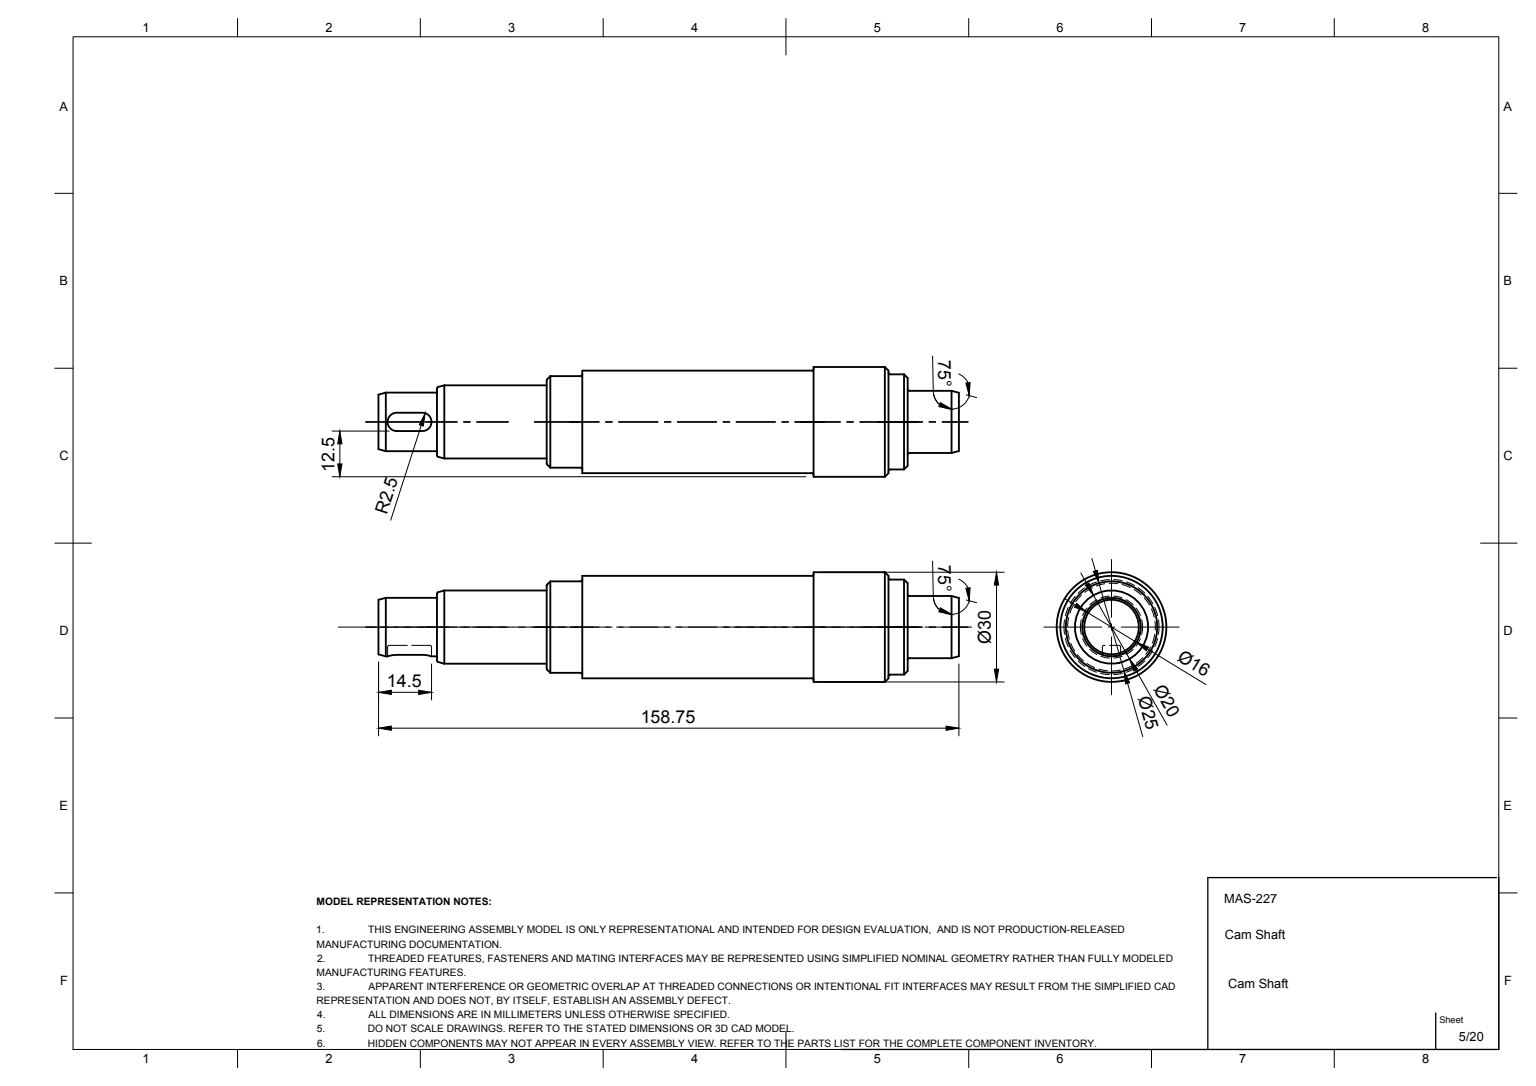
ISO-10303-21;
HEADER;
FILE_DESCRIPTION (('STEP AP214'),
    '1' );
FILE_NAME ( 'Cam Shaft.step', '2026-10-06T08:24:41', ( '' ), ( '' ), 'STEP AP214', 'Unspecified', '' );
FILE_SCHEMA (( 'AUTOMOTIVE_DESIGN' ));
ENDSEC;
DATA;
#1=ORIENTED_EDGE ( 'NONE', *, *, #7056, .T. ) ;
#8=CARTESIAN_POINT ( 'NONE',  ( 0.4441657790107835790, 0.2564944395515610931, 1.766732283464566899 ) ) ;
#9=CARTESIAN_POINT ( 'NONE',  ( -0.4441657790107816917, 0.2564944395515652564, 1.747047244094488194 ) ) ;
#12=ORIENTED_EDGE ( 'NONE', *, *, #1724, .F. ) ;
#14=CARTESIAN_POINT ( 'NONE',  ( 0.3392387706403788838, 0.1151913129404419922, -3.115157480314960647 ) ) ;
#21=CARTESIAN_POINT ( 'NONE',  ( 0.3324885138898234782, -0.04380447413659139394, 1.973425196850393970 ) ) ;
#25=VERTEX_POINT ( 'NONE', #21962 ) ;
#35=LINE ( 'NONE', #6897, #10289 ) ;
#46=CARTESIAN_POINT ( 'NONE',  ( -0.08600259748440698682, 0.2165354330708661457, -3.223068998490977499 ) ) ;
#47=ORIENTED_EDGE ( 'NONE', *, *, #24932, .T. ) ;
#49=DIRECTION ( 'NONE',  ( 0.000000000000000000, 0.000000000000000000, 1.000000000000000000 ) ) ;
#56=CARTESIAN_POINT ( 'NONE',  ( -0.5476281405333500718, 0.07214854559197644845, 0.9399606299212598381 ) ) ;
#59=ORIENTED_EDGE ( 'NONE', *, *, #13176, .F. ) ;
#74=CARTESIAN_POINT ( 'NONE',  ( 0.1480156394741928561, -0.5526079293736928522, 0.9399606299212598381 ) ) ;
#77=CARTESIAN_POINT ( 'NONE',  ( 0.04673558830902516809, 0.3552036222399216903, -3.115157480314960647 ) ) ;
#82=CARTESIAN_POINT ( 'NONE',  ( 0.4856708409191422549, -0.1649135259639211148, -1.550196850393700920 ) ) ;
#84=CARTESIAN_POINT ( 'NONE',  ( 0.5144793533649091311, -0.1379038425970198489, 1.747047244094488416 ) ) ;
#88=VERTEX_POINT ( 'NONE', #13082 ) ;
#90=CIRCLE ( 'NONE', #23529, 0.3937007874015748254 ) ;
#99=CARTESIAN_POINT ( 'NONE',  ( -0.3001918266901933974, 0.3912931228432126596, -1.550196850393700920 ) ) ;
#101=CARTESIAN_POINT ( 'NONE',  ( 0.1458850421962362143, -0.4296318976989931815, -1.934055118110236338 ) ) ;
#106=DIRECTION ( 'NONE',  ( -1.000000000000000000, 0.000000000000000000, -0.000000000000000000 ) ) ;
#113=CARTESIAN_POINT ( 'NONE',  ( -0.3350125228558759050, 0.2937477835494528011, -1.934055118110236560 ) ) ;
#118=CARTESIAN_POINT ( 'NONE',  ( -0.1839420097223181394, -0.5417097841048805762, 0.9399606299212598381 ) ) ;
#123=CARTESIAN_POINT ( 'NONE',  ( 0.3858827008519146728, -0.2227458012931471110, -1.934055118110236338 ) ) ;
#124=CARTESIAN_POINT ( 'NONE',  ( 0.3233561589689052385, -0.1867299569291582528, -3.115157480314960647 ) ) ;
#138=CARTESIAN_POINT ( 'NONE',  ( -0.4069448477556107946, -0.3121994997598286914, 1.766732283464566899 ) ) ;
#144=CARTESIAN_POINT ( 'NONE',  ( 0.3460635936745020680, -0.09269288654273737105, -3.115157480314960647 ) ) ;
#157=ORIENTED_EDGE ( 'NONE', *, *, #9364, .T. ) ;
#162=CARTESIAN_POINT ( 'NONE',  ( 0.09842519685039370636, 0.2165354330708661457, -3.456364829396325167 ) ) ;
#174=CARTESIAN_POINT ( 'NONE',  ( -0.07870736599817811097, 0.1968503937007873850, -3.212150913008701814 ) ) ;
#175=EDGE_LOOP ( 'NONE', ( #22367, #5338, #24383, #19393 ) ) ;
#188=CARTESIAN_POINT ( 'NONE',  ( -0.4382482975805212511, 0.3362148458989001609, 0.9399606299212598381 ) ) ;
#205=CARTESIAN_POINT ( 'NONE',  ( 0.07472527936312040042, -0.5671862884095228985, 0.9399606299212598381 ) ) ;
#215=CARTESIAN_POINT ( 'NONE',  ( 0.4954757973265890847, -0.2860025288253325582, 0.9399606299212601712 ) ) ;
#255=CARTESIAN_POINT ( 'NONE',  ( -0.03736310157557653361, -0.5708661417322835607, 0.9399606299212598381 ) ) ;
#258=CARTESIAN_POINT ( 'NONE',  ( 0.4303681241740789920, -0.1153557615287144622, -1.934055118110236338 ) ) ;
#259=CARTESIAN_POINT ( 'NONE',  ( -0.3233561589689049609, -0.1867299569291588357, -3.115157480314960647 ) ) ;
#271=CARTESIAN_POINT ( 'NONE',  ( 0.5118110236220472231, 0.03349795313260757468, 1.766732283464566899 ) ) ;
#277=CARTESIAN_POINT ( 'NONE',  ( 0.2362439534887500470, 0.2693339498142248156, -3.115157480314960647 ) ) ;
#283=CARTESIAN_POINT ( 'NONE',  ( 0.2521176338356670432, 0.2211428102655656758, 1.953740157480315043 ) ) ;
#285=VERTEX_POINT ( 'NONE', #25460 ) ;
#301=ORIENTED_EDGE ( 'NONE', *, *, #18506, .T. ) ;
#306=CARTESIAN_POINT ( 'NONE',  ( 0.07870736599818350943, 0.1968503937007873850, -3.212150913008773312 ) ) ;
#310=CARTESIAN_POINT ( 'NONE',  ( 0.3362554559023149814, -0.1141145734059788724, 1.953740157480315043 ) ) ;
#314=PLANE ( 'NONE',  #8850 ) ;
#317=CARTESIAN_POINT ( 'NONE',  ( 0.4783323773986625782, 0.2762247810518427271, 0.9399606299212598381 ) ) ;
#319=DIRECTION ( 'NONE',  ( 1.000000000000000000, 0.000000000000000000, 0.000000000000000000 ) ) ;
#324=AXIS2_PLACEMENT_3D ( 'NONE', #9492, #22508, #24756 ) ;
#330=ORIENTED_EDGE ( 'NONE', *, *, #18348, .T. ) ;
#332=CARTESIAN_POINT ( 'NONE',  ( -0.2529800193559212929, 0.5131133041954029084, 0.9399606299212598381 ) ) ;
#334=CARTESIAN_POINT ( 'NONE',  ( -0.5118110236220472231, 0.000000000000000000, 1.953740157480315043 ) ) ;
#349=LINE ( 'NONE', #4682, #16207 ) ;
#360=CARTESIAN_POINT ( 'NONE',  ( 0.4423390553432928751, 0.2180862235769577551, -1.550196850393700920 ) ) ;
#361=CARTESIAN_POINT ( 'NONE',  ( -0.4438564651657384008, -0.1188866373884874261, -1.928289503579162067 ) ) ;
#362=CARTESIAN_POINT ( 'NONE',  ( 0.09842519685039358146, 0.2991866959364303802, -3.548228346456693050 ) ) ;
#364=LINE ( 'NONE', #17572, #14246 ) ;
#381=CARTESIAN_POINT ( 'NONE',  ( 0.05811992390581651596, -0.4417530401346463909, -1.934055118110236560 ) ) ;
#382=CARTESIAN_POINT ( 'NONE',  ( -0.3349073414798507953, 0.1651192144506273274, -3.115157480314960647 ) ) ;
#396=CARTESIAN_POINT ( 'NONE',  ( -0.1649135259617042215, 0.4856708409200647392, 1.766732283464566899 ) ) ;
#399=ORIENTED_EDGE ( 'NONE', *, *, #24266, .F. ) ;
#400=CARTESIAN_POINT ( 'NONE',  ( 0.3349073414798194315, 0.1651192144506304638, -3.115157480314960647 ) ) ;
#405=CARTESIAN_POINT ( 'NONE',  ( -0.02190250779245987017, -0.3346456692913385988, 1.953740157480315043 ) ) ;
#408=ADVANCED_FACE ( 'NONE', ( #17123 ), #19236, .F. ) ;
#412=ORIENTED_EDGE ( 'NONE', *, *, #25098, .T. ) ;
#431=CARTESIAN_POINT ( 'NONE',  ( 0.2161875334157469797, -0.2816963220976381743, 1.953740157480315043 ) ) ;
#438=CARTESIAN_POINT ( 'NONE',  ( -0.1775991818008579581, 0.5230301363771275858, 0.9399606299212598381 ) ) ;
#453=CARTESIAN_POINT ( 'NONE',  ( -0.2860899518037610667, -0.4954156765914530247, 0.9399606299212598381 ) ) ;
#477=CARTESIAN_POINT ( 'NONE',  ( -0.03220957031754079214, -0.4921259842519685179, -1.550196850393700920 ) ) ;
#481=CARTESIAN_POINT ( 'NONE',  ( 0.1648264847746512829, -0.4857053587577857545, -1.550196850393700920 ) ) ;
#502=CARTESIAN_POINT ( 'NONE',  ( 0.2712680014829234043, -0.3534612032201311371, -1.934055118110236338 ) ) ;
#517=CARTESIAN_POINT ( 'NONE',  ( -0.4600326175560697783, 0.2268096725222554233, 1.747047244094488194 ) ) ;
#518=ADVANCED_FACE ( 'NONE', ( #21226 ), #21837, .T. ) ;
#521=CARTESIAN_POINT ( 'NONE',  ( 0.1867299569291587802, -0.3233561589689049609, -3.115157480314960647 ) ) ;
#522=EDGE_CURVE ( 'NONE', #3990, #21275, #23634, .T. ) ;
#526=CARTESIAN_POINT ( 'NONE',  ( -0.3175540113612211890, 0.1078280746903930443, 1.953740157480315043 ) ) ;
#535=CARTESIAN_POINT ( 'NONE',  ( -0.04840761057735708250, 0.1968503937007874127, -3.611172162805734942 ) ) ;
#538=CARTESIAN_POINT ( 'NONE',  ( -0.07874015748031502893, 0.1968503937007874127, -3.272637795275590733 ) ) ;
#542=CARTESIAN_POINT ( 'NONE',  ( -0.3074993854542729665, -0.1775730735577446262, 1.953740157480315043 ) ) ;
#549=ADVANCED_FACE ( 'NONE', ( #4668 ), #4259, .T. ) ;
#556=EDGE_CURVE ( 'NONE', #4928, #5829, #1626, .T. ) ;
#561=CARTESIAN_POINT ( 'NONE',  ( 0.4152525734085952824, 0.3642352168757231889, 0.9399606299212598381 ) ) ;
#574=CARTESIAN_POINT ( 'NONE',  ( -0.2904160862623708650, 0.1677079028045392328, 1.953740157480315043 ) ) ;
#579=CARTESIAN_POINT ( 'NONE',  ( -0.5131133041954075713, -0.2529800193559338384, 0.9399606299212598381 ) ) ;
#581=CARTESIAN_POINT ( 'NONE',  ( -0.2577577458591217563, -0.4472135058506044314, 1.766732283464566899 ) ) ;
#601=CARTESIAN_POINT ( 'NONE',  ( -0.06048688188729484105, 0.2165354330708661734, -3.626935712834467029 ) ) ;
#605=CARTESIAN_POINT ( 'NONE',  ( 0.1275996891957845991, -0.4763861460130774939, -1.550196850393700920 ) ) ;
#606=CARTESIAN_POINT ( 'NONE',  ( 0.03001016326913514068, -0.4585215200179055817, -1.928289503579156516 ) ) ;
#636=CARTESIAN_POINT ( 'NONE',  ( -0.2227458012934312725, -0.3858827008515844370, -1.934055118110236560 ) ) ;
#637=CARTESIAN_POINT ( 'NONE',  ( -0.3384212623783161011, 0.1668516812751324463, -3.100567304031758287 ) ) ;
#641=CARTESIAN_POINT ( 'NONE',  ( -0.2478439864030018425, -0.4300129863948121134, -1.569881889763780070 ) ) ;
#649=CARTESIAN_POINT ( 'NONE',  ( -0.1327036767659477978, -0.4954415918530775120, 1.747047244094488194 ) ) ;
#651=CARTESIAN_POINT ( 'NONE',  ( 0.2962590301041581609, -0.2272836761397895311, -3.115157480314960647 ) ) ;
#654=VECTOR ( 'NONE', #25570, 39.37007874015748143 ) ;
#656=CARTESIAN_POINT ( 'NONE',  ( 0.1677079028045289355, -0.2904160862623609840, 1.953740157480315043 ) ) ;
#663=ADVANCED_FACE ( 'NONE', ( #5225 ), #20348, .T. ) ;
#668=FACE_OUTER_BOUND ( 'NONE', #21089, .T. ) ;
#674=CARTESIAN_POINT ( 'NONE',  ( 0.04956879728060029772, 0.2165354330708661457, -3.186635197996628310 ) ) ;
#683=CARTESIAN_POINT ( 'NONE',  ( 0.1649135259617122706, 0.4856708409200614640, 1.766732283464566899 ) ) ;
#691=CARTESIAN_POINT ( 'NONE',  ( -0.3667122560601319692, 0.09855118063547732565, -3.100567304031763616 ) ) ;
#696=CARTESIAN_POINT ( 'NONE',  ( 0.5131133041954023533, 0.2529800193559384458, 0.9399606299212598381 ) ) ;
#704=CARTESIAN_POINT ( 'NONE',  ( 0.09842519685039355370, 0.2165354330708661457, -3.548228346456693050 ) ) ;
#711=CARTESIAN_POINT ( 'NONE',  ( 0.2521176338356516666, -0.2211428102655709216, 1.953740157480315043 ) ) ;
#713=SHAPE_REPRESENTATION ( 'Cam Shaft', ( #11588 ), #2999 ) ;
#718=CARTESIAN_POINT ( 'NONE',  ( 0.4984899526255158753, -0.1339654526248288402, 1.766732283464567788 ) ) ;
#724=VERTEX_POINT ( 'NONE', #23035 ) ;
#738=CARTESIAN_POINT ( 'NONE',  ( 0.3765118517642104257, -2.263258471485603576E-17, -3.100567304031763172 ) ) ;
#741=CARTESIAN_POINT ( 'NONE',  ( 0.3007905576423847704, 0.1482986320106501610, 1.973425196850393970 ) ) ;
#742=CARTESIAN_POINT ( 'NONE',  ( -0.5118110236220182463, 0.03349795313034509281, -1.550196850393700920 ) ) ;
#743=CARTESIAN_POINT ( 'NONE',  ( -0.2297883689023225706, -0.3979194638820617858, -1.928289503579150077 ) ) ;
#750=CARTESIAN_POINT ( 'NONE',  ( 0.1188866373884869265, 0.4438564651657460614, -1.928289503579154740 ) ) ;
#752=CARTESIAN_POINT ( 'NONE',  ( -0.03220957031754000111, 0.4921259842519685179, -1.569881889763779625 ) ) ;
#756=CARTESIAN_POINT ( 'NONE',  ( 0.4724409448465559103, 5.785732908924860203E-17, 1.953740157480315043 ) ) ;
#757=DIRECTION ( 'NONE',  ( 0.000000000000000000, 0.000000000000000000, 1.000000000000000000 ) ) ;
#763=CARTESIAN_POINT ( 'NONE',  ( -0.1775236553381950300, 0.3075341118176279642, 1.953740157480315487 ) ) ;
#766=CARTESIAN_POINT ( 'NONE',  ( 0.4498374011142918794, -0.05926487674658236643, -1.934055118110236338 ) ) ;
#770=FACE_OUTER_BOUND ( 'NONE', #2926, .T. ) ;
#775=EDGE_CURVE ( 'NONE', #24094, #88, #25559, .T. ) ;
#778=CARTESIAN_POINT ( 'NONE',  ( -0.4446020952038909901, -0.02920026389085020324, -1.934055118110237448 ) ) ;
#779=CARTESIAN_POINT ( 'NONE',  ( -0.1668516812751421607, 0.3384212623783116602, -3.100567304031759175 ) ) ;
#784=CARTESIAN_POINT ( 'NONE',  ( -0.3858397471888794783, 0.2228126397720086582, -1.934055118110236338 ) ) ;
#792=CARTESIAN_POINT ( 'NONE',  ( 0.2564944395515950104, 0.4441657790108120563, 1.747047244094488194 ) ) ;
#794=CARTESIAN_POINT ( 'NONE',  ( 0.3702005978258383068, -0.04877294052296102245, -3.115157480314960647 ) ) ;
#800=ORIENTED_EDGE ( 'NONE', *, *, #13640, .T. ) ;
#802=CARTESIAN_POINT ( 'NONE',  ( 0.1152775731717068236, 0.4303822302054135518, -1.934055118110236338 ) ) ;
#804=VERTEX_POINT ( 'NONE', #4097 ) ;
#816=CARTESIAN_POINT ( 'NONE',  ( -0.04380501567505455662, -0.3346456692913385433, 1.973425196850393970 ) ) ;
#817=CARTESIAN_POINT ( 'NONE',  ( 0.3184841198566381593, 0.1570220809524529026, 1.953740157480315043 ) ) ;
#822=CARTESIAN_POINT ( 'NONE',  ( -0.5280699926563170443, -0.06957181182498474448, 1.747047244094488194 ) ) ;
#823=CARTESIAN_POINT ( 'NONE',  ( 0.5118110236220472231, 0.000000000000000000, 1.766732283464566899 ) ) ;
#836=CARTESIAN_POINT ( 'NONE',  ( -0.4921259842519685179, -0.03220957031763953954, -1.569881889763779625 ) ) ;
#840=CARTESIAN_POINT ( 'NONE',  ( -0.4382482975804890546, -0.3362148458988509225, 0.9399606299212598381 ) ) ;
#856=CARTESIAN_POINT ( 'NONE',  ( -0.04380447413658625222, -0.3324885138898230341, 1.953740157480315043 ) ) ;
#871=EDGE_CURVE ( 'NONE', #12664, #8508, #14728, .T. ) ;
#878=CARTESIAN_POINT ( 'NONE',  ( 0.09842519685039355370, 0.2165354330708661457, -3.548228346456692162 ) ) ;
#885=CARTESIAN_POINT ( 'NONE',  ( -2.685748425196850164E-17, 0.000000000000000000, -3.115157480314960647 ) ) ;
#886=CARTESIAN_POINT ( 'NONE',  ( -0.3239425792934405024, 0.08676778863011171128, 1.973425196850393970 ) ) ;
#888=CARTESIAN_POINT ( 'NONE',  ( 0.03220957031753916844, -0.4921259842519685179, -1.550196850393700920 ) ) ;
#891=CARTESIAN_POINT ( 'NONE',  ( 0.5230301363771324707, 0.1775991818008611500, 0.9202755905511811330 ) ) ;
#896=CARTESIAN_POINT ( 'NONE',  ( 0.2031943647053748025, 0.4121342552748526455, -1.928289503579147190 ) ) ;
#914=CARTESIAN_POINT ( 'NONE',  ( 0.08582765042225336261, 0.3030860912054640921, -3.222734230592224858 ) ) ;
#920=CARTESIAN_POINT ( 'NONE',  ( 0.3572819248074489140, -0.1213180142433802344, -3.100567304031756066 ) ) ;
#925=CARTESIAN_POINT ( 'NONE',  ( -0.2228126397719833174, 0.3858397471888795893, -1.934055118110236338 ) ) ;
#931=FACE_OUTER_BOUND ( 'NONE', #26813, .T. ) ;
#933=CARTESIAN_POINT ( 'NONE',  ( 0.06699507805369034341, 0.5085118447801111330, 1.747047244094488194 ) ) ;
#937=CARTESIAN_POINT ( 'NONE',  ( -0.02464264302293797324, 0.3765118517642104257, -3.100567304031763172 ) ) ;
#948=CARTESIAN_POINT ( 'NONE',  ( 0.07667729696052867638, 0.1968503937007874405, -3.568863587253130021 ) ) ;
#950=B_SPLINE_CURVE_WITH_KNOTS ( 'NONE', 2,
 ( #2095, #10422, #14562 ),
 .UNSPECIFIED., .F., .F.,
 ( 3, 3 ),
 ( 0.000000000000000000, 1.000000000000000000 ),
 .UNSPECIFIED. ) ;
#952=CARTESIAN_POINT ( 'NONE',  ( -0.3392387706403475200, 0.1151913129404399938, -3.115157480314960647 ) ) ;
#961=CARTESIAN_POINT ( 'NONE',  ( -0.3543307086614173596, -0.02319089060378156514, 1.953740157480315043 ) ) ;
#964=FACE_OUTER_BOUND ( 'NONE', #13122, .T. ) ;
#966=CARTESIAN_POINT ( 'NONE',  ( -0.4004221243553304777, 0.3512268162760389667, 1.747047244094488194 ) ) ;
#974=CARTESIAN_POINT ( 'NONE',  ( -0.04632170870458265227, -0.3520570504767543962, 1.953740157480315043 ) ) ;
#975=DIRECTION ( 'NONE',  ( 1.000000000000000000, 0.000000000000000000, 0.000000000000000000 ) ) ;
#977=ORIENTED_EDGE ( 'NONE', *, *, #2179, .T. ) ;
#979=CARTESIAN_POINT ( 'NONE',  ( 0.1585706980422492418, -0.4669911931914798586, -1.569881889763779625 ) ) ;
#981=CARTESIAN_POINT ( 'NONE',  ( -0.5671862884095143498, 0.07472527936311554320, 0.9399606299212598381 ) ) ;
#990=DIRECTION ( 'NONE',  ( 0.000000000000000000, 0.000000000000000000, -1.000000000000000000 ) ) ;
#995=CARTESIAN_POINT ( 'NONE',  ( 0.3346456692913385988, 0.000000000000000000, 1.953740157480315043 ) ) ;
#1002=CARTESIAN_POINT ( 'NONE',  ( 0.000000000000000000, 0.000000000000000000, 2.504921259842519898 ) ) ;
#1007=ORIENTED_EDGE ( 'NONE', *, *, #24560, .F. ) ;
#1010=CARTESIAN_POINT ( 'NONE',  ( 0.02061007003135870153, 0.1968503937007873850, -3.624919108234744058 ) ) ;
#1019=ADVANCED_FACE ( 'NONE', ( #18015 ), #22311, .T. ) ;
#1024=CARTESIAN_POINT ( 'NONE',  ( -0.04380447413658894451, -0.3324885138898239778, 1.973425196850393970 ) ) ;
#1025=CARTESIAN_POINT ( 'NONE',  ( -0.4921259842519975503, -0.03220957031763956036, -1.550196850393700920 ) ) ;
#1029=CARTESIAN_POINT ( 'NONE',  ( -0.4152525734086685016, 0.3642352168757148623, 0.9399606299212598381 ) ) ;
#1031=DIRECTION ( 'NONE',  ( 0.000000000000000000, 0.000000000000000000, 1.000000000000000000 ) ) ;
#1037=CARTESIAN_POINT ( 'NONE',  ( -0.2180862235769353841, 0.4423390553432505756, -1.569881889763779625 ) ) ;
#1043=ORIENTED_EDGE ( 'NONE', *, *, #4237, .T. ) ;
#1047=VERTEX_POINT ( 'NONE', #15795 ) ;
#1052=CARTESIAN_POINT ( 'NONE',  ( -0.3929158813954686247, -0.2268989272875759633, -1.934055118110236338 ) ) ;
#1056=CARTESIAN_POINT ( 'NONE',  ( -0.04991389860279011464, 0.3112157083527658519, -3.186815069313337023 ) ) ;
#1064=VERTEX_POINT ( 'NONE', #15664 ) ;
#1065=CARTESIAN_POINT ( 'NONE',  ( -0.3702005978258584573, -0.04877294052295926691, -3.115157480314960647 ) ) ;
#1070=CARTESIAN_POINT ( 'NONE',  ( 0.3535065162672724748, -0.2712027394948692827, -1.934055118110236338 ) ) ;
#1073=CARTESIAN_POINT ( 'NONE',  ( 0.09842519685039366473, 0.1968503937007873850, -3.548228346456693050 ) ) ;
#1075=CARTESIAN_POINT ( 'NONE',  ( 0.3121994997598600552, -0.4069448477555897004, 1.766732283464566899 ) ) ;
#1081=CARTESIAN_POINT ( 'NONE',  ( 0.09762295995069811272, -0.3644697409450263215, -3.100567304031765836 ) ) ;
#1088=DIRECTION ( 'NONE',  ( 0.000000000000000000, -1.000000000000000000, 0.000000000000000000 ) ) ;
#1090=CARTESIAN_POINT ( 'NONE',  ( 0.4417361510193959506, -0.05819755867303935681, -1.934055118110236338 ) ) ;
#1097=CARTESIAN_POINT ( 'NONE',  ( -0.06881554280526554213, 0.1968503937007874127, -3.233007928613536919 ) ) ;
#1099=CARTESIAN_POINT ( 'NONE',  ( -0.3346456692913385988, 2.134256245050205639E-17, 1.973425196850393970 ) ) ;
#1105=CARTESIAN_POINT ( 'NONE',  ( 0.2341512108694265570, -0.2669480828848097009, 1.953740157480315043 ) ) ;
#1112=CARTESIAN_POINT ( 'NONE',  ( 0.4441657790107724213, -0.2564944395515492137, 1.747047244094488194 ) ) ;
#1113=CARTESIAN_POINT ( 'NONE',  ( 0.3855916753051445989, -0.3382184156732112590, 1.766732283464566899 ) ) ;
#1115=ORIENTED_EDGE ( 'NONE', *, *, #12278, .F. ) ;
#1117=EDGE_LOOP ( 'NONE', ( #20134, #3108, #1, #19528 ) ) ;
#1123=CARTESIAN_POINT ( 'NONE',  ( -0.3001918266902340870, -0.3912931228432089403, -1.569881889763779625 ) ) ;
#1136=CARTESIAN_POINT ( 'NONE',  ( -0.1677079028045393438, -0.2904160862623708095, 1.953740157480315043 ) ) ;
#1138=ORIENTED_EDGE ( 'NONE', *, *, #4001, .T. ) ;
#1145=CARTESIAN_POINT ( 'NONE',  ( -0.3135473077061334268, 0.000000000000000000, 2.504921259842519898 ) ) ;
#1152=DIRECTION ( 'NONE',  ( -0.2588190448135640476, 0.000000000000000000, -0.9659258263664939337 ) ) ;
#1153=CARTESIAN_POINT ( 'NONE',  ( 0.03965503742771005202, 0.1968503937007873850, -3.617030424444199088 ) ) ;
#1156=CARTESIAN_POINT ( 'NONE',  ( -0.07874015748031502893, 0.1968503937007874127, -3.272637795275590733 ) ) ;
#1168=EDGE_LOOP ( 'NONE', ( #2501, #9246, #14088, #7714 ) ) ;
#1169=CARTESIAN_POINT ( 'NONE',  ( -0.3007905576423873240, 0.1482986320106437494, 1.973425196850393970 ) ) ;
#1172=CARTESIAN_POINT ( 'NONE',  ( 0.5335524835332355886, 0.1429116519061127411, 0.9202755905511811330 ) ) ;
#1177=CARTESIAN_POINT ( 'NONE',  ( 0.03220957031753989008, 0.4921259842519685179, -1.569881889763779625 ) ) ;
#1181=LENGTH_MEASURE_WITH_UNIT ( LENGTH_MEASURE( 0.02539999999999999897 ), #9208 ) ;
#1187=VECTOR ( 'NONE', #1591, 39.37007874015748143 ) ;
#1192=CARTESIAN_POINT ( 'NONE',  ( 0.3184597017669858476, 0.1570773243922341800, 1.953740157480315043 ) ) ;
#1194=CARTESIAN_POINT ( 'NONE',  ( -0.4382752542995838052, -0.1173917140416377847, -1.934055118110236338 ) ) ;
#1196=CARTESIAN_POINT ( 'NONE',  ( 0.07874794988990475864, 0.3051012802738558571, -3.212194302032695070 ) ) ;
#1204=CARTESIAN_POINT ( 'NONE',  ( -0.3384212623783144913, -0.1668516812751341671, -3.100567304031760951 ) ) ;
#1207=CARTESIAN_POINT ( 'NONE',  ( -0.2761764805255799704, 0.3599896729929456529, -1.934055118110236338 ) ) ;
#1212=CARTESIAN_POINT ( 'NONE',  ( 0.06957181182498554939, 0.5280699926562867352, 1.747047244094488194 ) ) ;
#1217=CARTESIAN_POINT ( 'NONE',  ( -0.1213180142433868958, -0.3572819248074448062, -3.100567304031760951 ) ) ;
#1230=CARTESIAN_POINT ( 'NONE',  ( 0.3535065162672720307, 0.2712027394948698378, -1.934055118110236338 ) ) ;
#1235=CARTESIAN_POINT ( 'NONE',  ( 0.2180698645301765992, 0.2842490391651533721, -3.115157480314960647 ) ) ;
#1246=CARTESIAN_POINT ( 'NONE',  ( 0.4225965726692672009, 0.3242071728275124354, 1.747047244094488194 ) ) ;
#1248=CARTESIAN_POINT ( 'NONE',  ( -0.1327036767659643679, -0.4954415918530851726, 1.766732283464566899 ) ) ;
#1251=CARTESIAN_POINT ( 'NONE',  ( -0.3392387706403475200, 0.1151913129404399938, -3.115157480314960647 ) ) ;
#1260=CARTESIAN_POINT ( 'NONE',  ( 0.4921259842519685179, -0.03220957031753991784, -1.569881889763779625 ) ) ;
#1264=ORIENTED_EDGE ( 'NONE', *, *, #20212, .F. ) ;
#1267=CARTESIAN_POINT ( 'NONE',  ( 0.3574975638436101444, 4.268512490100411279E-17, -3.115157480314960647 ) ) ;
#1269=CARTESIAN_POINT ( 'NONE',  ( -0.3937007874015748254, 4.821444091131312140E-17, -1.934055118110236338 ) ) ;
#1303=CARTESIAN_POINT ( 'NONE',  ( 0.4600326175570071952, 0.2268096725200290653, -1.550196850393700920 ) ) ;
#1304=CARTESIAN_POINT ( 'NONE',  ( 0.5368353335967095408, 0.1442704874421229244, 0.9202755905511813550 ) ) ;
#1305=CARTESIAN_POINT ( 'NONE',  ( -0.1429116519061075785, -0.5335524835332366989, 0.9202755905511811330 ) ) ;
#1311=CARTESIAN_POINT ( 'NONE',  ( -0.4921259842519685179, 0.000000000000000000, -1.569881889763779625 ) ) ;
#1317=CARTESIAN_POINT ( 'NONE',  ( 0.3511566718594107961, 0.4004902621173285215, 1.747047244094488194 ) ) ;
#1326=CARTESIAN_POINT ( 'NONE',  ( -0.3184623230426369966, 0.1570784101599410065, 1.953740157480315487 ) ) ;
#1335=CARTESIAN_POINT ( 'NONE',  ( -0.4446020952038907681, 0.000000000000000000, -1.934055118110236338 ) ) ;
#1338=CARTESIAN_POINT ( 'NONE',  ( 0.1275996891957757451, -0.4763861460130329184, -1.569881889763779625 ) ) ;
#1341=CARTESIAN_POINT ( 'NONE',  ( 0.4303822302053771365, 0.1152775731717053109, -1.934055118110236338 ) ) ;
#1356=CARTESIAN_POINT ( 'NONE',  ( 0.1432577568504609655, -0.4218945342797526532, -1.934055118110236338 ) ) ;
#1358=ORIENTED_EDGE ( 'NONE', *, *, #13176, .T. ) ;
#1359=CARTESIAN_POINT ( 'NONE',  ( -0.4585215200179055817, 2.807634559150536355E-17, -1.928289503579156516 ) ) ;
#1362=CARTESIAN_POINT ( 'NONE',  ( 0.3574975638436101444, 0.02339816079119100625, -3.115157480314960647 ) ) ;
#1364=CARTESIAN_POINT ( 'NONE',  ( 0.08759279594700324079, 0.3259357382551449911, 1.973425196850393526 ) ) ;
#1373=CARTESIAN_POINT ( 'NONE',  ( -0.3771675965698903510, 0.4301570366553708613, 0.9399606299212600602 ) ) ;
#1376=DIRECTION ( 'NONE',  ( 1.000000000000000000, 0.000000000000000000, 0.000000000000000000 ) ) ;
#1379=CARTESIAN_POINT ( 'NONE',  ( 0.5280699926562892887, 0.06957181182498746452, 1.747047244094488194 ) ) ;
#1380=CARTESIAN_POINT ( 'NONE',  ( -0.3121994997598258603, -0.4069448477556126265, 1.766732283464566899 ) ) ;
#1390=CARTESIAN_POINT ( 'NONE',  ( -0.4921259842519685179, 0.000000000000000000, -1.550196850393700920 ) ) ;
#1419=ORIENTED_EDGE ( 'NONE', *, *, #20548, .F. ) ;
#1425=DIRECTION ( 'NONE',  ( 1.000000000000000000, 0.000000000000000000, 0.000000000000000000 ) ) ;
#1433=CARTESIAN_POINT ( 'NONE',  ( -0.02190250779245987017, -0.3346456692913387099, 1.973425196850393970 ) ) ;
#1434=CARTESIAN_POINT ( 'NONE',  ( -0.06699507805605005306, -0.5085118447796763697, -1.550196850393700920 ) ) ;
#1438=CARTESIAN_POINT ( 'NONE',  ( -0.4783323773986942751, -0.2762247810518927427, 0.9399606299212598381 ) ) ;
#1442=B_SPLINE_SURFACE_WITH_KNOTS ( 'NONE', 2, 3, ( 
 ( #11031, #8366, #4400, #1858 ),
 ( #8629, #19657, #16981, #21497 ),
 ( #2136, #25871, #2266, #15151 ) ),
 .UNSPECIFIED., .F., .F., .F.,
 ( 3, 3 ),
 ( 4, 4 ),
 ( 0.000000000000000000, 1.000000000000000000 ),
 ( -0.006999999999999992339, 0.000000000000000000 ),
 .UNSPECIFIED. ) ;
#1445=CARTESIAN_POINT ( 'NONE',  ( 0.3667122560601320802, -0.09855118063547688156, -3.100567304031763172 ) ) ;
#1447=CARTESIAN_POINT ( 'NONE',  ( 0.09586345222253732368, 0.2165354330708661457, -3.246875207736362956 ) ) ;
#1453=FACE_OUTER_BOUND ( 'NONE', #16309, .T. ) ;
#1473=CARTESIAN_POINT ( 'NONE',  ( -0.1152775731717027019, -0.4303822302053992854, -1.934055118110236338 ) ) ;
#1481=CARTESIAN_POINT ( 'NONE',  ( 0.4954415918530775120, -0.1327036767659478256, 1.747047244094488194 ) ) ;
#1487=CARTESIAN_POINT ( 'NONE',  ( -0.1668516812751398570, -0.3384212623783108276, -3.100567304031765392 ) ) ;
#1489=DIRECTION ( 'NONE',  ( -0.000000000000000000, -0.000000000000000000, 1.000000000000000000 ) ) ;
#1490=CARTESIAN_POINT ( 'NONE',  ( 0.09187177619659094019, 0.3429980251342388264, 1.953740157480315043 ) ) ;
#1495=CARTESIAN_POINT ( 'NONE',  ( 0.07472527936311225416, 0.5671862884095085766, 0.9399606299212598381 ) ) ;
#1497=ORIENTED_EDGE ( 'NONE', *, *, #21755, .T. ) ;
#1503=CARTESIAN_POINT ( 'NONE',  ( -0.3551931031211721379, -0.04679574315772278004, -3.115157480314960647 ) ) ;
#1509=DIRECTION ( 'NONE',  ( -1.000000000000000000, 0.000000000000000000, -0.000000000000000000 ) ) ;
#1512=CARTESIAN_POINT ( 'NONE',  ( -0.5708661417322834497, 0.000000000000000000, 0.9399606299212598381 ) ) ;
#1520=CARTESIAN_POINT ( 'NONE',  ( -0.5118110236220472231, 0.03349795313264340019, 1.766732283464566899 ) ) ;
#1529=CARTESIAN_POINT ( 'NONE',  ( 0.1078280746903962500, -0.3175540113612315696, 1.973425196850393970 ) ) ;
#1532=CARTESIAN_POINT ( 'NONE',  ( 0.1585706980422384171, -0.4669911931914537129, -1.550196850393700920 ) ) ;
#1563=CARTESIAN_POINT ( 'NONE',  ( -0.5335524835332333682, 0.1429116519061236767, 0.9202755905511811330 ) ) ;
#1572=FACE_OUTER_BOUND ( 'NONE', #24833, .T. ) ;
#1578=CARTESIAN_POINT ( 'NONE',  ( 0.2041304421298449356, -0.2660793235464211093, 1.973425196850393970 ) ) ;
#1580=CARTESIAN_POINT ( 'NONE',  ( 0.5335524835332418059, -0.1429116519061131296, 0.9399606299212598381 ) ) ;
#1586=CARTESIAN_POINT ( 'NONE',  ( 0.4225410690757945842, 0.3242876858385722039, 1.747047244094488416 ) ) ;
#1587=ORIENTED_EDGE ( 'NONE', *, *, #21256, .T. ) ;
#1591=DIRECTION ( 'NONE',  ( 0.000000000000000000, 0.000000000000000000, 1.000000000000000000 ) ) ;
#1601=CARTESIAN_POINT ( 'NONE',  ( 0.3346456692913385988, 2.049113738730807321E-17, 1.973425196850393970 ) ) ;
#1609=CARTESIAN_POINT ( 'NONE',  ( 0.3102804211134971291, -0.1791085948260274507, -3.115157480314961091 ) ) ;
#1611=CARTESIAN_POINT ( 'NONE',  ( -0.03220957031754079214, -0.4921259842519684624, -1.569881889763779625 ) ) ;
#1613=CARTESIAN_POINT ( 'NONE',  ( 0.4296318976989619842, -0.1458850421962461508, -1.934055118110236338 ) ) ;
#1620=CARTESIAN_POINT ( 'NONE',  ( 0.3242071728275122688, 0.4225965726692672564, 1.747047244094488194 ) ) ;
#1623=ADVANCED_FACE ( 'NONE', ( #931 ), #12970, .T. ) ;
#1626=B_SPLINE_CURVE_WITH_KNOTS ( 'NONE', 2,
 ( #5078, #9046, #11444 ),
 .UNSPECIFIED., .F., .F.,
 ( 3, 3 ),
 ( 0.000000000000000000, 1.000000000000000000 ),
 .UNSPECIFIED. ) ;
#1627=CARTESIAN_POINT ( 'NONE',  ( 0.4446006764000813294, 0.02917857698668059607, -1.934055118110236560 ) ) ;
#1629=CARTESIAN_POINT ( 'NONE',  ( -0.2817310484609168997, -0.2161381151963037983, 1.953740157480315043 ) ) ;
#1633=CARTESIAN_POINT ( 'NONE',  ( -0.3010840436257778419, -0.2313841235333768398, -3.100567304031763172 ) ) ;
#1634=CARTESIAN_POINT ( 'NONE',  ( -0.5708661417322835607, 0.000000000000000000, 0.9399606299212598381 ) ) ;
#1642=CARTESIAN_POINT ( 'NONE',  ( -0.04679574315772200288, 0.3551931031211610357, -3.115157480314960647 ) ) ;
#1643=CARTESIAN_POINT ( 'NONE',  ( -0.5511811023622047445, 3.375010863791918375E-17, 0.9202755905511811330 ) ) ;
#1651=CARTESIAN_POINT ( 'NONE',  ( 0.5417490723637030658, 0.1838434515542585190, 0.9399606299212597271 ) ) ;
#1659=CARTESIAN_POINT ( 'NONE',  ( 0.2564944395515950104, 0.4441657790108120563, 1.747047244094488194 ) ) ;
#1665=CARTESIAN_POINT ( 'NONE',  ( 0.2817828961649161412, -0.3666644560843326239, -1.928289503579156516 ) ) ;
#1668=CARTESIAN_POINT ( 'NONE',  ( -0.3175540113612297932, -0.1078280746904006077, 1.973425196850393970 ) ) ;
#1671=CARTESIAN_POINT ( 'NONE',  ( -0.03220957031754079214, -0.4921259842519685179, -1.550196850393700920 ) ) ;
#1677=DIRECTION ( 'NONE',  ( 0.000000000000000000, 0.000000000000000000, -1.000000000000000000 ) ) ;
#1694=EDGE_LOOP ( 'NONE', ( #4784, #800, #15232, #24470 ) ) ;
#1700=CARTESIAN_POINT ( 'NONE',  ( -0.5085118447796470598, -0.06699507805605113553, -1.550196850393700920 ) ) ;
#1702=CARTESIAN_POINT ( 'NONE',  ( -0.5511811023622047445, 0.000000000000000000, 0.9202755905511811330 ) ) ;
#1703=CARTESIAN_POINT ( 'NONE',  ( 0.4857053587577992437, 0.1648264847746080952, -1.550196850393700920 ) ) ;
#1715=CARTESIAN_POINT ( 'NONE',  ( -0.1677079028045287967, 0.2904160862623510475, 1.953740157480315043 ) ) ;
#1716=CARTESIAN_POINT ( 'NONE',  ( 0.3855916753034687172, 0.3382184156749162285, -1.550196850393700920 ) ) ;
#1719=CARTESIAN_POINT ( 'NONE',  ( -0.1429116519060979196, -0.5335524835332288163, 0.9399606299212598381 ) ) ;
#1724=EDGE_CURVE ( 'NONE', #3938, #18589, #364, .T. ) ;
#1731=CARTESIAN_POINT ( 'NONE',  ( 0.4856708409191126674, 0.1649135259639225026, -1.550196850393700920 ) ) ;
#1742=CARTESIAN_POINT ( 'NONE',  ( 0.3543307086614173596, 0.000000000000000000, 1.953740157480315043 ) ) ;
#1749=CARTESIAN_POINT ( 'NONE',  ( -0.3392634445560575029, -0.1151354519024665318, -3.115157480314960647 ) ) ;
#1751=CARTESIAN_POINT ( 'NONE',  ( -0.3599896729929590866, -0.2761764805255594313, -1.934055118110236338 ) ) ;
#1757=CARTESIAN_POINT ( 'NONE',  ( -0.5144970376935736889, 0.1378076643338841389, 1.747047244094488194 ) ) ;
#1766=ORIENTED_EDGE ( 'NONE', *, *, #4888, .T. ) ;
#1768=CARTESIAN_POINT ( 'NONE',  ( 0.3520466617656906050, 0.04638120790933070170, 1.953740157480315043 ) ) ;
#1779=CARTESIAN_POINT ( 'NONE',  ( -0.2693339498142344746, -0.2362439534887506021, -3.115157480314960647 ) ) ;
#1785=CARTESIAN_POINT ( 'NONE',  ( -0.09586345242798390009, 0.2165354330708661734, -3.246875208232354648 ) ) ;
#1789=AXIS2_PLACEMENT_3D ( 'NONE', #2792, #20182, #20047 ) ;
#1803=CARTESIAN_POINT ( 'NONE',  ( 0.3213305936751376102, 0.1584254766472200371, -3.115157480314960647 ) ) ;
#1805=CARTESIAN_POINT ( 'NONE',  ( -0.1200170377978880404, -0.4465874321618643061, -1.928289503579156294 ) ) ;
#1806=VERTEX_POINT ( 'NONE', #5550 ) ;
#1808=CARTESIAN_POINT ( 'NONE',  ( -0.1078280746904014958, -0.3175540113612295157, 1.973425196850393970 ) ) ;
#1812=CARTESIAN_POINT ( 'NONE',  ( -0.3252100150720461658, 0.3707612262532960501, -1.550196850393700920 ) ) ;
#1834=CARTESIAN_POINT ( 'NONE',  ( -2.685748425196850164E-17, 0.000000000000000000, -3.115157480314960647 ) ) ;
#1839=LENGTH_MEASURE_WITH_UNIT ( LENGTH_MEASURE( 0.02539999999999999897 ), #25850 ) ;
#1840=ORIENTED_EDGE ( 'NONE', *, *, #26753, .F. ) ;
#1854=VECTOR ( 'NONE', #10953, 39.37007874015748854 ) ;
#1856=ORIENTED_EDGE ( 'NONE', *, *, #775, .F. ) ;
#1858=CARTESIAN_POINT ( 'NONE',  ( -0.07874015748031495954, 0.1968503937007873850, -3.272637795275590733 ) ) ;
#1860=CARTESIAN_POINT ( 'NONE',  ( 0.1482986320106470801, -0.3007905576423859917, 1.973425196850393970 ) ) ;
#1861=DIRECTION ( 'NONE',  ( -0.000000000000000000, -0.000000000000000000, 1.000000000000000000 ) ) ;
#1865=CARTESIAN_POINT ( 'NONE',  ( 0.4783323773986630778, -0.2762247810518744240, 0.9399606299212598381 ) ) ;
#1868=CARTESIAN_POINT ( 'NONE',  ( 0.2693781226336498524, 0.2362017869178958951, -3.115157480314961980 ) ) ;
#1872=CARTESIAN_POINT ( 'NONE',  ( -0.2268096725200260955, 0.4600326175569864340, -1.550196850393700920 ) ) ;
#1875=CARTESIAN_POINT ( 'NONE',  ( -0.4225410690760224575, -0.3242876858381196770, 1.747047244094488194 ) ) ;
#1879=AXIS2_PLACEMENT_3D ( 'NONE', #19649, #10746, #6792 ) ;
#1892=CARTESIAN_POINT ( 'NONE',  ( -0.4585215200179055817, 0.03001016326912889221, -1.928289503579156516 ) ) ;
#1907=ORIENTED_EDGE ( 'NONE', *, *, #6203, .F. ) ;
#1909=CARTESIAN_POINT ( 'NONE',  ( -0.3520466617656973218, 0.04638120790932954290, 1.953740157480315043 ) ) ;
#1914=CARTESIAN_POINT ( 'NONE',  ( 0.5671862884095085766, -0.07472527936312026164, 0.9399606299212598381 ) ) ;
#1919=ADVANCED_FACE ( 'NONE', ( #21749 ), #8460, .T. ) ;
#1921=CARTESIAN_POINT ( 'NONE',  ( -0.02438677169350859236, -0.3726024258163779246, -3.115157480314960647 ) ) ;
#1927=CARTESIAN_POINT ( 'NONE',  ( 0.4793172621399190980, -0.1288129352161812291, -1.569881889763779625 ) ) ;
#1929=CARTESIAN_POINT ( 'NONE',  ( -0.4382482975805018222, 0.3362148458988871713, 0.9202755905511811330 ) ) ;
#1932=CARTESIAN_POINT ( 'NONE',  ( 0.5525886237723619532, 0.1481199686341792554, 0.9399606299212597271 ) ) ;
#1937=CARTESIAN_POINT ( 'NONE',  ( -0.2564944395515745823, 0.4441657790107744752, 1.766732283464566899 ) ) ;
#1941=CARTESIAN_POINT ( 'NONE',  ( -0.3102476824511484210, -0.1791601451668926870, -3.115157480314960647 ) ) ;
#1943=FACE_OUTER_BOUND ( 'NONE', #20847, .T. ) ;
#1945=CARTESIAN_POINT ( 'NONE',  ( -0.08676778863011193332, -0.3239425792934405024, 1.973425196850393970 ) ) ;
#1960=CARTESIAN_POINT ( 'NONE',  ( -0.01308409974552196542, 0.3147525462474320412, -3.645993128380378590 ) ) ;
#1972=CARTESIAN_POINT ( 'NONE',  ( 0.06048688226685065145, 0.2165354330708661457, -3.193930429277373140 ) ) ;
#1981=CARTESIAN_POINT ( 'NONE',  ( 0.1775991818008376133, 0.5230301363771421297, 0.9202755905511811330 ) ) ;
#1985=ORIENTED_EDGE ( 'NONE', *, *, #5181, .T. ) ;
#1996=CARTESIAN_POINT ( 'NONE',  ( 0.3346456692913385988, 0.000000000000000000, 1.973425196850393970 ) ) ;
#2000=CARTESIAN_POINT ( 'NONE',  ( -0.2442565704126459791, -0.4954197419817803483, 0.9399606299212598381 ) ) ;
#2002=CARTESIAN_POINT ( 'NONE',  ( -6.092417322834646079E-17, 0.5905905511811023745, -3.272637795275590733 ) ) ;
#2009=CARTESIAN_POINT ( 'NONE',  ( 0.1327036767636011194, 0.4954415918535620689, -1.550196850393700920 ) ) ;
#2010=CARTESIAN_POINT ( 'NONE',  ( -0.2530774914999985303, -0.5130713940403577311, 0.9399606299212601712 ) ) ;
#2013=CARTESIAN_POINT ( 'NONE',  ( 0.4225434286521223548, -0.3242892624567478843, 1.747047244094488194 ) ) ;
#2017=EDGE_LOOP ( 'NONE', ( #1840, #6428 ) ) ;
#2019=DIRECTION ( 'NONE',  ( 0.000000000000000000, 0.000000000000000000, 1.000000000000000000 ) ) ;
#2028=CARTESIAN_POINT ( 'NONE',  ( 0.2180862235769585322, 0.4423390553432415273, -1.550196850393700920 ) ) ;
#2032=CARTESIAN_POINT ( 'NONE',  ( 0.2991932138496286586, -0.3411003281197161341, -1.934055118110236338 ) ) ;
#2033=CARTESIAN_POINT ( 'NONE',  ( 0.3346456692913385988, 2.049113738730807321E-17, 1.973425196850393970 ) ) ;
#2034=CARTESIAN_POINT ( 'NONE',  ( -0.1432577568504646015, 0.4218945342797250642, -1.934055118110236338 ) ) ;
#2040=CARTESIAN_POINT ( 'NONE',  ( 0.5280699926562971713, -0.06957181182499251604, 1.747047244094488194 ) ) ;
#2045=CARTESIAN_POINT ( 'NONE',  ( -0.3858827008516800827, 0.2227458012932893583, -1.934055118110236560 ) ) ;
#2048=CARTESIAN_POINT ( 'NONE',  ( 0.3184841198566246701, -0.1570220809524502659, 1.953740157480315043 ) ) ;
#2053=CARTESIAN_POINT ( 'NONE',  ( 0.07472527936312040042, -0.5671862884095228985, 0.9399606299212598381 ) ) ;
#2054=DIRECTION ( 'NONE',  ( -1.000000000000000000, 0.000000000000000000, 0.000000000000000000 ) ) ;
#2059=CARTESIAN_POINT ( 'NONE',  ( 0.3606853515406420185, -0.09660931395005377398, -3.115157480314960647 ) ) ;
#2065=CARTESIAN_POINT ( 'NONE',  ( 0.2478439864030018147, -0.4300129863948118913, -1.569881889763779625 ) ) ;
#2069=CARTESIAN_POINT ( 'NONE',  ( 0.5118110236220473341, 6.402768735150616610E-17, -1.550196850393700920 ) ) ;
#2075=CARTESIAN_POINT ( 'NONE',  ( 0.5144970376935932288, -0.1378076643338853879, 1.747047244094488194 ) ) ;
#2077=CARTESIAN_POINT ( 'NONE',  ( -0.3121994997598258603, -0.4069448477556126265, 1.766732283464566899 ) ) ;
#2081=EDGE_LOOP ( 'NONE', ( #12866, #14072, #25975, #11994 ) ) ;
#2083=CARTESIAN_POINT ( 'NONE',  ( 0.3460635936744816399, 0.09269288654273792616, -3.115157480314960647 ) ) ;
#2084=ORIENTED_EDGE ( 'NONE', *, *, #7458, .F. ) ;
#2086=CIRCLE ( 'NONE', #19695, 0.5905511811023621549 ) ;
#2090=CARTESIAN_POINT ( 'NONE',  ( -0.2211428102655751127, -0.2521176338356575508, 1.973425196850393970 ) ) ;
#2093=CARTESIAN_POINT ( 'NONE',  ( -0.3707612262532960501, 0.3252100150720461658, -1.550196850393700920 ) ) ;
#2095=CARTESIAN_POINT ( 'NONE',  ( -0.5511811023622047445, 3.375010863791918375E-17, 0.9202755905511811330 ) ) ;
#2116=CARTESIAN_POINT ( 'NONE',  ( -0.06296589279854497567, 0.1968503937007873850, -3.224248289462050998 ) ) ;
#2126=CARTESIAN_POINT ( 'NONE',  ( 0.4783323773986672967, -0.2762247810518773106, 0.9202755905511811330 ) ) ;
#2136=CARTESIAN_POINT ( 'NONE',  ( -0.09842519685039370636, 0.2165354330708661457, -3.548228346456693050 ) ) ;
#2143=CARTESIAN_POINT ( 'NONE',  ( 0.3482225189666513510, -0.4539000224940975547, 0.9399606299212598381 ) ) ;
#2148=CARTESIAN_POINT ( 'NONE',  ( -0.3213085410496429040, 0.1584824234588512737, -3.115157480314961091 ) ) ;
#2152=CARTESIAN_POINT ( 'NONE',  ( 0.5085118447796558305, 0.06699507805605002531, -1.550196850393700920 ) ) ;
#2172=CARTESIAN_POINT ( 'NONE',  ( -0.3707612262533165337, -0.3252100150720257932, -1.569881889763779625 ) ) ;
#2173=CARTESIAN_POINT ( 'NONE',  ( -0.4585215200179055817, 0.000000000000000000, -1.928289503579156516 ) ) ;
#2179=EDGE_CURVE ( 'NONE', #14125, #1064, #15162, .T. ) ;
#2185=CARTESIAN_POINT ( 'NONE',  ( -0.09842519685039370636, 0.2165354330708661457, -3.548228346456693050 ) ) ;
#2187=CARTESIAN_POINT ( 'NONE',  ( 0.3995913070738940642, 0.1970988029425181920, -1.934055118110236338 ) ) ;
#2197=CARTESIAN_POINT ( 'NONE',  ( 0.3606853515406215904, 0.09660931395005435685, -3.115157480314960647 ) ) ;
#2207=CARTESIAN_POINT ( 'NONE',  ( 0.4092783051644228731, 0.3145317858139328182, 1.766732283464566899 ) ) ;
#2209=CARTESIAN_POINT ( 'NONE',  ( -0.3382184156732166436, 0.3855916753051391033, 1.766732283464566899 ) ) ;
#2212=EDGE_LOOP ( 'NONE', ( #12586, #23625, #17128, #15554 ) ) ;
#2214=CARTESIAN_POINT ( 'NONE',  ( -0.04679574315772456333, -0.3551931031211519874, -3.115157480314960647 ) ) ;
#2236=ADVANCED_FACE ( 'NONE', ( #27103 ), #25129, .T. ) ;
#2237=VECTOR ( 'NONE', #11282, 39.37007874015748143 ) ;
#2239=CARTESIAN_POINT ( 'NONE',  ( -0.06002032661671147240, 0.4585215200179056372, -1.928289503579156516 ) ) ;
#2243=CARTESIAN_POINT ( 'NONE',  ( -0.06048688226689048764, 0.1968503937007873850, -3.193930429277412220 ) ) ;
#2246=AXIS2_PLACEMENT_3D ( 'NONE', #2393, #11022, #319 ) ;
#2251=CARTESIAN_POINT ( 'NONE',  ( 0.4446020952038907681, 5.549066237130534971E-17, -1.934055118110236338 ) ) ;
#2255=CARTESIAN_POINT ( 'NONE',  ( 0.4382482975805169212, -0.3362148458988646338, 0.9202755905511811330 ) ) ;
#2266=CARTESIAN_POINT ( 'NONE',  ( -0.09842519685039370636, 0.2165354330708661457, -3.364501312335955063 ) ) ;
#2274=CARTESIAN_POINT ( 'NONE',  ( -0.3772436174784328244, 0.4300830224589641260, 0.9399606299212598381 ) ) ;
#2282=CARTESIAN_POINT ( 'NONE',  ( -0.3912931228432058872, -0.3001918266902326993, -1.550196850393700920 ) ) ;
#2283=CARTESIAN_POINT ( 'NONE',  ( -0.4538422614037148084, -0.3483115186076898295, 0.9399606299212598381 ) ) ;
#2297=CARTESIAN_POINT ( 'NONE',  ( 0.06441834428466734763, 0.4889536969035060965, -1.550196850393700920 ) ) ;
#2298=EDGE_CURVE ( 'NONE', #19599, #5829, #18049, .T. ) ;
#2299=CARTESIAN_POINT ( 'NONE',  ( 0.3454440660767517657, -0.3030032861724969440, -1.928289503579156516 ) ) ;
#2300=CARTESIAN_POINT ( 'NONE',  ( 0.4438564651657277427, 0.1188866373884867045, -1.928289503579172726 ) ) ;
#2307=CARTESIAN_POINT ( 'NONE',  ( 0.4225965726693019509, -0.3242071728275352505, 1.747047244094488194 ) ) ;
#2313=ORIENTED_EDGE ( 'NONE', *, *, #26134, .F. ) ;
#2321=CARTESIAN_POINT ( 'NONE',  ( 0.3482225189666513510, -0.4539000224940975547, 0.9399606299212598381 ) ) ;
#2322=CARTESIAN_POINT ( 'NONE',  ( -0.4724409448465559103, 0.000000000000000000, 1.953740157480315043 ) ) ;
#2326=CARTESIAN_POINT ( 'NONE',  ( -0.3350145293472930885, -0.2937497900410970253, -1.934055118110236338 ) ) ;
#2327=CARTESIAN_POINT ( 'NONE',  ( -0.2807137536170348779, -0.2462256503456018430, -3.115157480314960647 ) ) ;
#2333=COLOUR_RGB ( '', 0.72549020, 0.75294118, 0.79215686) ;
#2338=DIRECTION ( 'NONE',  ( -0.000000000000000000, -0.000000000000000000, -1.000000000000000000 ) ) ;
#2339=CARTESIAN_POINT ( 'NONE',  ( 0.4600326175560556230, 0.2268096725222457644, 1.766732283464566899 ) ) ;
#2340=CARTESIAN_POINT ( 'NONE',  ( -0.5085118447801415531, -0.06699507805368200286, 1.747047244094488194 ) ) ;
#2344=AXIS2_PLACEMENT_3D ( 'NONE', #4791, #990, #13410 ) ;
#2346=CARTESIAN_POINT ( 'NONE',  ( -0.3606853515406169275, 0.09660931395005029065, -3.115157480314960647 ) ) ;
#2351=CARTESIAN_POINT ( 'NONE',  ( 0.3175540113612289050, 0.1078280746903826914, 1.953740157480315043 ) ) ;
#2357=EDGE_LOOP ( 'NONE', ( #8662, #5777 ) ) ;
#2361=CARTESIAN_POINT ( 'NONE',  ( -0.2228126397720058549, -0.3858397471888898589, -1.934055118110236338 ) ) ;
#2371=DIRECTION ( 'NONE',  ( 0.000000000000000000, 0.000000000000000000, -1.000000000000000000 ) ) ;
#2376=CARTESIAN_POINT ( 'NONE',  ( -0.09586345222253926657, 0.2165354330708661457, -3.246875207736367841 ) ) ;
#2391=ORIENTED_EDGE ( 'NONE', *, *, #8273, .T. ) ;
#2392=CARTESIAN_POINT ( 'NONE',  ( -0.4954197419817281123, 0.2442565704126535286, 0.9399606299212598381 ) ) ;
#2393=CARTESIAN_POINT ( 'NONE',  ( 0.000000000000000000, 0.000000000000000000, 0.9399606299212598381 ) ) ;
#2411=DIRECTION ( 'NONE',  ( 1.000000000000000000, 0.000000000000000000, 0.000000000000000000 ) ) ;
#2428=EDGE_LOOP ( 'NONE', ( #26101, #7798 ) ) ;
#2440=CARTESIAN_POINT ( 'NONE',  ( -0.2466292688015002954, -0.4270824798167766612, -1.569881889763779625 ) ) ;
#2441=CARTESIAN_POINT ( 'NONE',  ( 0.4121342552748372690, -0.2031943647053953139, -1.928289503579153630 ) ) ;
#2448=CARTESIAN_POINT ( 'NONE',  ( -0.1712563538833084820, -0.5043504886477717664, 1.747047244094488194 ) ) ;
#2452=AXIS2_PLACEMENT_3D ( 'NONE', #16676, #18775, #6357 ) ;
#2468=CARTESIAN_POINT ( 'NONE',  ( -0.3702005978258633423, 0.04877294052296513721, -3.115157480314960647 ) ) ;
#2476=CIRCLE ( 'NONE', #20065, 0.5118110236220472231 ) ;
#2478=ORIENTED_EDGE ( 'NONE', *, *, #11220, .T. ) ;
#2483=PRODUCT_CONTEXT ( 'NONE', #11249, 'mechanical' ) ;
#2484=CARTESIAN_POINT ( 'NONE',  ( 0.2564944395515608710, 0.4441657790107836346, 1.766732283464566899 ) ) ;
#2486=AXIS2_PLACEMENT_3D ( 'NONE', #8171, #18884, #16494 ) ;
#2490=CARTESIAN_POINT ( 'NONE',  ( 0.3606853515406420185, -0.09660931395005377398, -3.115157480314960647 ) ) ;
#2495=CARTESIAN_POINT ( 'NONE',  ( 0.3324885138898166503, 0.04380447413659039474, 1.953740157480315043 ) ) ;
#2497=ORIENTED_EDGE ( 'NONE', *, *, #3094, .F. ) ;
#2499=CARTESIAN_POINT ( 'NONE',  ( 0.4527559054764770385, 5.549066237130534971E-17, -1.934055118110236338 ) ) ;
#2501=ORIENTED_EDGE ( 'NONE', *, *, #16475, .F. ) ;
#2530=CARTESIAN_POINT ( 'NONE',  ( 0.4954197419817712444, -0.2442565704126122561, 0.9202755905511811330 ) ) ;
#2544=CARTESIAN_POINT ( 'NONE',  ( 0.1839420097223035677, -0.5417097841048799101, 0.9399606299212598381 ) ) ;
#2569=CARTESIAN_POINT ( 'NONE',  ( -0.4270824798167728864, 0.2466292688015120915, -1.550196850393700920 ) ) ;
#2573=CARTESIAN_POINT ( 'NONE',  ( -0.3362148458988422073, 0.4382482975805319092, 0.9202755905511811330 ) ) ;
#2577=CARTESIAN_POINT ( 'NONE',  ( 0.03001016326913580681, 0.4585215200179055817, -1.928289503579156516 ) ) ;
#2592=CARTESIAN_POINT ( 'NONE',  ( -0.4527559054764770385, 0.02963280468031418563, -1.934055118110236338 ) ) ;
#2599=CARTESIAN_POINT ( 'NONE',  ( 0.2993674444872233553, -0.2296683860596848981, -3.100567304031763172 ) ) ;
#2603=B_SPLINE_CURVE_WITH_KNOTS ( 'NONE', 2,
 ( #11290, #26521, #13679 ),
 .UNSPECIFIED., .F., .F.,
 ( 3, 3 ),
 ( 0.000000000000000000, 1.000000000000000000 ),
 .UNSPECIFIED. ) ;
#2614=CARTESIAN_POINT ( 'NONE',  ( -0.4984899526255159308, 0.1339654526248284516, 1.766732283464566899 ) ) ;
#2615=CARTESIAN_POINT ( 'NONE',  ( -0.5085118447801413311, 0.06699507805369032953, 1.747047244094488194 ) ) ;
#2621=CARTESIAN_POINT ( 'NONE',  ( -0.3726024258163779246, -0.02438677169354843896, -3.115157480314960647 ) ) ;
#2626=CARTESIAN_POINT ( 'NONE',  ( 0.2041304421298504035, -0.2660793235464293249, 1.953740157480315043 ) ) ;
#2638=CARTESIAN_POINT ( 'NONE',  ( 0.06881018027183069541, 0.1968503937007874127, -3.233009657539146708 ) ) ;
#2645=CARTESIAN_POINT ( 'NONE',  ( -0.02319089060378104472, -0.3543307086614173596, 1.953740157480315043 ) ) ;
#2660=CARTESIAN_POINT ( 'NONE',  ( 0.4527559054764771496, 0.000000000000000000, -1.934055118110236338 ) ) ;
#2663=CARTESIAN_POINT ( 'NONE',  ( -0.07214854559198104200, 0.5476281405333119912, 0.9399606299212598381 ) ) ;
#2665=ORIENTED_EDGE ( 'NONE', *, *, #21755, .F. ) ;
#2678=CARTESIAN_POINT ( 'NONE',  ( -0.2529800193559321730, -0.5131133041954082374, 0.9399606299212598381 ) ) ;
#2698=CARTESIAN_POINT ( 'NONE',  ( 0.02564049093248907743, 0.3139791838537054902, -3.643473821106772981 ) ) ;
#2700=CARTESIAN_POINT ( 'NONE',  ( 0.06699507805605696420, 0.5085118447796661556, -1.550196850393700920 ) ) ;
#2701=CARTESIAN_POINT ( 'NONE',  ( 0.3645739570812638330, -0.2796934465393868807, -1.928289503579156072 ) ) ;
#2703=CARTESIAN_POINT ( 'NONE',  ( 0.1188866373884749916, -0.4438564651657395665, -1.928289503579163178 ) ) ;
#2705=CARTESIAN_POINT ( 'NONE',  ( -0.03607471876262472593, 0.5511811023622047445, 0.9202755905511811330 ) ) ;
#2709=CARTESIAN_POINT ( 'NONE',  ( 0.1477428134820460426, 0.4351030398461616100, -1.928289503579165842 ) ) ;
#2712=DIRECTION ( 'NONE',  ( 0.7071067818211401734, 8.659560570126452765E-17, -0.7071067805519547500 ) ) ;
#2733=CARTESIAN_POINT ( 'NONE',  ( 0.1886891683788904650, 0.3267488823401754061, -3.100567304031762284 ) ) ;
#2745=CARTESIAN_POINT ( 'NONE',  ( -0.2268096725222598919, -0.4600326175560532915, 1.747047244094488194 ) ) ;
#2748=CARTESIAN_POINT ( 'NONE',  ( 0.2462256503455911016, 0.2807137536170354331, -3.115157480314960647 ) ) ;
#2755=CARTESIAN_POINT ( 'NONE',  ( -0.3346456692913385988, -0.02190250779246036283, 1.953740157480315043 ) ) ;
#2763=CARTESIAN_POINT ( 'NONE',  ( 0.06294381634853177254, 0.1968503937007874127, -3.596635957034346021 ) ) ;
#2767=CARTESIAN_POINT ( 'NONE',  ( 0.000000000000000000, 0.000000000000000000, 1.747047244094488194 ) ) ;
#2770=CARTESIAN_POINT ( 'NONE',  ( -0.1570220809524502104, -0.3184841198566448206, 1.953740157480315043 ) ) ;
#2777=CARTESIAN_POINT ( 'NONE',  ( 0.3121994997598427912, 0.4069448477556012467, 1.766732283464566899 ) ) ;
#2790=CARTESIAN_POINT ( 'NONE',  ( 0.03607471876262387245, -0.5511811023622048555, 0.9399606299212598381 ) ) ;
#2791=VERTEX_POINT ( 'NONE', #12929 ) ;
#2792=CARTESIAN_POINT ( 'NONE',  ( 0.000000000000000000, 0.000000000000000000, 1.747047244094488194 ) ) ;
#2801=CARTESIAN_POINT ( 'NONE',  ( -0.3239425792934415571, -0.08676778863010886633, 1.953740157480315043 ) ) ;
#2806=CARTESIAN_POINT ( 'NONE',  ( -0.1339654526248285349, -0.4984899526255157087, 1.766732283464566677 ) ) ;
#2809=CARTESIAN_POINT ( 'NONE',  ( 0.3574961452116665606, 0.02345921195965534889, -3.115157480314960647 ) ) ;
#2822=ORIENTED_EDGE ( 'NONE', *, *, #16341, .F. ) ;
#2830=CARTESIAN_POINT ( 'NONE',  ( 0.09842519685039370636, 0.2165354330708661457, -3.272637795275590733 ) ) ;
#2832=CARTESIAN_POINT ( 'NONE',  ( -0.2521176338356572177, -0.2211428102655754180, 1.973425196850393970 ) ) ;
#2834=CARTESIAN_POINT ( 'NONE',  ( -0.4423390553432768879, -0.2180862235769457091, -1.550196850393700920 ) ) ;
#2836=CARTESIAN_POINT ( 'NONE',  ( 0.06001958459476169905, -0.4555658499976140696, -1.928289503579150077 ) ) ;
#2838=CARTESIAN_POINT ( 'NONE',  ( 0.1429116519061275903, 0.5335524835332325910, 0.9202755905511811330 ) ) ;
#2843=CARTESIAN_POINT ( 'NONE',  ( -0.4763861460130329739, 0.1275996891957754675, -1.569881889763779625 ) ) ;
#2846=DIRECTION ( 'NONE',  ( 0.2588190448135643806, 0.000000000000000000, 0.9659258263664939337 ) ) ;
#2849=CLOSED_SHELL ( 'NONE', ( #19233, #19425, #7267, #3992, #27872, #3766, #16838, #549, #518, #21735, #15372, #5394, #24391, #24830, #4706, #6449, #19552, #6236, #23916, #4940, #4260, #15149, #16729, #21569, #22767, #11069, #663, #19835, #22092, #3616, #10112, #7090, #6231, #6239, #23934, #408, #27024, #12980, #20774, #11670, #18690, #18113, #24949, #13433, #22326, #1019, #1623, #1919, #10233, #25707, #18777, #12122, #10296, #2236, #13299, #4620 ) ) ;
#2856=CARTESIAN_POINT ( 'NONE',  ( 0.4069519308877023178, -0.2006393256663573099, -1.934055118110236338 ) ) ;
#2866=CARTESIAN_POINT ( 'NONE',  ( -0.3740848232703756771, 0.04928467685643712209, -3.100567304031759175 ) ) ;
#2871=EDGE_CURVE ( 'NONE', #20420, #3990, #24254, .T. ) ;
#2872=CARTESIAN_POINT ( 'NONE',  ( -0.4300129863948120579, -0.2478439864030019535, -1.569881889763780070 ) ) ;
#2879=ORIENTED_EDGE ( 'NONE', *, *, #24423, .T. ) ;
#2882=CARTESIAN_POINT ( 'NONE',  ( 0.03349795313264332386, 0.5118110236220472231, 1.747047244094488194 ) ) ;
#2883=CARTESIAN_POINT ( 'NONE',  ( -0.06699507805371239522, -0.5085118447801502128, 1.747047244094488194 ) ) ;
#2886=CARTESIAN_POINT ( 'NONE',  ( -0.04877294052296160531, 0.3702005978258477437, -3.115157480314960647 ) ) ;
#2897=CARTESIAN_POINT ( 'NONE',  ( 0.4303822302053771365, 0.1152775731717053109, -1.934055118110236338 ) ) ;
#2908=CARTESIAN_POINT ( 'NONE',  ( -0.04956879728060034629, 0.2165354330708661734, -3.186635197996628310 ) ) ;
#2910=CARTESIAN_POINT ( 'NONE',  ( -0.3259357382551450466, -0.08759279594700321303, 1.973425196850394192 ) ) ;
#2914=DIRECTION ( 'NONE',  ( 0.7071067818211439482, 8.659560570126498371E-17, -0.7071067805519510863 ) ) ;
#2919=CARTESIAN_POINT ( 'NONE',  ( -0.5144970376935736889, 0.1378076643338841389, 1.747047244094488194 ) ) ;
#2926=EDGE_LOOP ( 'NONE', ( #26692, #19413, #18428, #2665 ) ) ;
#2929=CARTESIAN_POINT ( 'NONE',  ( -0.3252100150720461658, 0.3707612262532960501, -1.569881889763779625 ) ) ;
#2932=CARTESIAN_POINT ( 'NONE',  ( -0.3642352168757849173, -0.4152525734086955356, 0.9399606299212598381 ) ) ;
#2960=LINE ( 'NONE', #20072, #13900 ) ;
#2971=CARTESIAN_POINT ( 'NONE',  ( -0.2521176338356575508, 0.2211428102655751127, 1.973425196850393970 ) ) ;
#2972=CARTESIAN_POINT ( 'NONE',  ( 0.3912931228432192099, -0.3001918266902123267, -1.550196850393700920 ) ) ;
#2976=CARTESIAN_POINT ( 'NONE',  ( 0.3642352168757554964, -0.4152525734086275899, 0.9202755905511811330 ) ) ;
#2981=CARTESIAN_POINT ( 'NONE',  ( -0.3001918266902143251, 0.3912931228432222075, -1.569881889763779625 ) ) ;
#2991=CARTESIAN_POINT ( 'NONE',  ( 0.1775220790477149424, 0.3075317527317797395, 1.953740157480315043 ) ) ;
#2994=CARTESIAN_POINT ( 'NONE',  ( -0.2761764805255463306, -0.3599896729929341621, -1.934055118110236338 ) ) ;
#2995=CARTESIAN_POINT ( 'NONE',  ( -0.3726024258163779246, 0.02438677169354841121, -3.115157480314960647 ) ) ;
#2999=( GEOMETRIC_REPRESENTATION_CONTEXT ( 3 ) GLOBAL_UNCERTAINTY_ASSIGNED_CONTEXT ( ( #24565 ) ) GLOBAL_UNIT_ASSIGNED_CONTEXT ( ( #17236, #18926, #25289 ) ) REPRESENTATION_CONTEXT ( 'NONE', 'WORKASPACE' ) ) ;
#3003=CARTESIAN_POINT ( 'NONE',  ( 0.2993674444872273521, 0.2296683860596781812, -3.100567304031764060 ) ) ;
#3007=CARTESIAN_POINT ( 'NONE',  ( -0.4921259842519686845, -0.06441914069860964209, -1.569881889763780070 ) ) ;
#3016=CARTESIAN_POINT ( 'NONE',  ( 0.1327036767659575123, -0.4954415918530866714, 1.766732283464566899 ) ) ;
#3020=CIRCLE ( 'NONE', #18825, 0.4921259842519685179 ) ;
#3021=CARTESIAN_POINT ( 'NONE',  ( 0.3233561589689049054, 0.1867299569291689110, -3.115157480314960647 ) ) ;
#3033=CARTESIAN_POINT ( 'NONE',  ( 0.1152775731716972618, -0.4303822302053990634, -1.934055118110236338 ) ) ;
#3040=CARTESIAN_POINT ( 'NONE',  ( 0.3346456692913385988, 2.049113738730807321E-17, 1.973425196850393970 ) ) ;
#3046=CARTESIAN_POINT ( 'NONE',  ( 0.1141709026133643362, 0.3362336590883639453, 1.953740157480315043 ) ) ;
#3052=CARTESIAN_POINT ( 'NONE',  ( -0.5144970376935739109, -0.1378076643338908835, 1.747047244094488194 ) ) ;
#3053=CARTESIAN_POINT ( 'NONE',  ( -0.1327036767659680594, 0.4954415918530845619, 1.766732283464566899 ) ) ;
#3062=EDGE_CURVE ( 'NONE', #17898, #14958, #14383, .T. ) ;
#3064=CARTESIAN_POINT ( 'NONE',  ( 0.4270824798167637826, -0.2466292688015195855, -1.569881889763779625 ) ) ;
#3067=CARTESIAN_POINT ( 'NONE',  ( -0.5476281405333571772, -0.07214854559198842499, 0.9399606299212598381 ) ) ;
#3084=CARTESIAN_POINT ( 'NONE',  ( 0.3239425792934414461, -0.08676778863010961573, 1.953740157480315043 ) ) ;
#3094=EDGE_CURVE ( 'NONE', #10030, #4351, #19419, .T. ) ;
#3104=CARTESIAN_POINT ( 'NONE',  ( -0.06880207798751750148, 0.1968503937007873850, -3.587883383884437727 ) ) ;
#3108=ORIENTED_EDGE ( 'NONE', *, *, #14866, .F. ) ;
#3118=CARTESIAN_POINT ( 'NONE',  ( -0.1078280746904014958, -0.3175540113612295157, 1.973425196850393970 ) ) ;
#3119=CARTESIAN_POINT ( 'NONE',  ( 0.4889536969034951053, 0.06441834428467130280, -1.550196850393700920 ) ) ;
#3123=CARTESIAN_POINT ( 'NONE',  ( 0.07214854559197284023, -0.5476281405333195407, 0.9202755905511811330 ) ) ;
#3125=CONICAL_SURFACE ( 'NONE', #24330, 0.2938622683360631593, 0.2617993874999998138 ) ;
#3127=CARTESIAN_POINT ( 'NONE',  ( 0.09855118063547671503, -0.3667122560601320247, -3.100567304031763172 ) ) ;
#3154=CARTESIAN_POINT ( 'NONE',  ( 0.04928467685643810742, 0.3740848232703744003, -3.100567304031763172 ) ) ;
#3159=CARTESIAN_POINT ( 'NONE',  ( 0.3858397471888842523, 0.2228126397719887297, -1.934055118110236338 ) ) ;
#3163=CARTESIAN_POINT ( 'NONE',  ( 0.3382184156732089830, -0.3855916753051465973, 1.766732283464566899 ) ) ;
#3166=CARTESIAN_POINT ( 'NONE',  ( 0.2488091035917030791, 0.2836590635674509642, -3.100567304031764948 ) ) ;
#3175=CARTESIAN_POINT ( 'NONE',  ( -6.092417322834646079E-17, 0.1968503937007874127, -3.272637795275590733 ) ) ;
#3177=CARTESIAN_POINT ( 'NONE',  ( -0.1152775731717027019, -0.4303822302053992854, -1.934055118110236338 ) ) ;
#3180=CARTESIAN_POINT ( 'NONE',  ( 0.5118110236220472231, 6.267877318470705905E-17, 1.953740157480315043 ) ) ;
#3183=CARTESIAN_POINT ( 'NONE',  ( -0.3213305936751693626, 0.1584254766472210918, -3.115157480314960647 ) ) ;
#3184=CARTESIAN_POINT ( 'NONE',  ( -0.07874015748031502893, 0.1968503937007873850, -3.262343610818749795 ) ) ;
#3190=CARTESIAN_POINT ( 'NONE',  ( 0.09187177619658809524, -0.3429980251342298336, 1.953740157480315043 ) ) ;
#3196=CARTESIAN_POINT ( 'NONE',  ( 0.2663596103035608120, 0.4612490782035171266, 1.747047244094488194 ) ) ;
#3198=CARTESIAN_POINT ( 'NONE',  ( 0.3382184156732163660, 0.3855916753051394363, 1.747047244094488194 ) ) ;
#3202=EDGE_CURVE ( 'NONE', #24677, #19192, #17913, .T. ) ;
#3207=EDGE_LOOP ( 'NONE', ( #5503, #12814, #14113, #25331 ) ) ;
#3208=ORIENTED_EDGE ( 'NONE', *, *, #21724, .F. ) ;
#3210=CARTESIAN_POINT ( 'NONE',  ( -0.1585706980422252055, -0.4669911931914896841, -1.569881889763779625 ) ) ;
#3236=CARTESIAN_POINT ( 'NONE',  ( -0.06296589279854382382, 0.1968503937007873850, -3.596617852270226567 ) ) ;
#3251=CARTESIAN_POINT ( 'NONE',  ( 0.1585706980422384171, -0.4669911931914537129, -1.550196850393700920 ) ) ;
#3255=CARTESIAN_POINT ( 'NONE',  ( 0.1429116519061227053, -0.5335524835332334792, 0.9202755905511811330 ) ) ;
#3267=CARTESIAN_POINT ( 'NONE',  ( -0.1379032889621888969, 0.5144765700550301135, 1.747047244094488194 ) ) ;
#3268=FILL_AREA_STYLE ('',( #26447 ) ) ;
#3271=EDGE_LOOP ( 'NONE', ( #24542, #16400, #27074, #1358 ) ) ;
#3290=CARTESIAN_POINT ( 'NONE',  ( -0.3644697409450258219, -0.09762295995070061072, -3.100567304031765836 ) ) ;
#3294=CARTESIAN_POINT ( 'NONE',  ( -0.3996230174612653285, -0.1970259548082108347, -1.934055118110236338 ) ) ;
#3302=CARTESIAN_POINT ( 'NONE',  ( 0.3512268162760394108, 0.4004221243553300891, 1.747047244094488194 ) ) ;
#3304=CARTESIAN_POINT ( 'NONE',  ( 0.2488091035916884242, -0.2836590635674675620, -3.100567304031759175 ) ) ;
#3314=CARTESIAN_POINT ( 'NONE',  ( 0.4446020952038907681, 0.02909913904662021419, -1.934055118110236338 ) ) ;
#3320=CARTESIAN_POINT ( 'NONE',  ( 0.1584254766472226184, 0.3213305936751399972, -3.115157480314960647 ) ) ;
#3321=CARTESIAN_POINT ( 'NONE',  ( 0.2775852647713620280, -0.4816145447621893450, 0.9202755905511812440 ) ) ;
#3323=CARTESIAN_POINT ( 'NONE',  ( -2.685748425196850164E-17, 0.000000000000000000, -3.745078740157480546 ) ) ;
#3326=CARTESIAN_POINT ( 'NONE',  ( 0.2924088307484721261, -0.1685339107540413384, 1.973425196850394192 ) ) ;
#3337=CARTESIAN_POINT ( 'NONE',  ( 0.06957181182498554939, 0.5280699926562867352, 1.747047244094488194 ) ) ;
#3338=CARTESIAN_POINT ( 'NONE',  ( -0.5085118447801436625, -0.06699507805368999647, 1.766732283464566899 ) ) ;
#3350=CARTESIAN_POINT ( 'NONE',  ( 0.1585706980422248169, 0.4669911931914899617, -1.569881889763779625 ) ) ;
#3363=CIRCLE ( 'NONE', #15129, 0.2938622683360631593 ) ;
#3365=CARTESIAN_POINT ( 'NONE',  ( -0.3935368318888682326, 0.3024344094364739277, -1.569881889763779625 ) ) ;
#3376=DIRECTION ( 'NONE',  ( 1.000000000000000000, 0.000000000000000000, 0.000000000000000000 ) ) ;
#3383=CARTESIAN_POINT ( 'NONE',  ( -0.4954247181591361904, -0.1327957795771543825, -1.550196850393700254 ) ) ;
#3385=FACE_BOUND ( 'NONE', #2357, .T. ) ;
#3388=CARTESIAN_POINT ( 'NONE',  ( 0.4954219348937308198, -0.1327952259508279609, -1.550196850393700476 ) ) ;
#3391=CARTESIAN_POINT ( 'NONE',  ( -0.2904160862623646477, -0.1677079028045411757, 1.973425196850393970 ) ) ;
#3392=CARTESIAN_POINT ( 'NONE',  ( 0.3855916753034099864, -0.3382184156749167836, -1.550196850393700920 ) ) ;
#3394=CARTESIAN_POINT ( 'NONE',  ( 0.4783323773986672967, -0.2762247810518773106, 0.9202755905511811330 ) ) ;
#3398=ORIENTED_EDGE ( 'NONE', *, *, #9003, .T. ) ;
#3400=CARTESIAN_POINT ( 'NONE',  ( -0.3252100150720461658, 0.3707612262532960501, -1.569881889763779625 ) ) ;
#3404=CARTESIAN_POINT ( 'NONE',  ( 0.5314960629921260393, 0.000000000000000000, 1.747047244094488194 ) ) ;
#3410=LINE ( 'NONE', #20666, #1187 ) ;
#3416=CARTESIAN_POINT ( 'NONE',  ( 0.2006393256663384084, 0.4069519308876483610, -1.934055118110236338 ) ) ;
#3419=CARTESIAN_POINT ( 'NONE',  ( 0.03190927504541822557, 0.3133984839257918931, -3.179301372150324045 ) ) ;
#3423=ORIENTED_EDGE ( 'NONE', *, *, #2871, .F. ) ;
#3430=CARTESIAN_POINT ( 'NONE',  ( 0.3552036222398872733, -0.04673558830919831431, -3.115157480314960203 ) ) ;
#3433=CARTESIAN_POINT ( 'NONE',  ( 0.4446020952038907681, 0.02909913904662021419, -1.934055118110236338 ) ) ;
#3440=CARTESIAN_POINT ( 'NONE',  ( -0.5280699926563169333, 0.06957181182499308503, 1.747047244094488194 ) ) ;
#3446=CARTESIAN_POINT ( 'NONE',  ( -0.3765118517642104257, -0.02464264302297883638, -3.100567304031763172 ) ) ;
#3460=CARTESIAN_POINT ( 'NONE',  ( 0.2228126397719810137, -0.3858397471888643793, -1.934055118110236338 ) ) ;
#3465=CARTESIAN_POINT ( 'NONE',  ( 0.3213305936751376102, 0.1584254766472200371, -3.115157480314960647 ) ) ;
#3468=DIRECTION ( 'NONE',  ( -0.000000000000000000, -0.000000000000000000, 1.000000000000000000 ) ) ;
#3472=CARTESIAN_POINT ( 'NONE',  ( -2.685748425196850164E-17, 0.000000000000000000, -3.745078740157480546 ) ) ;
#3474=CARTESIAN_POINT ( 'NONE',  ( 0.2676050456844303871, -0.2056553984168022209, 1.973425196850394192 ) ) ;
#3482=CARTESIAN_POINT ( 'NONE',  ( 0.5118110236220472231, 0.000000000000000000, 1.747047244094488194 ) ) ;
#3484=CARTESIAN_POINT ( 'NONE',  ( -0.03349795313264326141, 0.5118110236220472231, 1.747047244094488194 ) ) ;
#3486=CARTESIAN_POINT ( 'NONE',  ( -0.3574975638436101444, 0.02339816079122976691, -3.115157480314960647 ) ) ;
#3489=CARTESIAN_POINT ( 'NONE',  ( -0.4446020952038907681, 0.000000000000000000, -1.934055118110236338 ) ) ;
#3493=CARTESIAN_POINT ( 'NONE',  ( -0.06441834428466612639, 0.4889536969035325753, -1.569881889763779625 ) ) ;
#3522=CARTESIAN_POINT ( 'NONE',  ( -0.04956879678465797578, 0.1968503937007203553, -3.634230943941200831 ) ) ;
#3535=CARTESIAN_POINT ( 'NONE',  ( 0.4599954779394911930, -0.2268956277333457894, -1.550196850393700920 ) ) ;
#3538=CARTESIAN_POINT ( 'NONE',  ( -0.5118110236220763110, -0.03349795313034512750, -1.550196850393700920 ) ) ;
#3539=CARTESIAN_POINT ( 'NONE',  ( 0.4407612517155324872, 0.3387265385688508768, 0.9202755905511812440 ) ) ;
#3540=CARTESIAN_POINT ( 'NONE',  ( -0.5511811023622048555, 0.03607471876259065596, 0.9399606299212598381 ) ) ;
#3568=CARTESIAN_POINT ( 'NONE',  ( -0.3552078253616823833, -0.04672900338023027594, -3.115157480314959759 ) ) ;
#3572=CARTESIAN_POINT ( 'NONE',  ( 0.2712027394948776093, -0.3535065162672919037, -1.934055118110236338 ) ) ;
#3584=CARTESIAN_POINT ( 'NONE',  ( 0.1378076643338917162, 0.5144970376936037759, 1.747047244094488194 ) ) ;
#3590=VECTOR ( 'NONE', #6075, 39.37007874015748143 ) ;
#3591=CARTESIAN_POINT ( 'NONE',  ( 0.3644697409450263215, 0.09762295995069791843, -3.100567304031765836 ) ) ;
#3596=CARTESIAN_POINT ( 'NONE',  ( -0.2669480828848088128, -0.2341512108694275007, 1.953740157480315043 ) ) ;
#3599=CARTESIAN_POINT ( 'NONE',  ( -0.3765118517642104257, 2.305470170520414967E-17, -3.100567304031763172 ) ) ;
#3600=CARTESIAN_POINT ( 'NONE',  ( -0.5526079293737016229, 0.1480156394741962422, 0.9399606299212598381 ) ) ;
#3607=CARTESIAN_POINT ( 'NONE',  ( 0.2842490391651530390, 0.2180698645301770711, -3.115157480314960647 ) ) ;
#3608=CARTESIAN_POINT ( 'NONE',  ( 0.1442704874421230632, -0.5368353335967093187, 0.9202755905511807999 ) ) ;
#3616=ADVANCED_FACE ( 'NONE', ( #26434 ), #7101, .T. ) ;
#3627=CARTESIAN_POINT ( 'NONE',  ( 0.4441657790107856330, -0.2564944395515579845, 1.766732283464566899 ) ) ;
#3637=CARTESIAN_POINT ( 'NONE',  ( 0.4669911931914377257, 0.1585706980422264545, -1.550196850393700920 ) ) ;
#3640=ORIENTED_EDGE ( 'NONE', *, *, #23073, .T. ) ;
#3665=DIRECTION ( 'NONE',  ( 0.000000000000000000, 0.000000000000000000, 1.000000000000000000 ) ) ;
#3683=CARTESIAN_POINT ( 'NONE',  ( 0.2904160862623688666, 0.1677079028045472542, 1.953740157480315043 ) ) ;
#3686=CARTESIAN_POINT ( 'NONE',  ( 0.1429116519061375268, 0.5335524835332416949, 0.9399606299212598381 ) ) ;
#3693=CARTESIAN_POINT ( 'NONE',  ( 0.3454440660767458815, 0.3030032861725153737, -1.928289503579147635 ) ) ;
#3698=CARTESIAN_POINT ( 'NONE',  ( 0.06947563356181042649, 0.5280876769850310071, 1.747047244094488194 ) ) ;
#3703=ORIENTED_EDGE ( 'NONE', *, *, #12278, .T. ) ;
#3706=CARTESIAN_POINT ( 'NONE',  ( -0.3511566718596346171, -0.4004902621171045340, 1.747047244094487528 ) ) ;
#3725=CARTESIAN_POINT ( 'NONE',  ( 0.06441834428466665374, -0.4889536969035324088, -1.569881889763779625 ) ) ;
#3727=CARTESIAN_POINT ( 'NONE',  ( 0.1432577568504609655, -0.4218945342797526532, -1.934055118110236338 ) ) ;
#3729=EDGE_CURVE ( 'NONE', #7673, #3938, #13479, .T. ) ;
#3735=CARTESIAN_POINT ( 'NONE',  ( -0.1378076643338909391, 0.5144970376935737999, 1.747047244094488194 ) ) ;
#3741=CARTESIAN_POINT ( 'NONE',  ( -0.2488091035917020799, -0.2836590635674518524, -3.100567304031764948 ) ) ;
#3744=CARTESIAN_POINT ( 'NONE',  ( -0.02319089060378104472, -0.3543307086614173596, 1.953740157480315043 ) ) ;
#3750=CARTESIAN_POINT ( 'NONE',  ( 0.5335524835332418059, -0.1429116519061131296, 0.9399606299212598381 ) ) ;
#3756=CARTESIAN_POINT ( 'NONE',  ( 0.1151913129404419367, -0.3392387706403586223, -3.115157480314960647 ) ) ;
#3758=CARTESIAN_POINT ( 'NONE',  ( 0.000000000000000000, 0.000000000000000000, 1.914370078775489148 ) ) ;
#3765=CARTESIAN_POINT ( 'NONE',  ( -0.3149606299212598381, 3.857155272905049219E-17, -3.745078740157480546 ) ) ;
#3766=ADVANCED_FACE ( 'NONE', ( #20084 ), #4410, .T. ) ;
#3773=VECTOR ( 'NONE', #17359, 39.37007874015748143 ) ;
#3778=CARTESIAN_POINT ( 'NONE',  ( 0.4600326175560556230, -0.2268096725222457644, 1.766732283464566899 ) ) ;
#3788=CARTESIAN_POINT ( 'NONE',  ( 0.2904160862623631489, 0.1677079028045434517, 1.973425196850393970 ) ) ;
#3790=ORIENTED_EDGE ( 'NONE', *, *, #14504, .F. ) ;
#3791=CARTESIAN_POINT ( 'NONE',  ( 0.3252100150720381722, -0.3707612262533039327, -1.550196850393700920 ) ) ;
#3798=CARTESIAN_POINT ( 'NONE',  ( 0.000000000000000000, 0.000000000000000000, 1.707677165389662743 ) ) ;
#3799=VECTOR ( 'NONE', #27879, 39.37007874015748854 ) ;
#3820=CARTESIAN_POINT ( 'NONE',  ( -0.4954415918535808872, -0.1327036767636090853, -1.550196850393700920 ) ) ;
#3823=CARTESIAN_POINT ( 'NONE',  ( -0.03607471876262472593, 0.5511811023622047445, 0.9202755905511811330 ) ) ;
#3827=ORIENTED_EDGE ( 'NONE', *, *, #10852, .F. ) ;
#3831=CARTESIAN_POINT ( 'NONE',  ( -0.4068940122753434974, -0.3122781343786983355, -1.550196850393701142 ) ) ;
#3838=CARTESIAN_POINT ( 'NONE',  ( -0.02190250779246035590, 0.3346456692913385988, 1.953740157480315043 ) ) ;
#3839=CARTESIAN_POINT ( 'NONE',  ( 0.1327036767636163017, -0.4954415918535808872, -1.550196850393700920 ) ) ;
#3841=CARTESIAN_POINT ( 'NONE',  ( 0.5476281405333121022, -0.07214854559198019546, 0.9399606299212598381 ) ) ;
#3845=CARTESIAN_POINT ( 'NONE',  ( 0.2181214148710974021, 0.2842163005027489864, -3.115157480314961091 ) ) ;
#3849=CARTESIAN_POINT ( 'NONE',  ( 0.5144751499634915293, 0.1379104267273083551, 1.747047244094488194 ) ) ;
#3852=CARTESIAN_POINT ( 'NONE',  ( 0.03349795313024148125, 0.5118110236220473341, -1.550196850393700920 ) ) ;
#3857=CARTESIAN_POINT ( 'NONE',  ( -0.2662775206742153955, -0.4613022222208275624, 1.747047244094488194 ) ) ;
#3865=CARTESIAN_POINT ( 'NONE',  ( 0.07874015748031489015, 0.1968503937007874127, -3.272637795275590733 ) ) ;
#3873=B_SPLINE_CURVE_WITH_KNOTS ( 'NONE', 3,
 ( #18048, #11443, #11862, #9045, #26280, #7206, #581, #2806, #15694, #6946, #13699, #20064, #7078, #17659, #24297, #718, #15568, #13418 ),
 .UNSPECIFIED., .F., .F.,
 ( 4, 2, 2, 2, 2, 2, 2, 2, 4 ),
 ( 0.5000000000000000000, 0.5625000000000000000, 0.6250000000000000000, 0.6875000000000000000, 0.7500000000000000000, 0.8125000000000000000, 0.8750000000000000000, 0.9375000000000000000, 1.000000000000000000 ),
 .UNSPECIFIED. ) ;
#3874=CARTESIAN_POINT ( 'NONE',  ( 0.4669911931914907388, -0.1585706980422228185, -1.569881889763779625 ) ) ;
#3876=CARTESIAN_POINT ( 'NONE',  ( -0.3929158813954686247, -0.2268989272875759633, -1.934055118110236338 ) ) ;
#3878=CARTESIAN_POINT ( 'NONE',  ( -0.4351030398461734339, 0.1477428134820354677, -1.928289503579158959 ) ) ;
#3883=CARTESIAN_POINT ( 'NONE',  ( 0.4612490782035170156, 0.2663596103035609786, 1.747047244094488194 ) ) ;
#3885=CARTESIAN_POINT ( 'NONE',  ( 0.3937007874015748254, 0.000000000000000000, -3.036417322828325105 ) ) ;
#3889=CARTESIAN_POINT ( 'NONE',  ( 0.4446020952038907681, 5.549066237130534971E-17, -1.934055118110236338 ) ) ;
#3890=CARTESIAN_POINT ( 'NONE',  ( -0.3074993854542726890, 0.1775730735577450703, 1.953740157480315043 ) ) ;
#3903=CARTESIAN_POINT ( 'NONE',  ( -0.2180698645301767380, -0.2842490391651532611, -3.115157480314960647 ) ) ;
#3904=CARTESIAN_POINT ( 'NONE',  ( -0.5368353335967092077, -0.1442704874421231187, 0.9202755905511812440 ) ) ;
#3912=DIRECTION ( 'NONE',  ( 0.000000000000000000, 0.000000000000000000, 1.000000000000000000 ) ) ;
#3920=CARTESIAN_POINT ( 'NONE',  ( -0.4069448477556031341, -0.3121994997598085408, 1.747047244094488194 ) ) ;
#3925=CARTESIAN_POINT ( 'NONE',  ( -0.2272836761398000505, 0.2962590301041647667, -3.115157480314960647 ) ) ;
#3931=B_SPLINE_CURVE_WITH_KNOTS ( 'NONE', 3,
 ( #12660, #21291, #1927, #25662, #6316, #21427, #2065, #17591, #11098, #4593, #26207, #641, #24226, #11369, #2872, #19987, #3007, #7004 ),
 .UNSPECIFIED., .F., .F.,
 ( 4, 2, 2, 2, 2, 2, 2, 2, 4 ),
 ( 0.5000000000000000000, 0.5625000000000000000, 0.6250000000000000000, 0.6875000000000000000, 0.7500000000000000000, 0.8125000000000000000, 0.8750000000000001110, 0.9375000000000000000, 1.000000000000000000 ),
 .UNSPECIFIED. ) ;
#3932=CARTESIAN_POINT ( 'NONE',  ( -0.1677079028045370956, -0.2904160862623674233, 1.973425196850393970 ) ) ;
#3935=CARTESIAN_POINT ( 'NONE',  ( -0.2466292688015410683, 0.4270824798167730529, -1.550196850393700920 ) ) ;
#3938=VERTEX_POINT ( 'NONE', #362 ) ;
#3943=CARTESIAN_POINT ( 'NONE',  ( 0.1431849087165211198, -0.4219262446670075661, -1.934055118110236338 ) ) ;
#3971=CARTESIAN_POINT ( 'NONE',  ( 0.2762247810519147251, 0.4783323773986423166, 0.9202755905511811330 ) ) ;
#3987=CARTESIAN_POINT ( 'NONE',  ( -0.5417097841048968965, 0.1839420097223028183, 0.9399606299212598381 ) ) ;
#3990=VERTEX_POINT ( 'NONE', #17820 ) ;
#3991=CARTESIAN_POINT ( 'NONE',  ( -0.2362017869178774654, 0.2693781226336497969, -3.115157480314962424 ) ) ;
#3992=ADVANCED_FACE ( 'NONE', ( #13174 ), #8230, .T. ) ;
#3999=CARTESIAN_POINT ( 'NONE',  ( -0.4954415918535620134, 0.1327036767636087800, -1.550196850393700920 ) ) ;
#4000=CARTESIAN_POINT ( 'NONE',  ( -0.1481194149836671525, -0.5525858403826198195, 0.9399606299212598381 ) ) ;
#4001=EDGE_CURVE ( 'NONE', #21690, #5829, #13698, .T. ) ;
#4005=CARTESIAN_POINT ( 'NONE',  ( 0.3122765577851944196, 0.4068916527368734437, -1.550196850393701142 ) ) ;
#4020=CARTESIAN_POINT ( 'NONE',  ( -0.3030032861725269200, 0.3454440660767091886, -1.928289503579165620 ) ) ;
#4028=CARTESIAN_POINT ( 'NONE',  ( -0.03478633594543645985, -0.5314960629921260393, 1.747047244094488194 ) ) ;
#4030=EDGE_LOOP ( 'NONE', ( #13868, #12961, #18175, #3423 ) ) ;
#4040=CARTESIAN_POINT ( 'NONE',  ( 0.3429980251342366060, 0.09187177619658697114, 1.953740157480315043 ) ) ;
#4042=CIRCLE ( 'NONE', #5861, 0.4724409448465559103 ) ;
#4050=CARTESIAN_POINT ( 'NONE',  ( 0.3535721684718142188, -0.1200583359873150652, -3.115157480314960647 ) ) ;
#4059=CARTESIAN_POINT ( 'NONE',  ( 0.2860025288258006282, 0.4954757973262963189, 0.9399606299212598381 ) ) ;
#4065=CARTESIAN_POINT ( 'NONE',  ( -0.5085118447801436625, -0.06699507805368999647, 1.766732283464566899 ) ) ;
#4067=CARTESIAN_POINT ( 'NONE',  ( -0.2564944395516098874, 0.4441657790107518822, 1.747047244094488194 ) ) ;
#4070=CARTESIAN_POINT ( 'NONE',  ( 0.02339816079119088829, 0.3574975638436101444, -3.115157480314960647 ) ) ;
#4072=CARTESIAN_POINT ( 'NONE',  ( -0.4585215200179058037, -0.06002032661671150016, -1.928289503579156516 ) ) ;
#4075=CARTESIAN_POINT ( 'NONE',  ( -0.2904160862623674788, 0.1677079028045369846, 1.973425196850393970 ) ) ;
#4077=CARTESIAN_POINT ( 'NONE',  ( -0.03220957031754000111, 0.4921259842519685179, -1.550196850393700920 ) ) ;
#4086=CARTESIAN_POINT ( 'NONE',  ( -0.03190474515785463733, 0.3133989528012832704, -3.641566340106785038 ) ) ;
#4095=CARTESIAN_POINT ( 'NONE',  ( -0.4585215200179055817, 0.06002032661671174996, -1.928289503579156516 ) ) ;
#4097=CARTESIAN_POINT ( 'NONE',  ( 0.3135473077061334268, 3.969037272548740164E-17, 2.504921259842519898 ) ) ;
#4102=CARTESIAN_POINT ( 'NONE',  ( 0.4921259842519685179, 0.000000000000000000, -1.894685039405410665 ) ) ;
#4107=EDGE_LOOP ( 'NONE', ( #8858, #19737, #10539, #2313 ) ) ;
#4112=CARTESIAN_POINT ( 'NONE',  ( 0.5511811023622047445, 0.03607471876262480226, 0.9202755905511811330 ) ) ;
#4122=CARTESIAN_POINT ( 'NONE',  ( 0.3149606299212598381, 0.000000000000000000, -3.115157480314960647 ) ) ;
#4124=CARTESIAN_POINT ( 'NONE',  ( 0.2521176338356617697, -0.2211428102655709493, 1.973425196850393970 ) ) ;
#4129=CARTESIAN_POINT ( 'NONE',  ( 0.07214854559195596484, 0.5476281405333121022, 0.9399606299212598381 ) ) ;
#4136=CARTESIAN_POINT ( 'NONE',  ( 0.4441657790094322711, 0.2564944395535476707, -1.550196850393700920 ) ) ;
#4137=CARTESIAN_POINT ( 'NONE',  ( 0.2530785775249113079, -0.5130740159361732999, 0.9399606299212600602 ) ) ;
#4156=CARTESIAN_POINT ( 'NONE',  ( -0.4921259842519685179, -0.03220957031763953954, -1.569881889763779625 ) ) ;
#4158=CARTESIAN_POINT ( 'NONE',  ( -0.02963280468032113146, 0.4527559054764770385, -1.934055118110236338 ) ) ;
#4162=B_SPLINE_CURVE_WITH_KNOTS ( 'NONE', 3,
 ( #12876, #14760, #4272, #12465, #14611, #2148, #25743, #23368, #12738, #3991, #27870, #10614, #21646, #10763, #5977, #21366, #6396, #19379, #77, #23214, #8505, #19238, #27732, #3845, #12606, #1868, #10474, #19093, #16989, #14892, #23501, #26414, #2809, #22325 ),
 .UNSPECIFIED., .F., .F.,
 ( 4, 2, 2, 2, 2, 2, 2, 2, 2, 2, 2, 2, 2, 2, 2, 2, 4 ),
 ( 0.000000000000000000, 0.03124999999999996531, 0.06249999999999993061, 0.09374999999999988898, 0.1249999999999998890, 0.1562499999999998612, 0.1874999999999998335, 0.2187499999999998335, 0.2499999999999998335, 0.2812499999999997780, 0.3124999999999997780, 0.3437499999999997224, 0.3749999999999997224, 0.4062499999999997780, 0.4374999999999998335, 0.4687499999999999445, 0.5000000000000000000 ),
 .UNSPECIFIED. ) ;
#4167=CARTESIAN_POINT ( 'NONE',  ( 0.4004221243553557907, -0.3512268162760437407, 1.747047244094488194 ) ) ;
#4173=B_SPLINE_SURFACE_WITH_KNOTS ( 'NONE', 2, 3, ( 
 ( #10173, #18791, #27428, #12455, #13285, #11162, #14883, #23715, #5306, #7860, #25215, #20637, #9463, #7499, #5670, #17927, #13710, #878 ),
 ( #18056, #16126, #26999, #20210, #5386, #24866, #3522, #22474, #24722, #12022, #9604, #18209, #26699, #24583, #9318, #14005, #22617, #26846 ),
 ( #15980, #7215, #15833, #3104, #3236, #22332, #20495, #11877, #11736, #9897, #1010, #1153, #27143, #22906, #18354, #16399, #5529, #14151 ) ),
 .UNSPECIFIED., .F., .F., .F.,
 ( 3, 3 ),
 ( 4, 2, 2, 2, 2, 2, 2, 2, 4 ),
 ( 0.000000000000000000, 1.000000000000000000 ),
 ( 4.712388980384689674, 5.105088062083414258, 5.497787143782137953, 5.890486225480861648, 6.283185307179586232, 6.675884388878310816, 7.068583470577034511, 7.461282552275758206, 7.853981633974482790 ),
 .UNSPECIFIED. ) ;
#4177=CARTESIAN_POINT ( 'NONE',  ( 0.02319089060378159983, 0.3543307086614173596, 1.953740157480315043 ) ) ;
#4178=ORIENTED_EDGE ( 'NONE', *, *, #6267, .F. ) ;
#4187=CARTESIAN_POINT ( 'NONE',  ( 0.1867299569291683836, 0.3233561589689052940, -3.115157480314960647 ) ) ;
#4188=CARTESIAN_POINT ( 'NONE',  ( -0.09586345242798399724, 0.2165354330708661734, -3.573990933499928691 ) ) ;
#4202=CARTESIAN_POINT ( 'NONE',  ( -0.4441657790107744752, -0.2564944395515745823, 1.766732283464566899 ) ) ;
#4203=CARTESIAN_POINT ( 'NONE',  ( -0.5118110236220472231, 0.03349795313264340019, 1.747047244094488194 ) ) ;
#4209=CARTESIAN_POINT ( 'NONE',  ( 0.3102476824511484210, 0.1791601451668926315, -3.115157480314960647 ) ) ;
#4214=CARTESIAN_POINT ( 'NONE',  ( 0.1482986320106399469, 0.3007905576423889893, 1.973425196850393970 ) ) ;
#4217=CARTESIAN_POINT ( 'NONE',  ( -0.1585706980422388890, 0.4669911931914605963, -1.550196850393700920 ) ) ;
#4237=EDGE_CURVE ( 'NONE', #15069, #804, #19759, .T. ) ;
#4242=CARTESIAN_POINT ( 'NONE',  ( 0.06880207798751564185, 0.1968503937007873850, -3.232982757847921995 ) ) ;
#4250=CARTESIAN_POINT ( 'NONE',  ( -0.3362148458988422073, 0.4382482975805319092, 0.9202755905511811330 ) ) ;
#4259=CONICAL_SURFACE ( 'NONE', #7865, 0.2938622683360631593, 0.2617993874999998138 ) ;
#4260=ADVANCED_FACE ( 'NONE', ( #18874 ), #10125, .T. ) ;
#4270=DIRECTION ( 'NONE',  ( -0.000000000000000000, -0.000000000000000000, -1.000000000000000000 ) ) ;
#4272=CARTESIAN_POINT ( 'NONE',  ( -0.3552036222399427290, 0.04673558830906447692, -3.115157480314960647 ) ) ;
#4277=CARTESIAN_POINT ( 'NONE',  ( -0.4763861460130774939, -0.1275996891957774104, -1.550196850393700920 ) ) ;
#4278=CARTESIAN_POINT ( 'NONE',  ( 0.5672083774005964862, -0.07462150385395434349, 0.9399606299212600602 ) ) ;
#4281=CARTESIAN_POINT ( 'NONE',  ( -0.5314960629921260393, 6.402768735150616610E-17, 1.747047244094488194 ) ) ;
#4295=CARTESIAN_POINT ( 'NONE',  ( 0.3252100150720097504, 0.3707612262533033776, -1.550196850393700920 ) ) ;
#4299=CARTESIAN_POINT ( 'NONE',  ( 0.2006393256663695779, -0.4069519308876702324, -1.934055118110236338 ) ) ;
#4310=CARTESIAN_POINT ( 'NONE',  ( -0.4446020952038907126, 0.02918571160814592211, -1.934055118110236560 ) ) ;
#4317=CARTESIAN_POINT ( 'NONE',  ( 0.03736310157557471562, -0.5708661417322835607, 0.9399606299212598381 ) ) ;
#4322=CARTESIAN_POINT ( 'NONE',  ( 0.2962590301041581609, -0.2272836761397895311, -3.115157480314960647 ) ) ;
#4327=FACE_OUTER_BOUND ( 'NONE', #24593, .T. ) ;
#4339=CARTESIAN_POINT ( 'NONE',  ( -0.03349795313264251895, -0.5118110236220473341, 1.766732283464566899 ) ) ;
#4344=CARTESIAN_POINT ( 'NONE',  ( -0.3551931031211721379, -0.04679574315772278004, -3.115157480314960647 ) ) ;
#4350=CARTESIAN_POINT ( 'NONE',  ( -0.3324885138898245329, -0.04380447413658584976, 1.973425196850393970 ) ) ;
#4351=VERTEX_POINT ( 'NONE', #6518 ) ;
#4364=EDGE_CURVE ( 'NONE', #18101, #724, #17498, .T. ) ;
#4373=CARTESIAN_POINT ( 'NONE',  ( 0.01288382760289561411, 0.1968503937007873850, -3.174212598425197207 ) ) ;
#4385=CARTESIAN_POINT ( 'NONE',  ( -0.5335524835332334792, -0.1429116519061227608, 0.9202755905511811330 ) ) ;
#4400=CARTESIAN_POINT ( 'NONE',  ( -0.07874015748031495954, 0.1968503937007873850, -3.364501312335955063 ) ) ;
#4406=CARTESIAN_POINT ( 'NONE',  ( -0.03736310157557561074, 0.5708661417322835607, 0.9399606299212598381 ) ) ;
#4407=CARTESIAN_POINT ( 'NONE',  ( 0.03359157810863758198, -0.5118124425184569226, -1.550196850393701142 ) ) ;
#4410=B_SPLINE_SURFACE_WITH_KNOTS ( 'NONE', 2, 3, ( 
 ( #16141, #18225, #27158, #16277, #26568, #741, #7660, #9329, #24737, #26861, #22490, #15847, #15994, #7227, #5398, #13583, #18508, #13724, #14017, #22629, #24321, #9767, #22345, #11891, #4970, #2971, #18363, #11606, #1169, #20227, #886, #24880, #27014, #9473, #5539, #26712, #14163, #22764, #3391, #22204, #2832, #7372, #24594, #5248, #13870, #3118, #20366, #1024, #1433, #5830, #27582, #23204, #10327, #1860, #18945, #1578, #10045, #4124, #8224, #7942, #23358, #18651, #21218, #16843, #19229, #1996 ),
 ( #6250, #14753, #27432, #27292, #14454, #23065, #3683, #12308, #20933, #10178, #18796, #25451, #25311, #10467, #8087, #16699, #5970, #3838, #12458, #12598, #27724, #21066, #1715, #12004, #5367, #24850, #18042, #574, #11856, #13693, #26538, #22457, #15687, #13990, #22314, #2801, #9170, #11435, #13557, #7481, #11577, #20477, #26978, #1136, #9738, #20193, #14127, #856, #9442, #20058, #7630, #11716, #7343, #22734, #17789, #26408, #15962, #711, #24564, #5216, #7072, #13841, #3084, #20338, #16250, #995 ),
 ( #9583, #24293, #4941, #22176, #9303, #817, #18010, #15658, #4904, #9405, #22424, #26375, #26648, #3046, #26945, #17879, #7303, #26795, #13659, #15924, #13516, #20023, #4764, #24530, #5178, #13807, #11681, #24258, #16211, #7591, #22142, #20304, #17758, #961, #9548, #22012, #24665, #7036, #542, #16071, #9137, #18153, #7441, #5330, #2770, #13952, #9265, #22564, #2645, #9701, #26504, #3190, #11822, #11273, #20442, #7169, #1105, #19892, #15790, #18300, #27090, #8298, #8159, #20725, #22849, #18734 ) ),
 .UNSPECIFIED., .F., .T., .F.,
 ( 3, 3 ),
 ( 4, 2, 2, 2, 2, 2, 2, 2, 2, 2, 2, 2, 2, 2, 2, 2, 2, 2, 2, 2, 2, 2, 2, 2, 2, 2, 2, 2, 2, 2, 2, 2, 4 ),
 ( 0.000000000000000000, 1.000000000000000000 ),
 ( 0.000000000000000000, 0.1963495408493620697, 0.3926990816987241395, 0.5890486225480862092, 0.7853981633974482790, 0.9817477042468103487, 1.178097245096172418, 1.374446785945534488, 1.570796326794896558, 1.767145867644258628, 1.963495408493620697, 2.159844949342982545, 2.356194490192344837, 2.552544031041707129, 2.748893571891068976, 2.945243112740430824, 3.141592653589793116, 3.337942194439155408, 3.534291735288517255, 3.730641276137879103, 3.926990816987241395, 4.123340357836603687, 4.319689898685965090, 4.516039439535327382, 4.712388980384689674, 4.908738521234051966, 5.105088062083414258, 5.301437602932775661, 5.497787143782137953, 5.694136684631500245, 5.890486225480861648, 6.086835766330223940, 6.283185307179586232 ),
 .UNSPECIFIED. ) ;
#4420=CARTESIAN_POINT ( 'NONE',  ( 0.3121994997578272368, 0.4069448477569235778, -1.550196850393700920 ) ) ;
#4424=CARTESIAN_POINT ( 'NONE',  ( -0.2564158049324432587, 0.4442166144912507164, -1.550196850393700920 ) ) ;
#4436=EDGE_LOOP ( 'NONE', ( #7593, #13367, #19602, #25805 ) ) ;
#4439=CARTESIAN_POINT ( 'NONE',  ( -0.03220957031754000111, 0.4921259842519685179, -1.550196850393700920 ) ) ;
#4440=CARTESIAN_POINT ( 'NONE',  ( 0.3411003281197161341, 0.2991932138496539162, -1.934055118110236338 ) ) ;
#4450=CARTESIAN_POINT ( 'NONE',  ( 0.2712695779737101520, 0.3534635626042424428, -1.934055118110236560 ) ) ;
#4460=CARTESIAN_POINT ( 'NONE',  ( 0.4446020952038907681, 5.549066237130534971E-17, -1.934055118110236338 ) ) ;
#4461=CARTESIAN_POINT ( 'NONE',  ( 0.2462256503455911016, 0.2807137536170354331, -3.115157480314960647 ) ) ;
#4478=CARTESIAN_POINT ( 'NONE',  ( 0.3382184156732163660, 0.3855916753051394363, 1.766732283464566899 ) ) ;
#4483=AXIS2_PLACEMENT_3D ( 'NONE', #3323, #3468, #20296 ) ;
#4490=CARTESIAN_POINT ( 'NONE',  ( -0.2904160862623708650, 0.1677079028045392328, 1.953740157480315043 ) ) ;
#4498=DIRECTION ( 'NONE',  ( -0.000000000000000000, -0.000000000000000000, 1.000000000000000000 ) ) ;
#4505=LINE ( 'NONE', #6767, #10977 ) ;
#4512=CARTESIAN_POINT ( 'NONE',  ( -0.06880207798751733494, 0.1968503937007873850, -3.232982757847917554 ) ) ;
#4521=CARTESIAN_POINT ( 'NONE',  ( 0.000000000000000000, 0.000000000000000000, 1.953740157480315043 ) ) ;
#4527=CARTESIAN_POINT ( 'NONE',  ( 0.1775991818008583745, 0.5230301363771922007, 0.9399606299212598381 ) ) ;
#4545=CARTESIAN_POINT ( 'NONE',  ( -0.4300830224589284878, -0.3772436174784035146, 0.9399606299212598381 ) ) ;
#4563=CARTESIAN_POINT ( 'NONE',  ( 0.06046064452055317090, 0.3092451502564478871, -3.626963221729183839 ) ) ;
#4566=CARTESIAN_POINT ( 'NONE',  ( 0.1477428134820237549, -0.4351030398461813720, -1.928289503579156294 ) ) ;
#4567=CARTESIAN_POINT ( 'NONE',  ( -0.5511811023622047445, 0.000000000000000000, 0.9202755905511811330 ) ) ;
#4574=CIRCLE ( 'NONE', #17640, 0.5511811023268710086 ) ;
#4582=CARTESIAN_POINT ( 'NONE',  ( -0.05926487674658593302, 0.4498374011143062567, -1.934055118110236338 ) ) ;
#4593=CARTESIAN_POINT ( 'NONE',  ( -0.06441914069860958658, -0.4921259842519685179, -1.569881889763779403 ) ) ;
#4597=LINE ( 'NONE', #9107, #6365 ) ;
#4598=CARTESIAN_POINT ( 'NONE',  ( 0.2268096725222374654, 0.4600326175560591202, 1.766732283464566899 ) ) ;
#4604=CARTESIAN_POINT ( 'NONE',  ( 0.3535721684718142188, -0.1200583359873150652, -3.115157480314960647 ) ) ;
#4620=ADVANCED_FACE ( 'NONE', ( #13735 ), #14309, .T. ) ;
#4639=CARTESIAN_POINT ( 'NONE',  ( 0.2341095169845144042, -0.2669917830071620313, 1.953740157480315043 ) ) ;
#4644=FACE_OUTER_BOUND ( 'NONE', #18336, .T. ) ;
#4648=CARTESIAN_POINT ( 'NONE',  ( -0.03607471876262562105, -0.5511811023622046335, 0.9202755905511811330 ) ) ;
#4666=CARTESIAN_POINT ( 'NONE',  ( 0.2860899518037664513, 0.4954156765914491944, 0.9399606299212598381 ) ) ;
#4668=FACE_OUTER_BOUND ( 'NONE', #11145, .T. ) ;
#4674=CARTESIAN_POINT ( 'NONE',  ( -0.1327036767636080028, -0.4954415918535519658, -1.550196850393700920 ) ) ;
#4682=CARTESIAN_POINT ( 'NONE',  ( 0.5511811023622047445, 0.000000000000000000, -1.550196850393700920 ) ) ;
#4692=CARTESIAN_POINT ( 'NONE',  ( -0.4585215200179055817, 0.000000000000000000, -1.928289503579156516 ) ) ;
#4694=CARTESIAN_POINT ( 'NONE',  ( 0.3645739570812638330, -0.2796934465393868807, -1.928289503579156072 ) ) ;
#4697=CARTESIAN_POINT ( 'NONE',  ( -0.06001958459474868862, 0.4555658499976078524, -1.928289503579158515 ) ) ;
#4706=ADVANCED_FACE ( 'NONE', ( #11033 ), #15154, .T. ) ;
#4722=CARTESIAN_POINT ( 'NONE',  ( 0.3572819248074444731, 0.1213180142433879782, -3.100567304031760951 ) ) ;
#4735=CARTESIAN_POINT ( 'NONE',  ( -0.1649135259617106886, 0.4856708409200803378, 1.747047244094488194 ) ) ;
#4741=CARTESIAN_POINT ( 'NONE',  ( -0.2462256503456003442, -0.2807137536170363767, -3.115157480314960647 ) ) ;
#4745=CARTESIAN_POINT ( 'NONE',  ( -0.2211428102655801364, -0.2521176338356625468, 1.953740157480315043 ) ) ;
#4755=CARTESIAN_POINT ( 'NONE',  ( -0.03962986251637951735, 0.1968503937007874127, -3.617043892030582963 ) ) ;
#4764=CARTESIAN_POINT ( 'NONE',  ( -0.1775730735577547292, 0.3074993854542629190, 1.953740157480315043 ) ) ;
#4770=CARTESIAN_POINT ( 'NONE',  ( -2.685748425196850164E-17, 0.000000000000000000, -3.745078740157480546 ) ) ;
#4771=CARTESIAN_POINT ( 'NONE',  ( -0.03349795313264326141, 0.5118110236220472231, 1.766732283464566899 ) ) ;
#4780=CARTESIAN_POINT ( 'NONE',  ( -0.4921259842519685179, 0.03220957031763950484, -1.569881889763779625 ) ) ;
#4783=CARTESIAN_POINT ( 'NONE',  ( 0.1775991818008606782, -0.5230301363771325818, 0.9202755905511811330 ) ) ;
#4784=ORIENTED_EDGE ( 'NONE', *, *, #5227, .F. ) ;
#4791=CARTESIAN_POINT ( 'NONE',  ( -2.685748425196850164E-17, 0.000000000000000000, -3.115157480314960647 ) ) ;
#4802=CARTESIAN_POINT ( 'NONE',  ( 0.5131133041954023533, 0.2529800193559384458, 0.9399606299212598381 ) ) ;
#4824=CARTESIAN_POINT ( 'NONE',  ( -0.04956879728060041568, 0.2165354330708661457, -3.634230943735655472 ) ) ;
#4828=CARTESIAN_POINT ( 'NONE',  ( -1.452994488188976472E-16, 0.3149606299212598381, -3.646653543307086576 ) ) ;
#4829=CARTESIAN_POINT ( 'NONE',  ( 0.2268096725200263730, 0.4600326175569572351, -1.550196850393700920 ) ) ;
#4831=CARTESIAN_POINT ( 'NONE',  ( -0.03001016326913591784, 0.4585215200179055817, -1.928289503579156516 ) ) ;
#4832=AXIS2_PLACEMENT_3D ( 'NONE', #8544, #25638, #106 ) ;
#4839=( CONVERSION_BASED_UNIT ( 'INCH', #1181 ) LENGTH_UNIT ( ) NAMED_UNIT ( #27099 ) ) ;
#4852=CARTESIAN_POINT ( 'NONE',  ( -0.3349573549949665940, -0.2938049579018697788, -1.934055118110236338 ) ) ;
#4854=CARTESIAN_POINT ( 'NONE',  ( -0.5118110236220473341, 0.000000000000000000, -1.550196850393700920 ) ) ;
#4858=CARTESIAN_POINT ( 'NONE',  ( 0.1153552079389292689, -0.4303653410901767673, -1.934055118110235894 ) ) ;
#4859=CARTESIAN_POINT ( 'NONE',  ( 0.2296683860596776539, 0.2993674444872277962, -3.100567304031764060 ) ) ;
#4874=CARTESIAN_POINT ( 'NONE',  ( -0.4472135058506044869, 0.2577577458591217008, 1.766732283464566899 ) ) ;
#4875=CARTESIAN_POINT ( 'NONE',  ( -0.3855916753051391033, -0.3382184156731863900, 1.747047244094488194 ) ) ;
#4881=CARTESIAN_POINT ( 'NONE',  ( 0.3535721684717935132, 0.1200583359873110406, -3.115157480314960647 ) ) ;
#4887=CARTESIAN_POINT ( 'NONE',  ( -0.04380447413658832695, 0.3324885138898346360, 1.953740157480315043 ) ) ;
#4888=EDGE_CURVE ( 'NONE', #16690, #8508, #6581, .T. ) ;
#4896=EDGE_LOOP ( 'NONE', ( #15308, #27700, #5949, #22955 ) ) ;
#4903=DIRECTION ( 'NONE',  ( -1.000000000000000000, 0.000000000000000000, 0.000000000000000000 ) ) ;
#4904=CARTESIAN_POINT ( 'NONE',  ( 0.2669480828848126985, 0.2341512108694336625, 1.953740157480315043 ) ) ;
#4912=CARTESIAN_POINT ( 'NONE',  ( -0.5511811023622047445, 6.750021727583836750E-17, -1.550196850393700920 ) ) ;
#4921=ORIENTED_EDGE ( 'NONE', *, *, #15428, .T. ) ;
#4925=CARTESIAN_POINT ( 'NONE',  ( -0.3362148458988263311, -0.4382482975805425118, 0.9202755905511811330 ) ) ;
#4928=VERTEX_POINT ( 'NONE', #7233 ) ;
#4930=DIRECTION ( 'NONE',  ( 1.000000000000000000, 0.000000000000000000, 0.000000000000000000 ) ) ;
#4940=ADVANCED_FACE ( 'NONE', ( #13450 ), #5255, .T. ) ;
#4941=CARTESIAN_POINT ( 'NONE',  ( 0.3520466617656906050, 0.04638120790933070170, 1.953740157480315043 ) ) ;
#4946=CARTESIAN_POINT ( 'NONE',  ( 0.03736310157557554135, 0.5708661417322835607, 0.9399606299212598381 ) ) ;
#4952=CIRCLE ( 'NONE', #23497, 0.5905511811023621549 ) ;
#4959=CARTESIAN_POINT ( 'NONE',  ( -0.07874015748031511219, 0.1968503937007874127, -3.548228346456693050 ) ) ;
#4970=CARTESIAN_POINT ( 'NONE',  ( -0.2211428102655755012, 0.2521176338356572177, 1.973425196850393970 ) ) ;
#4972=CARTESIAN_POINT ( 'NONE',  ( 0.4669911931914963454, -0.1585706980422251222, -1.550196850393700920 ) ) ;
#4973=CARTESIAN_POINT ( 'NONE',  ( 0.2297883689023126064, 0.3979194638820598984, -1.928289503579157183 ) ) ;
#4975=CARTESIAN_POINT ( 'NONE',  ( 0.2442565704126475612, 0.4954197419817565895, 0.9202755905511811330 ) ) ;
#4981=LINE ( 'NONE', #13597, #13625 ) ;
#4987=CARTESIAN_POINT ( 'NONE',  ( 0.3543307086614173596, 0.000000000000000000, 1.953740157480315043 ) ) ;
#4998=CARTESIAN_POINT ( 'NONE',  ( 0.1213180142433946118, -0.3572819248074403653, -3.100567304031765392 ) ) ;
#5007=VERTEX_POINT ( 'NONE', #13730 ) ;
#5011=CARTESIAN_POINT ( 'NONE',  ( -0.3121994997597934973, 0.4069448477556333321, 1.747047244094488194 ) ) ;
#5014=CARTESIAN_POINT ( 'NONE',  ( -0.3765118517642104257, 0.000000000000000000, -3.100567304031763172 ) ) ;
#5020=CARTESIAN_POINT ( 'NONE',  ( 0.1078280746903977072, 0.3175540113612247972, 1.953740157480315043 ) ) ;
#5026=CARTESIAN_POINT ( 'NONE',  ( 0.5511811023622048555, 6.829619984160658046E-17, 0.9399606299212598381 ) ) ;
#5028=CARTESIAN_POINT ( 'NONE',  ( -0.05819755867303792046, 0.4417361510194100505, -1.934055118110236338 ) ) ;
#5036=CARTESIAN_POINT ( 'NONE',  ( -0.3574975638436101444, 0.000000000000000000, -3.115157480314960647 ) ) ;
#5040=DIRECTION ( 'NONE',  ( -0.000000000000000000, -0.000000000000000000, -1.000000000000000000 ) ) ;
#5047=CARTESIAN_POINT ( 'NONE',  ( 0.3242071728275122688, 0.4225965726692672564, 1.747047244094488194 ) ) ;
#5049=B_SPLINE_CURVE_WITH_KNOTS ( 'NONE', 3,
 ( #6035, #14526, #9835, #20998, #10245, #14671, #3321, #3608, #12097, #5467, #23129, #18433, #23275, #12238, #21138, #3904, #14377, #1643 ),
 .UNSPECIFIED., .F., .F.,
 ( 4, 2, 2, 2, 2, 2, 2, 2, 4 ),
 ( 0.5000000000000000000, 0.5625000000000000000, 0.6250000000000000000, 0.6875000000000000000, 0.7500000000000000000, 0.8125000000000000000, 0.8750000000000001110, 0.9375000000000001110, 1.000000000000000000 ),
 .UNSPECIFIED. ) ;
#5057=CARTESIAN_POINT ( 'NONE',  ( 0.3912931228432083297, 0.3001918266902350307, -1.569881889763779625 ) ) ;
#5060=CARTESIAN_POINT ( 'NONE',  ( -0.07214854559199535000, -0.5476281405333250918, 0.9399606299212598381 ) ) ;
#5072=VERTEX_POINT ( 'NONE', #7807 ) ;
#5076=CARTESIAN_POINT ( 'NONE',  ( -0.03001016326913665336, -0.4585215200179055817, -1.928289503579156516 ) ) ;
#5078=CARTESIAN_POINT ( 'NONE',  ( -0.07874015748031511219, 0.1968503937007874127, -3.548228346456693050 ) ) ;
#5099=CARTESIAN_POINT ( 'NONE',  ( 0.09522041251245175197, 0.3002250111098912488, -3.573961723184375661 ) ) ;
#5100=CARTESIAN_POINT ( 'NONE',  ( 0.3121994997578272368, 0.4069448477569235778, -1.550196850393700920 ) ) ;
#5101=CARTESIAN_POINT ( 'NONE',  ( -0.2297883689023087483, 0.3979194638820583441, -1.928289503579160513 ) ) ;
#5104=CARTESIAN_POINT ( 'NONE',  ( 0.3362148458988418187, -0.4382482975805321312, 0.9202755905511811330 ) ) ;
#5126=CARTESIAN_POINT ( 'NONE',  ( 0.2991932138496286586, -0.3411003281197161341, -1.934055118110236338 ) ) ;
#5129=CARTESIAN_POINT ( 'NONE',  ( 0.09524629980714841015, 0.3002167689318728239, -3.247000705324971648 ) ) ;
#5134=CARTESIAN_POINT ( 'NONE',  ( -0.3534612032199798692, -0.2712680014832878905, -1.934055118110236560 ) ) ;
#5135=CARTESIAN_POINT ( 'NONE',  ( -0.1213180142433854664, 0.3572819248074437515, -3.100567304031767168 ) ) ;
#5140=CARTESIAN_POINT ( 'NONE',  ( -0.2796934465393772773, -0.3645739570812616681, -1.928289503579163178 ) ) ;
#5143=CONICAL_SURFACE ( 'NONE', #20951, 0.4724409448465559103, 0.7853981642948979491 ) ;
#5147=CARTESIAN_POINT ( 'NONE',  ( 0.09842519685039366473, 0.1968503937007873850, -3.456364829396326943 ) ) ;
#5149=CARTESIAN_POINT ( 'NONE',  ( -0.4600326175560703335, -0.2268096725222389642, 1.747047244094488194 ) ) ;
#5151=ORIENTED_EDGE ( 'NONE', *, *, #16475, .T. ) ;
#5153=CARTESIAN_POINT ( 'NONE',  ( -0.1651192144506347381, 0.3349073414798414139, -3.115157480314960647 ) ) ;
#5164=CARTESIAN_POINT ( 'NONE',  ( 0.3349573549949907414, 0.2938049579018708890, -1.934055118110236338 ) ) ;
#5178=CARTESIAN_POINT ( 'NONE',  ( -0.2341512108694376038, 0.2669480828848188603, 1.953740157480315043 ) ) ;
#5181=EDGE_CURVE ( 'NONE', #22055, #1806, #23436, .T. ) ;
#5185=CARTESIAN_POINT ( 'NONE',  ( -0.2663596103035606455, 0.4612490782034870396, 1.747047244094488194 ) ) ;
#5187=CARTESIAN_POINT ( 'NONE',  ( 0.2564944395515608710, 0.4441657790107836346, 1.766732283464566899 ) ) ;
#5199=CARTESIAN_POINT ( 'NONE',  ( 0.3252100150720242944, 0.3707612262533179215, -1.569881889763779625 ) ) ;
#5202=CARTESIAN_POINT ( 'NONE',  ( -0.4783323773986942751, -0.2762247810518927427, 0.9399606299212598381 ) ) ;
#5203=ORIENTED_EDGE ( 'NONE', *, *, #20343, .T. ) ;
#5208=LINE ( 'NONE', #13831, #24858 ) ;
#5216=CARTESIAN_POINT ( 'NONE',  ( 0.2904160862623607620, -0.1677079028045494191, 1.953740157480315043 ) ) ;
#5225=FACE_OUTER_BOUND ( 'NONE', #19319, .T. ) ;
#5227=EDGE_CURVE ( 'NONE', #21275, #20990, #3873, .T. ) ;
#5229=CARTESIAN_POINT ( 'NONE',  ( 0.000000000000000000, 0.000000000000000000, 0.000000000000000000 ) ) ;
#5240=VECTOR ( 'NONE', #27035, 39.37007874015748854 ) ;
#5243=CARTESIAN_POINT ( 'NONE',  ( 0.1896185148830507872, 0.3289909311256233870, -3.100567304031763172 ) ) ;
#5248=CARTESIAN_POINT ( 'NONE',  ( -0.1677079028045370956, -0.2904160862623674233, 1.973425196850393970 ) ) ;
#5250=CARTESIAN_POINT ( 'NONE',  ( -0.4069448477569480582, 0.3121994997578198539, -1.550196850393700920 ) ) ;
#5254=CARTESIAN_POINT ( 'NONE',  ( 0.3362148458988273303, 0.4382482975805419012, 0.9202755905511811330 ) ) ;
#5255=CYLINDRICAL_SURFACE ( 'NONE', #14837, 0.5905511811023621549 ) ;
#5260=AXIS2_PLACEMENT_3D ( 'NONE', #17991, #21328, #18151 ) ;
#5266=VERTEX_POINT ( 'NONE', #12140 ) ;
#5270=DIRECTION ( 'NONE',  ( -1.000000000000000000, 0.000000000000000000, 0.000000000000000000 ) ) ;
#5272=CARTESIAN_POINT ( 'NONE',  ( -0.3075317527319259558, 0.1775220790475501298, 1.953740157480314821 ) ) ;
#5274=CARTESIAN_POINT ( 'NONE',  ( -0.3599896729929590866, -0.2761764805255594313, -1.934055118110236338 ) ) ;
#5277=CARTESIAN_POINT ( 'NONE',  ( -0.01298392085634582534, 0.3147567063785114416, -3.174859699051844064 ) ) ;
#5284=CARTESIAN_POINT ( 'NONE',  ( 0.1886891683788910479, -0.3267488823401750730, -3.100567304031762284 ) ) ;
#5287=VERTEX_POINT ( 'NONE', #22741 ) ;
#5288=CARTESIAN_POINT ( 'NONE',  ( -0.4498374011142775575, 0.05926487674658489219, -1.934055118110236338 ) ) ;
#5297=CARTESIAN_POINT ( 'NONE',  ( -0.03349795313264326141, 0.5118110236220472231, 1.747047244094488194 ) ) ;
#5302=CARTESIAN_POINT ( 'NONE',  ( -0.3267488823401750730, -0.1886891683788910756, -3.100567304031762284 ) ) ;
#5306=CARTESIAN_POINT ( 'NONE',  ( -0.01288382760289888754, 0.2165354330708661457, -3.646653543307086576 ) ) ;
#5308=ORIENTED_EDGE ( 'NONE', *, *, #15428, .F. ) ;
#5309=CARTESIAN_POINT ( 'NONE',  ( 0.2564173815262089096, 0.4442189740295122147, -1.550196850393701364 ) ) ;
#5313=CARTESIAN_POINT ( 'NONE',  ( 0.1970259548082060608, 0.3996230174612934172, -1.934055118110236338 ) ) ;
#5321=CARTESIAN_POINT ( 'NONE',  ( 0.000000000000000000, 0.000000000000000000, 1.953740157480315043 ) ) ;
#5330=CARTESIAN_POINT ( 'NONE',  ( -0.1775730735577452091, -0.3074993854542726335, 1.953740157480315043 ) ) ;
#5335=CARTESIAN_POINT ( 'NONE',  ( -0.5043504886477528926, -0.1712563538833036247, 1.747047244094488194 ) ) ;
#5336=CARTESIAN_POINT ( 'NONE',  ( -0.3121994997598287469, 0.4069448477556107946, 1.766732283464566899 ) ) ;
#5338=ORIENTED_EDGE ( 'NONE', *, *, #24560, .T. ) ;
#5344=CARTESIAN_POINT ( 'NONE',  ( -0.3996230174612752095, 0.1970259548082017587, -1.934055118110236338 ) ) ;
#5346=CARTESIAN_POINT ( 'NONE',  ( 0.3346456692913385988, 0.000000000000000000, 1.973425196850393970 ) ) ;
#5349=CARTESIAN_POINT ( 'NONE',  ( 0.4669911931914907388, -0.1585706980422228185, -1.569881889763779625 ) ) ;
#5351=ORIENTED_EDGE ( 'NONE', *, *, #9973, .F. ) ;
#5367=CARTESIAN_POINT ( 'NONE',  ( -0.2211428102655905170, 0.2521176338356723168, 1.953740157480315043 ) ) ;
#5368=UNCERTAINTY_MEASURE_WITH_UNIT (LENGTH_MEASURE( 1.000000000000000082E-05 ), #4839, 'distance_accuracy_value', 'NONE') ;
#5374=AXIS2_PLACEMENT_3D ( 'NONE', #16718, #2019, #27604 ) ;
#5386=CARTESIAN_POINT ( 'NONE',  ( -0.07870736599817637624, 0.1968503937007873850, -3.608715228723573976 ) ) ;
#5394=ADVANCED_FACE ( 'NONE', ( #964 ), #8509, .T. ) ;
#5398=CARTESIAN_POINT ( 'NONE',  ( 0.08676778863010990717, 0.3239425792934408910, 1.973425196850393970 ) ) ;
#5399=CARTESIAN_POINT ( 'NONE',  ( 0.3252100150720381722, -0.3707612262533039327, -1.550196850393700920 ) ) ;
#5403=CARTESIAN_POINT ( 'NONE',  ( -0.5476281405333195407, -0.07214854559197286799, 0.9202755905511811330 ) ) ;
#5404=DIRECTION ( 'NONE',  ( 1.000000000000000000, 0.000000000000000000, 0.000000000000000000 ) ) ;
#5408=CARTESIAN_POINT ( 'NONE',  ( -0.1275996891957758561, 0.4763861460130329184, -1.569881889763779625 ) ) ;
#5422=CARTESIAN_POINT ( 'NONE',  ( -0.02325127328499143609, 0.3543292900372674303, 1.953740157480315043 ) ) ;
#5425=CARTESIAN_POINT ( 'NONE',  ( -0.4296318976989931815, -0.1458850421962362698, -1.934055118110236338 ) ) ;
#5434=EDGE_LOOP ( 'NONE', ( #1497, #47, #6439, #12 ) ) ;
#5439=CARTESIAN_POINT ( 'NONE',  ( -0.2296683860596777926, -0.2993674444872276297, -3.100567304031764060 ) ) ;
#5440=CARTESIAN_POINT ( 'NONE',  ( -0.3460488714339713390, -0.09275962632023325438, -3.115157480314960647 ) ) ;
#5443=CARTESIAN_POINT ( 'NONE',  ( -0.2991932138496531390, 0.3411003281196664516, -1.934055118110236338 ) ) ;
#5450=CARTESIAN_POINT ( 'NONE',  ( 0.5043504886477625515, 0.1712563538832952981, 1.747047244094488194 ) ) ;
#5454=CARTESIAN_POINT ( 'NONE',  ( 0.3572819248074489140, -0.1213180142433802344, -3.100567304031756066 ) ) ;
#5457=CARTESIAN_POINT ( 'NONE',  ( 0.2938622683360631593, 0.000000000000000000, -3.745078740157480546 ) ) ;
#5467=CARTESIAN_POINT ( 'NONE',  ( -0.07214943758244271588, -0.5511811023622046335, 0.9202755905511812440 ) ) ;
#5468=CARTESIAN_POINT ( 'NONE',  ( 0.3259357382551449356, 0.08759279594700336569, 1.973425196850393970 ) ) ;
#5480=ORIENTED_EDGE ( 'NONE', *, *, #1724, .T. ) ;
#5483=CARTESIAN_POINT ( 'NONE',  ( 0.4600326175560532915, -0.2268096725222599475, 1.747047244094488194 ) ) ;
#5485=CARTESIAN_POINT ( 'NONE',  ( -0.07874015748031502893, 0.1968503937007874127, -3.272637795275590733 ) ) ;
#5486=B_SPLINE_CURVE_WITH_KNOTS ( 'NONE', 3,
 ( #9797, #13752, #15872, #5129, #20252, #914, #1196, #14193, #22795, #3419, #16021, #12057, #24619, #22517, #5277, #20676, #13898, #1056, #25186, #10629, #21243, #5714, #27747, #8246, #20812, #27318 ),
 .UNSPECIFIED., .F., .F.,
 ( 4, 2, 2, 2, 2, 2, 2, 2, 2, 2, 2, 2, 4 ),
 ( -0.006894309973022127655, -0.006402040495999860442, -0.005909771018977594097, -0.004925232064933059671, -0.003940693110888525245, -0.003448423633866250226, -0.002956154156843975207, -0.002463884679821699321, -0.001971615202799424302, -0.0009870762487548898761, -2.537294710355450511E-06, 0.0004897321823118935477, 0.0009820016593341408112 ),
 .UNSPECIFIED. ) ;
#5487=CARTESIAN_POINT ( 'NONE',  ( 0.1327036767659691974, 0.4954415918531168139, 1.747047244094488194 ) ) ;
#5500=CARTESIAN_POINT ( 'NONE',  ( 0.4669911931914765835, 0.1585706980422571244, -1.569881889763779625 ) ) ;
#5503=ORIENTED_EDGE ( 'NONE', *, *, #23744, .F. ) ;
#5516=CARTESIAN_POINT ( 'NONE',  ( -0.4921259842519685179, 0.06441914069860968373, -1.569881889763779625 ) ) ;
#5529=CARTESIAN_POINT ( 'NONE',  ( 0.07874015747999514592, 0.1968503937007873850, -3.558537267005753346 ) ) ;
#5535=CARTESIAN_POINT ( 'NONE',  ( 0.3289909311256232205, 0.1896185148830506484, -3.100567304031764060 ) ) ;
#5539=CARTESIAN_POINT ( 'NONE',  ( -0.3324885138898245329, -0.04380447413658584976, 1.973425196850393970 ) ) ;
#5547=CARTESIAN_POINT ( 'NONE',  ( 0.4763861460130340286, 0.1275996891957706103, -1.569881889763779625 ) ) ;
#5550=CARTESIAN_POINT ( 'NONE',  ( -0.3937007874015748254, 4.821444091131312140E-17, -3.036417322828325105 ) ) ;
#5551=LINE ( 'NONE', #27693, #25826 ) ;
#5553=FACE_OUTER_BOUND ( 'NONE', #27528, .T. ) ;
#5562=CARTESIAN_POINT ( 'NONE',  ( -0.04632226222404308563, 0.3520598332080951964, 1.953740157480315043 ) ) ;
#5569=CARTESIAN_POINT ( 'NONE',  ( 0.07874015748031495954, 0.1968503937007874127, -3.364501312335958172 ) ) ;
#5577=CARTESIAN_POINT ( 'NONE',  ( 0.3460530745557667820, -0.09275304139126368252, -3.115157480314960647 ) ) ;
#5579=CARTESIAN_POINT ( 'NONE',  ( 0.1152775731716972618, -0.4303822302053990634, -1.934055118110236338 ) ) ;
#5583=CARTESIAN_POINT ( 'NONE',  ( 0.07874015748031495954, 0.1968503937007873850, -3.548228346456692162 ) ) ;
#5585=CARTESIAN_POINT ( 'NONE',  ( -0.4612490782034865955, 0.2663596103035612561, 1.747047244094488194 ) ) ;
#5588=VERTEX_POINT ( 'NONE', #22708 ) ;
#5591=CARTESIAN_POINT ( 'NONE',  ( -0.3644697409450258219, -0.09762295995070061072, -3.100567304031765836 ) ) ;
#5597=PLANE ( 'NONE',  #8701 ) ;
#5600=CARTESIAN_POINT ( 'NONE',  ( 0.2712027394948776093, -0.3535065162672919037, -1.934055118110236338 ) ) ;
#5607=CARTESIAN_POINT ( 'NONE',  ( 0.2362439534887394721, -0.2693339498142455213, -3.115157480314960647 ) ) ;
#5613=CARTESIAN_POINT ( 'NONE',  ( 0.04380501567505449417, -0.3346456692913384878, 1.973425196850393970 ) ) ;
#5614=CONICAL_SURFACE ( 'NONE', #21405, 0.5511811023268710086, 0.7853981642949031672 ) ;
#5619=ORIENTED_EDGE ( 'NONE', *, *, #12525, .T. ) ;
#5623=CARTESIAN_POINT ( 'NONE',  ( -0.4225965726692971769, 0.3242071728275127129, 1.747047244094488194 ) ) ;
#5626=CARTESIAN_POINT ( 'NONE',  ( -0.06699507805369578350, -0.5085118447801426633, 1.766732283464566899 ) ) ;
#5637=CARTESIAN_POINT ( 'NONE',  ( -0.2466292688015002954, -0.4270824798167766612, -1.569881889763779625 ) ) ;
#5640=ORIENTED_EDGE ( 'NONE', *, *, #4237, .F. ) ;
#5656=B_SPLINE_CURVE_WITH_KNOTS ( 'NONE', 2,
 ( #15649, #2499, #26097 ),
 .UNSPECIFIED., .F., .F.,
 ( 3, 3 ),
 ( 0.000000000000000000, 1.000000000000000000 ),
 .UNSPECIFIED. ) ;
#5670=CARTESIAN_POINT ( 'NONE',  ( 0.08600259748440709784, 0.2165354330708661457, -3.597797143241304951 ) ) ;
#5687=CARTESIAN_POINT ( 'NONE',  ( 0.3382184156749452608, -0.3855916753034395184, -1.550196850393700920 ) ) ;
#5690=CARTESIAN_POINT ( 'NONE',  ( 0.3387265385688508212, 0.4407612517155324316, 0.9202755905511812440 ) ) ;
#5691=CARTESIAN_POINT ( 'NONE',  ( -0.5511811023622048555, 0.000000000000000000, 0.9399606299212598381 ) ) ;
#5693=EDGE_CURVE ( 'NONE', #1064, #23265, #21674, .T. ) ;
#5701=CARTESIAN_POINT ( 'NONE',  ( -0.3511586785142654654, 0.4004922687717341612, 1.747047244094488194 ) ) ;
#5704=EDGE_LOOP ( 'NONE', ( #1264, #5640, #5203, #4178 ) ) ;
#5714=CARTESIAN_POINT ( 'NONE',  ( -0.09333834261715735769, 0.3008238710200430988, -3.240734708634343875 ) ) ;
#5720=LINE ( 'NONE', #2322, #1854 ) ;
#5724=CARTESIAN_POINT ( 'NONE',  ( -0.3213059197594588245, -0.1584813376851955946, -3.115157480314960647 ) ) ;
#5728=CARTESIAN_POINT ( 'NONE',  ( 0.2712027394948692827, 0.3535065162672724748, -1.934055118110236338 ) ) ;
#5733=CARTESIAN_POINT ( 'NONE',  ( 0.09842519685039370636, 0.2165354330708661457, -3.548228346456692162 ) ) ;
#5735=CARTESIAN_POINT ( 'NONE',  ( -0.4004221243553298115, -0.3512268162760094348, 1.747047244094488194 ) ) ;
#5740=CARTESIAN_POINT ( 'NONE',  ( -0.1213180142433854664, 0.3572819248074437515, -3.100567304031767168 ) ) ;
#5743=B_SPLINE_SURFACE_WITH_KNOTS ( 'NONE', 2, 3, ( 
 ( #5346, #18605, #20461, #14107, #25685, #27531, #3788, #12955, #12407, #14556, #27810, #8175, #4214, #19318, #8444, #10702, #14834, #10416, #12549, #16788, #17204, #19179, #12679, #18889, #25401, #8041, #6065, #4075, #23714, #21022, #16935, #23154, #21308, #23445, #4350, #21451, #1668, #25258, #12819, #6470, #14697, #2090, #23304, #3932, #25545, #1808, #1945, #18753, #15105, #10276, #10556, #21166, #1529, #19034, #8586, #17067, #10137, #27669, #23580, #8317, #6336, #6205, #5921, #21, #14966, #25823 ),
 ( #27388, #16649, #2495, #26357, #2351, #8722, #26487, #8854, #283, #15513, #19873, #9117, #13498, #5020, #7021, #17865, #11116, #21584, #4887, #10843, #17736, #6753, #22125, #15644, #19608, #23852, #19457, #4490, #6612, #526, #26094, #24243, #11387, #2755, #20005, #6884, #19736, #13233, #15386, #9244, #11252, #4745, #10982, #23973, #17344, #21857, #24112, #13097, #405, #8988, #25960, #17612, #26226, #21993, #656, #2626, #7153, #15775, #15238, #24377, #21722, #26774, #7422, #27070, #26629, #14223 ),
 ( #23406, #27349, #1768, #4040, #10734, #18847, #21127, #27773, #6021, #14657, #14513, #20983, #5745, #12511, #1490, #12646, #4177, #17035, #17169, #25508, #8550, #23543, #14360, #10102, #25214, #21410, #5886, #3890, #21274, #8000, #10380, #1909, #22974, #27490, #19000, #8413, #23261, #27633, #23115, #1629, #3596, #8278, #18713, #10520, #12782, #25646, #12225, #20840, #3744, #16898, #16603, #14800, #19140, #12365, #6300, #10234, #8138, #14934, #19283, #16747, #2048, #25359, #13064, #13193, #26058, #8952 ) ),
 .UNSPECIFIED., .F., .T., .F.,
 ( 3, 3 ),
 ( 4, 2, 2, 2, 2, 2, 2, 2, 2, 2, 2, 2, 2, 2, 2, 2, 2, 2, 2, 2, 2, 2, 2, 2, 2, 2, 2, 2, 2, 2, 2, 2, 4 ),
 ( 0.000000000000000000, 1.000000000000000000 ),
 ( 0.000000000000000000, 0.1963495408493620697, 0.3926990816987241395, 0.5890486225480862092, 0.7853981633974482790, 0.9817477042468103487, 1.178097245096172418, 1.374446785945534488, 1.570796326794896558, 1.767145867644258628, 1.963495408493620697, 2.159844949342982545, 2.356194490192344837, 2.552544031041707129, 2.748893571891068976, 2.945243112740430824, 3.141592653589793116, 3.337942194439155408, 3.534291735288517255, 3.730641276137879103, 3.926990816987241395, 4.123340357836603687, 4.319689898685965090, 4.516039439535327382, 4.712388980384689674, 4.908738521234051966, 5.105088062083414258, 5.301437602932775661, 5.497787143782137953, 5.694136684631500245, 5.890486225480861648, 6.086835766330223940, 6.283185307179586232 ),
 .UNSPECIFIED. ) ;
#5745=CARTESIAN_POINT ( 'NONE',  ( 0.1570220809524471017, 0.3184841198566427112, 1.953740157480315043 ) ) ;
#5749=CARTESIAN_POINT ( 'NONE',  ( -0.1480156394741914683, 0.5526079293737398146, 0.9399606299212598381 ) ) ;
#5755=CARTESIAN_POINT ( 'NONE',  ( -0.3102476824511484210, -0.1791601451668926870, -3.115157480314960647 ) ) ;
#5773=CARTESIAN_POINT ( 'NONE',  ( -0.4856708409200654608, 0.1649135259617025839, 1.766732283464566899 ) ) ;
#5777=ORIENTED_EDGE ( 'NONE', *, *, #3202, .F. ) ;
#5785=CARTESIAN_POINT ( 'NONE',  ( 0.03220957031753916844, -0.4921259842519685179, -1.550196850393700920 ) ) ;
#5794=EDGE_CURVE ( 'NONE', #26373, #18491, #17329, .T. ) ;
#5812=LINE ( 'NONE', #14291, #15302 ) ;
#5829=VERTEX_POINT ( 'NONE', #10577 ) ;
#5830=CARTESIAN_POINT ( 'NONE',  ( 0.02190250779246093876, -0.3346456692913385433, 1.973425196850393970 ) ) ;
#5832=CARTESIAN_POINT ( 'NONE',  ( 0.2564944395535923571, -0.4441657790094409863, -1.550196850393700920 ) ) ;
#5835=CARTESIAN_POINT ( 'NONE',  ( 0.3642352168757231889, -0.4152525734085952269, 0.9399606299212598381 ) ) ;
#5848=CARTESIAN_POINT ( 'NONE',  ( 0.5280876769849813801, -0.06947563356185804118, 1.747047244094488194 ) ) ;
#5860=CARTESIAN_POINT ( 'NONE',  ( -0.2938622683360632148, 3.727965067992227128E-17, -3.745078740157480546 ) ) ;
#5861=AXIS2_PLACEMENT_3D ( 'NONE', #7438, #16067, #13946 ) ;
#5864=CARTESIAN_POINT ( 'NONE',  ( 0.1584813376851776368, -0.3213059197594625993, -3.115157480314961980 ) ) ;
#5866=CARTESIAN_POINT ( 'NONE',  ( 0.3001918266902144361, -0.3912931228432220410, -1.569881889763779625 ) ) ;
#5868=CARTESIAN_POINT ( 'NONE',  ( -0.3858397471888894703, -0.2228126397719936702, -1.934055118110236338 ) ) ;
#5876=CARTESIAN_POINT ( 'NONE',  ( 0.5085118447801502128, -0.06699507805371243685, 1.747047244094488194 ) ) ;
#5880=CARTESIAN_POINT ( 'NONE',  ( 0.2296683860596781812, -0.2993674444872274631, -3.100567304031764060 ) ) ;
#5886=CARTESIAN_POINT ( 'NONE',  ( -0.2817310484609166221, 0.2161381151963042424, 1.953740157480315043 ) ) ;
#5892=CARTESIAN_POINT ( 'NONE',  ( 0.3482225189666449672, 0.4539000224941344697, 0.9399606299212598381 ) ) ;
#5897=CARTESIAN_POINT ( 'NONE',  ( -0.09269288654274109029, 0.3460635936744927421, -3.115157480314960647 ) ) ;
#5899=DIRECTION ( 'NONE',  ( 1.000000000000000000, 0.000000000000000000, 0.000000000000000000 ) ) ;
#5904=EDGE_LOOP ( 'NONE', ( #8750, #17527, #17002, #26771 ) ) ;
#5905=CARTESIAN_POINT ( 'NONE',  ( -0.1481199686337219545, 0.5525886237725313732, 0.9399606299212598381 ) ) ;
#5912=CARTESIAN_POINT ( 'NONE',  ( 0.4069448477555986377, -0.3121994997598466770, 1.766732283464566899 ) ) ;
#5921=CARTESIAN_POINT ( 'NONE',  ( 0.3239425792934409465, -0.08676778863010950471, 1.973425196850393970 ) ) ;
#5925=CARTESIAN_POINT ( 'NONE',  ( -0.2180862235769588653, -0.4423390553432484107, -1.550196850393700920 ) ) ;
#5949=ORIENTED_EDGE ( 'NONE', *, *, #9973, .T. ) ;
#5956=CARTESIAN_POINT ( 'NONE',  ( -0.3642352168757148068, 0.4152525734086684461, 0.9202755905511811330 ) ) ;
#5959=B_SPLINE_CURVE_WITH_KNOTS ( 'NONE', 3,
 ( #11262, #22003, #948, #24119, #2763, #9538, #11395, #26495, #22268, #7161, #15913, #4755, #535, #9126, #18140, #26784, #17745, #24385 ),
 .UNSPECIFIED., .F., .F.,
 ( 4, 2, 2, 2, 2, 2, 2, 2, 4 ),
 ( 0.000000000000000000, 0.1250000000000000000, 0.2500000000000000000, 0.3750000000000000000, 0.5000000000000000000, 0.6250000000000000000, 0.7500000000000000000, 0.8750000000000000000, 1.000000000000000000 ),
 .UNSPECIFIED. ) ;
#5970=CARTESIAN_POINT ( 'NONE',  ( 0.02190250779246040100, 0.3346456692913385988, 1.953740157480315043 ) ) ;
#5971=CARTESIAN_POINT ( 'NONE',  ( -0.5085118447796470598, -0.06699507805605113553, -1.550196850393700920 ) ) ;
#5973=CARTESIAN_POINT ( 'NONE',  ( -0.4300830224589641260, 0.3772436174784328244, 0.9399606299212598381 ) ) ;
#5977=CARTESIAN_POINT ( 'NONE',  ( -0.09275248786873620255, 0.3460502918090236357, -3.115157480314960647 ) ) ;
#5980=CARTESIAN_POINT ( 'NONE',  ( 0.4613045817969895213, 0.2662790972925014876, 1.747047244094487972 ) ) ;
#5985=CARTESIAN_POINT ( 'NONE',  ( -0.3707612262533164782, -0.3252100150720257377, -1.550196850393700920 ) ) ;
#6003=EDGE_LOOP ( 'NONE', ( #20167, #26088, #12946, #27847 ) ) ;
#6005=CARTESIAN_POINT ( 'NONE',  ( 0.1173917140416251143, -0.4382752542995838052, -1.934055118110236338 ) ) ;
#6006=CARTESIAN_POINT ( 'NONE',  ( 0.4351030398461776527, -0.1477428134820240602, -1.928289503579159625 ) ) ;
#6007=CONICAL_SURFACE ( 'NONE', #24934, 0.3726024258163779246, 0.2617993874999969828 ) ;
#6011=CARTESIAN_POINT ( 'NONE',  ( 0.3574975638436101444, 4.268512490100411279E-17, -3.115157480314960647 ) ) ;
#6012=CARTESIAN_POINT ( 'NONE',  ( -0.5314960629921260393, -0.03478633594543723700, 1.747047244094488194 ) ) ;
#6016=CARTESIAN_POINT ( 'NONE',  ( -0.09842519685039370636, 0.2165354330708661457, -3.456364829396325611 ) ) ;
#6021=CARTESIAN_POINT ( 'NONE',  ( 0.2669480828848126985, 0.2341512108694336625, 1.953740157480315043 ) ) ;
#6027=CARTESIAN_POINT ( 'NONE',  ( -0.4300830224589284878, -0.3772436174784035146, 0.9399606299212598381 ) ) ;
#6034=CARTESIAN_POINT ( 'NONE',  ( 0.2180698645301770711, -0.2842490391651530390, -3.115157480314960647 ) ) ;
#6035=CARTESIAN_POINT ( 'NONE',  ( 0.5511811023622047445, 3.414809992080329023E-17, 0.9202755905511811330 ) ) ;
#6037=CARTESIAN_POINT ( 'NONE',  ( -2.685748425196850164E-17, 0.000000000000000000, -1.934055118110236338 ) ) ;
#6043=CARTESIAN_POINT ( 'NONE',  ( -0.07870736637777368816, 0.2165354330708661734, -3.212150913388296392 ) ) ;
#6047=ORIENTED_EDGE ( 'NONE', *, *, #11966, .T. ) ;
#6054=CARTESIAN_POINT ( 'NONE',  ( 0.06957181182499888594, -0.5280699926562973934, 1.747047244094488194 ) ) ;
#6057=CARTESIAN_POINT ( 'NONE',  ( 0.06699507805370044644, -0.5085118447801416641, 1.766732283464566899 ) ) ;
#6060=CARTESIAN_POINT ( 'NONE',  ( 0.1584254766472199816, -0.3213305936751578717, -3.115157480314960647 ) ) ;
#6065=CARTESIAN_POINT ( 'NONE',  ( -0.2660793235464223860, 0.2041304421298429095, 1.973425196850393970 ) ) ;
#6067=CARTESIAN_POINT ( 'NONE',  ( 0.3912931228432192099, -0.3001918266902123267, -1.550196850393700920 ) ) ;
#6075=DIRECTION ( 'NONE',  ( -0.2588190448135617161, 3.169619147893037226E-17, 0.9659258263664945998 ) ) ;
#6077=DIRECTION ( 'NONE',  ( -0.000000000000000000, -0.000000000000000000, 1.000000000000000000 ) ) ;
#6079=ORIENTED_EDGE ( 'NONE', *, *, #22757, .F. ) ;
#6086=B_SPLINE_CURVE_WITH_KNOTS ( 'NONE', 3,
 ( #15841, #9468, #21212, #3383, #12158, #25156, #23056, #3831, #25867, #22271, #6515, #10888, #13374, #22000, #11258, #26364, #6527, #4407, #8637, #10899, #481, #12905, #15597, #10176, #7658, #22915, #23063, #25307, #3535, #18794, #3388, #8085, #22762, #14600 ),
 .UNSPECIFIED., .F., .F.,
 ( 4, 2, 2, 2, 2, 2, 2, 2, 2, 2, 2, 2, 2, 2, 2, 2, 4 ),
 ( 0.000000000000000000, 0.03124999999999995837, 0.06249999999999991673, 0.09374999999999987510, 0.1249999999999998335, 0.1562499999999997780, 0.1874999999999997780, 0.2187499999999997502, 0.2499999999999997780, 0.2812499999999997780, 0.3124999999999997780, 0.3437499999999998335, 0.3749999999999998335, 0.4062499999999998335, 0.4374999999999998890, 0.4687500000000000000, 0.5000000000000000000 ),
 .UNSPECIFIED. ) ;
#6088=CARTESIAN_POINT ( 'NONE',  ( -0.2309201403895327909, 0.4006498629591503935, -1.928289503579156960 ) ) ;
#6101=CARTESIAN_POINT ( 'NONE',  ( -0.4856708409191258236, -0.1649135259639268325, -1.550196850393700920 ) ) ;
#6104=CARTESIAN_POINT ( 'NONE',  ( -0.2442565704126104242, 0.4954197419817720216, 0.9202755905511811330 ) ) ;
#6117=CARTESIAN_POINT ( 'NONE',  ( 0.4600326175569787179, -0.2268096725200276775, -1.550196850393700920 ) ) ;
#6121=CARTESIAN_POINT ( 'NONE',  ( -0.5708661417322835607, 0.03736310157554031952, 0.9399606299212598381 ) ) ;
#6131=CARTESIAN_POINT ( 'NONE',  ( 0.3121994997578124154, -0.4069448477569433953, -1.550196850393700920 ) ) ;
#6137=CARTESIAN_POINT ( 'NONE',  ( -0.2356240016490478428, -0.4776900717920959383, 1.747047244094487972 ) ) ;
#6138=CARTESIAN_POINT ( 'NONE',  ( 0.3381532161288250404, 0.3856588814719275615, -1.550196850393701364 ) ) ;
#6142=B_SPLINE_CURVE_WITH_KNOTS ( 'NONE', 2,
 ( #24388, #26497, #13510 ),
 .UNSPECIFIED., .F., .F.,
 ( 3, 3 ),
 ( 0.000000000000000000, 1.000000000000000000 ),
 .UNSPECIFIED. ) ;
#6157=CARTESIAN_POINT ( 'NONE',  ( -0.3454440660767217341, 0.3030032861725395210, -1.928289503579147635 ) ) ;
#6162=ORIENTED_EDGE ( 'NONE', *, *, #24932, .F. ) ;
#6166=CARTESIAN_POINT ( 'NONE',  ( 0.06957181182499888594, -0.5280699926562973934, 1.747047244094488194 ) ) ;
#6172=CARTESIAN_POINT ( 'NONE',  ( -0.3995939286814633173, 0.1970998888479515987, -1.934055118110236338 ) ) ;
#6182=CARTESIAN_POINT ( 'NONE',  ( -0.2362439534887433856, 0.2693339498142315325, -3.115157480314960647 ) ) ;
#6197=ORIENTED_EDGE ( 'NONE', *, *, #12888, .F. ) ;
#6200=CARTESIAN_POINT ( 'NONE',  ( 0.2180698645301770711, -0.2842490391651530390, -3.115157480314960647 ) ) ;
#6203=EDGE_CURVE ( 'NONE', #14125, #21357, #24662, .T. ) ;
#6205=CARTESIAN_POINT ( 'NONE',  ( 0.3175540113612324578, -0.1078280746903944320, 1.973425196850393970 ) ) ;
#6208=EDGE_LOOP ( 'NONE', ( #23855, #3827, #18468, #9517 ) ) ;
#6209=CARTESIAN_POINT ( 'NONE',  ( 0.1585706980422246781, 0.4669911931914895176, -1.550196850393700920 ) ) ;
#6224=CARTESIAN_POINT ( 'NONE',  ( -0.09842519685039377575, 0.2165354330708661457, -3.272637795275590733 ) ) ;
#6227=ORIENTED_EDGE ( 'NONE', *, *, #22757, .T. ) ;
#6231=ADVANCED_FACE ( 'NONE', ( #27558, #6358 ), #16817, .T. ) ;
#6233=CARTESIAN_POINT ( 'NONE',  ( -0.4600326175569940945, -0.2268096725200247077, -1.550196850393700920 ) ) ;
#6236=ADVANCED_FACE ( 'NONE', ( #8470 ), #14991, .T. ) ;
#6237=CARTESIAN_POINT ( 'NONE',  ( 0.5230301363771324707, 0.1775991818008611500, 0.9202755905511811330 ) ) ;
#6239=ADVANCED_FACE ( 'NONE', ( #27085 ), #18437, .T. ) ;
#6250=CARTESIAN_POINT ( 'NONE',  ( 0.3346456692913385988, 0.000000000000000000, 1.953740157480315043 ) ) ;
#6254=CARTESIAN_POINT ( 'NONE',  ( -0.5476281405333571772, -0.07214854559198842499, 0.9399606299212598381 ) ) ;
#6261=CARTESIAN_POINT ( 'NONE',  ( 0.5118110236220473341, 0.03349795313024165472, -1.550196850393700920 ) ) ;
#6262=CARTESIAN_POINT ( 'NONE',  ( 0.3771675965698876309, -0.4301570366551953351, 0.9399606299212600602 ) ) ;
#6266=CARTESIAN_POINT ( 'NONE',  ( -0.5043892184459256578, -0.1711665596935614542, 1.747047244094487972 ) ) ;
#6267=EDGE_CURVE ( 'NONE', #12664, #22294, #20259, .T. ) ;
#6268=CARTESIAN_POINT ( 'NONE',  ( 0.06690352886846342995, 0.5085315017395506398, -1.550196850393700920 ) ) ;
#6283=CARTESIAN_POINT ( 'NONE',  ( 0.4069519308877018182, 0.2006393256663585589, -1.934055118110236338 ) ) ;
#6291=CARTESIAN_POINT ( 'NONE',  ( 0.1378076643338767004, -0.5144970376935934508, 1.747047244094488194 ) ) ;
#6296=DIRECTION ( 'NONE',  ( -0.000000000000000000, -0.000000000000000000, 1.000000000000000000 ) ) ;
#6297=CARTESIAN_POINT ( 'NONE',  ( -0.2227473777833936797, 0.3858850602362957072, -1.934055118110236338 ) ) ;
#6300=CARTESIAN_POINT ( 'NONE',  ( 0.1775730735577447927, -0.3074993854542728555, 1.953740157480315043 ) ) ;
#6304=CARTESIAN_POINT ( 'NONE',  ( -0.2529800193559321730, -0.5131133041954082374, 0.9399606299212598381 ) ) ;
#6305=AXIS2_PLACEMENT_3D ( 'NONE', #8029, #20731, #1376 ) ;
#6311=CARTESIAN_POINT ( 'NONE',  ( 0.1200583359873108324, 0.3535721684717922364, -3.115157480314960647 ) ) ;
#6316=CARTESIAN_POINT ( 'NONE',  ( 0.3935368318888682881, -0.3024344094364739832, -1.569881889763779625 ) ) ;
#6318=CARTESIAN_POINT ( 'NONE',  ( -0.4152525734086684461, 0.3642352168757148068, 0.9202755905511811330 ) ) ;
#6326=CARTESIAN_POINT ( 'NONE',  ( -0.4600326175560602304, -0.2268096725222347454, 1.766732283464566899 ) ) ;
#6330=CARTESIAN_POINT ( 'NONE',  ( 0.1584254766472226184, 0.3213305936751399972, -3.115157480314960647 ) ) ;
#6335=EDGE_CURVE ( 'NONE', #5588, #2791, #4042, .T. ) ;
#6336=CARTESIAN_POINT ( 'NONE',  ( 0.3007905576423843819, -0.1482986320106508549, 1.973425196850393970 ) ) ;
#6341=CARTESIAN_POINT ( 'NONE',  ( -0.3001918266901933974, 0.3912931228432126596, -1.550196850393700920 ) ) ;
#6349=CARTESIAN_POINT ( 'NONE',  ( -0.09842519685039370636, 0.2991866959364303802, -3.548228346456693050 ) ) ;
#6351=ORIENTED_EDGE ( 'NONE', *, *, #20587, .F. ) ;
#6356=CARTESIAN_POINT ( 'NONE',  ( 0.06441914069860958658, 0.4921259842519684624, -1.569881889763779625 ) ) ;
#6357=DIRECTION ( 'NONE',  ( -1.000000000000000000, 0.000000000000000000, 0.000000000000000000 ) ) ;
#6358=FACE_BOUND ( 'NONE', #9068, .T. ) ;
#6359=CARTESIAN_POINT ( 'NONE',  ( 0.07870736599821760715, 0.2165354330708661457, -3.212150913008740449 ) ) ;
#6365=VECTOR ( 'NONE', #2338, 39.37007874015748143 ) ;
#6368=CARTESIAN_POINT ( 'NONE',  ( 0.2442565704126475612, 0.4954197419817565895, 0.9202755905511811330 ) ) ;
#6386=CONICAL_SURFACE ( 'NONE', #27603, 0.5511811023268710086, 0.7853981642949031672 ) ;
#6391=CARTESIAN_POINT ( 'NONE',  ( 0.5511811023622048555, -0.03607471876262468430, 0.9399606299212598381 ) ) ;
#6396=CARTESIAN_POINT ( 'NONE',  ( -0.02345921195965510950, 0.3574961452116666161, -3.115157480314960647 ) ) ;
#6402=CARTESIAN_POINT ( 'NONE',  ( -0.4856708409191340392, 0.1649135259639384898, -1.550196850393700920 ) ) ;
#6417=CARTESIAN_POINT ( 'NONE',  ( -0.2180862235769436830, 0.4423390553432706707, -1.550196850393700920 ) ) ;
#6418=CARTESIAN_POINT ( 'NONE',  ( -0.3411003281197191872, -0.2991932138496762317, -1.934055118110236338 ) ) ;
#6428=ORIENTED_EDGE ( 'NONE', *, *, #16585, .F. ) ;
#6431=B_SPLINE_SURFACE_WITH_KNOTS ( 'NONE', 2, 3, ( 
 ( #3489, #10273, #24682, #10001, #18317, #5344, #7611, #13967, #27244, #22579, #20459, #925, #13769, #2034, #26932, #5028, #12089, #24516, #7571, #802, #13647, #5313, #14229, #24799, #22264, #5164, #1230, #13791, #11955, #22412, #2897, #18429, #3314, #9535, #1090, #18137, #9828, #27076, #22835, #7724, #24938, #20428, #5600, #3460, #20712, #1356, #3033, #16058, #13936, #22550, #18567, #3177, #9687, #11810, #2361, #12326, #27745, #4852, #15616, #19426, #6852, #17171, #21965, #21826, #25786, #22093 ),
 ( #26194, #2592, #19840, #9089, #10809, #6716, #21546, #17440, #17305, #25924, #15201, #23812, #15354, #13066, #23946, #4582, #18391, #14190, #14043, #22652, #22792, #3416, #13749, #20109, #9794, #9219, #13895, #11772, #17840, #26458, #7121, #15745, #11494, #22230, #766, #18093, #9646, #2856, #16018, #26886, #9356, #5126, #7393, #11918, #20249, #9498, #17961, #7250, #26599, #26738, #15869, #24761, #24474, #20537, #22372, #2994, #11627, #24616, #5274, #1052, #22514, #5425, #1194, #20554, #10086, #27477 ),
 ( #25204, #8122, #16728, #9667, #3878, #26905, #18694, #21111, #13733, #24063, #9339, #13453, #22355, #17945, #19822, #4697, #21952, #2577, #22076, #750, #2709, #896, #11341, #24332, #13592, #3693, #22814, #27054, #22669, #21670, #2300, #19548, #14785, #21254, #14643, #19122, #6006, #23245, #12496, #4694, #17568, #6975, #22072, #26180, #22349, #13320, #2703, #22209, #27017, #5076, #24993, #22460, #20344, #24492, #7007, #5140, #24228, #16035, #24632, #11788, #8603, #17224, #13483, #20421, #13638, #9527 ) ),
 .UNSPECIFIED., .F., .T., .F.,
 ( 3, 3 ),
 ( 4, 2, 2, 2, 2, 2, 2, 2, 2, 2, 2, 2, 2, 2, 2, 2, 2, 2, 2, 2, 2, 2, 2, 2, 2, 2, 2, 2, 2, 2, 2, 2, 4 ),
 ( 0.000000000000000000, 1.000000000000000000 ),
 ( 0.000000000000000000, 0.1963495408493620697, 0.3926990816987241395, 0.5890486225480862092, 0.7853981633974482790, 0.9817477042468103487, 1.178097245096172418, 1.374446785945534488, 1.570796326794896558, 1.767145867644258628, 1.963495408493620697, 2.159844949342982545, 2.356194490192344837, 2.552544031041707129, 2.748893571891068976, 2.945243112740430824, 3.141592653589793116, 3.337942194439155408, 3.534291735288517255, 3.730641276137879103, 3.926990816987241395, 4.123340357836603687, 4.319689898685965090, 4.516039439535327382, 4.712388980384689674, 4.908738521234051966, 5.105088062083414258, 5.301437602932775661, 5.497787143782137953, 5.694136684631500245, 5.890486225480861648, 6.086835766330223940, 6.283185307179586232 ),
 .UNSPECIFIED. ) ;
#6432=CARTESIAN_POINT ( 'NONE',  ( 0.3534612032199636600, 0.2712680014832398734, -1.934055118110236338 ) ) ;
#6439=ORIENTED_EDGE ( 'NONE', *, *, #18603, .F. ) ;
#6441=CARTESIAN_POINT ( 'NONE',  ( -0.2462256503456003442, -0.2807137536170363767, -3.115157480314960647 ) ) ;
#6442=CARTESIAN_POINT ( 'NONE',  ( -0.09842519685039370636, 0.2165354330708661457, -3.548228346456693050 ) ) ;
#6449=ADVANCED_FACE ( 'NONE', ( #4327 ), #25375, .T. ) ;
#6458=CARTESIAN_POINT ( 'NONE',  ( -0.1649135259617057203, -0.4856708409200641841, 1.766732283464566899 ) ) ;
#6460=CARTESIAN_POINT ( 'NONE',  ( -0.3855916753051391033, -0.3382184156731863900, 1.747047244094488194 ) ) ;
#6465=CARTESIAN_POINT ( 'NONE',  ( 0.02339816079119036787, -0.3574975638436101444, -3.115157480314960647 ) ) ;
#6470=CARTESIAN_POINT ( 'NONE',  ( -0.2660793235464258277, -0.2041304421298378857, 1.973425196850393970 ) ) ;
#6480=B_SPLINE_CURVE_WITH_KNOTS ( 'NONE', 3,
 ( #6349, #23458, #6482, #6626, #15117, #13246, #12690, #11126, #21320, #4086, #10568, #1960, #8457, #23865 ),
 .UNSPECIFIED., .F., .F.,
 ( 4, 2, 2, 2, 2, 2, 4 ),
 ( -0.006894311516889582540, -0.006402023259230029545, -0.005909735001570475682, -0.004925158486251331527, -0.003940581970932187372, -0.003448293713272615295, -0.002956005455613042350 ),
 .UNSPECIFIED. ) ;
#6482=CARTESIAN_POINT ( 'NONE',  ( -0.09777734206179262977, 0.2994020000292518247, -3.561217286890655309 ) ) ;
#6497=CARTESIAN_POINT ( 'NONE',  ( -0.02576258753919771077, 0.1968503937007873850, -3.176774343053085481 ) ) ;
#6506=AXIS2_PLACEMENT_3D ( 'NONE', #3472, #9981, #1509 ) ;
#6508=CARTESIAN_POINT ( 'NONE',  ( -0.5335524835332036142, 0.1429116519061177371, 0.9399606299212598381 ) ) ;
#6515=CARTESIAN_POINT ( 'NONE',  ( -0.3122765577857348207, -0.4068916527365984415, -1.550196850393700476 ) ) ;
#6517=AXIS2_PLACEMENT_3D ( 'NONE', #23769, #15021, #2411 ) ;
#6518=CARTESIAN_POINT ( 'NONE',  ( 0.07874015748031489015, 0.1968503937007874127, -3.272637795275590733 ) ) ;
#6526=CARTESIAN_POINT ( 'NONE',  ( 0.2529800193559378352, 0.5131133041953702678, 0.9399606299212598381 ) ) ;
#6527=CARTESIAN_POINT ( 'NONE',  ( -0.03359157810863924731, -0.5118096047256377457, -1.550196850393700920 ) ) ;
#6528=AXIS2_PLACEMENT_3D ( 'NONE', #21597, #6077, #16662 ) ;
#6535=CARTESIAN_POINT ( 'NONE',  ( 0.4600326175569787179, -0.2268096725200276775, -1.550196850393700920 ) ) ;
#6536=CARTESIAN_POINT ( 'NONE',  ( 0.5708661417322835607, 6.829619984160658046E-17, 0.9399606299212598381 ) ) ;
#6557=CARTESIAN_POINT ( 'NONE',  ( -0.06441834428466812479, 0.4889536969035060410, -1.550196850393700920 ) ) ;
#6559=CARTESIAN_POINT ( 'NONE',  ( 0.4382752542995623779, 0.1173917140416305405, -1.934055118110236338 ) ) ;
#6567=CARTESIAN_POINT ( 'NONE',  ( -0.2355331214654103611, -0.4777261797697372470, 1.747047244094488194 ) ) ;
#6581=B_SPLINE_CURVE_WITH_KNOTS ( 'NONE', 3,
 ( #9700, #22277, #2910, #15923, #11542, #18299, #20157, #11968, #816, #5613, #9404, #22848, #26944, #3474, #3326, #12102, #24528, #2033 ),
 .UNSPECIFIED., .F., .F.,
 ( 4, 2, 2, 2, 2, 2, 2, 2, 4 ),
 ( 0.5000000000000000000, 0.5625000000000000000, 0.6250000000000000000, 0.6875000000000000000, 0.7500000000000000000, 0.8125000000000000000, 0.8750000000000001110, 0.9375000000000001110, 1.000000000000000000 ),
 .UNSPECIFIED. ) ;
#6585=CARTESIAN_POINT ( 'NONE',  ( 0.2807137536170455361, -0.2462256503455606815, -3.115157480314960647 ) ) ;
#6588=CARTESIAN_POINT ( 'NONE',  ( -0.09842519685039387289, 0.2165354330708660902, -3.561112174596415159 ) ) ;
#6600=CARTESIAN_POINT ( 'NONE',  ( 0.3121994997598427912, 0.4069448477556012467, 1.766732283464566899 ) ) ;
#6601=CARTESIAN_POINT ( 'NONE',  ( -0.4856708409200505283, -0.1649135259617098836, 1.747047244094488194 ) ) ;
#6605=CARTESIAN_POINT ( 'NONE',  ( -0.3233561589688984661, 0.1867299569291787087, -3.115157480314960647 ) ) ;
#6612=CARTESIAN_POINT ( 'NONE',  ( -0.3007905576423956506, 0.1482986320106521871, 1.953740157480315043 ) ) ;
#6626=CARTESIAN_POINT ( 'NONE',  ( -0.09524605906741696881, 0.3002168457537168766, -3.573866392918775503 ) ) ;
#6648=LINE ( 'NONE', #2660, #17868 ) ;
#6652=CARTESIAN_POINT ( 'NONE',  ( -0.3362148458988027944, 0.4382482975805537806, 0.9399606299212598381 ) ) ;
#6669=CARTESIAN_POINT ( 'NONE',  ( 0.2529800193559499921, -0.5131133041954075713, 0.9399606299212598381 ) ) ;
#6694=CARTESIAN_POINT ( 'NONE',  ( 0.3001918266902269261, 0.3912931228431901776, -1.550196850393700920 ) ) ;
#6695=CARTESIAN_POINT ( 'NONE',  ( -0.06001958459474868862, 0.4555658499976078524, -1.928289503579158515 ) ) ;
#6716=CARTESIAN_POINT ( 'NONE',  ( -0.4069519308876554664, 0.2006393256663590030, -1.934055118110236338 ) ) ;
#6725=CARTESIAN_POINT ( 'NONE',  ( -0.3606853515406169275, 0.09660931395005029065, -3.115157480314960647 ) ) ;
#6733=AXIS2_PLACEMENT_3D ( 'NONE', #20426, #22686, #9024 ) ;
#6738=CARTESIAN_POINT ( 'NONE',  ( 0.4984899526255159308, 0.1339654526248287292, 1.766732283464566677 ) ) ;
#6743=CARTESIAN_POINT ( 'NONE',  ( -0.4856708409200499732, 0.1649135259616961724, 1.747047244094488194 ) ) ;
#6748=CARTESIAN_POINT ( 'NONE',  ( -0.09660931395005634137, -0.3606853515406420185, -3.115157480314960647 ) ) ;
#6753=CARTESIAN_POINT ( 'NONE',  ( -0.1482986320106466638, 0.3007905576423924310, 1.953740157480315043 ) ) ;
#6756=ORIENTED_EDGE ( 'NONE', *, *, #20212, .T. ) ;
#6767=CARTESIAN_POINT ( 'NONE',  ( -1.452994488188976472E-16, 0.5905905511811023745, -3.646653543307086576 ) ) ;
#6787=CARTESIAN_POINT ( 'NONE',  ( 0.5335524835332415838, 0.1429116519061139345, 0.9399606299212598381 ) ) ;
#6792=DIRECTION ( 'NONE',  ( -1.000000000000000000, 0.000000000000000000, 0.000000000000000000 ) ) ;
#6804=CARTESIAN_POINT ( 'NONE',  ( 0.3482225189666449672, 0.4539000224941344697, 0.9399606299212598381 ) ) ;
#6814=CARTESIAN_POINT ( 'NONE',  ( 0.03349795313024073878, -0.5118110236220473341, -1.550196850393700920 ) ) ;
#6830=CARTESIAN_POINT ( 'NONE',  ( -2.685748425196850164E-17, 0.000000000000000000, -1.934055118110236338 ) ) ;
#6831=CARTESIAN_POINT ( 'NONE',  ( -0.03001016326913665336, -0.4585215200179055817, -1.928289503579156516 ) ) ;
#6833=CARTESIAN_POINT ( 'NONE',  ( -0.5230301363771427958, 0.1775991818008358647, 0.9202755905511811330 ) ) ;
#6852=CARTESIAN_POINT ( 'NONE',  ( -0.3996230174612653285, -0.1970259548082108347, -1.934055118110236338 ) ) ;
#6858=AXIS2_PLACEMENT_3D ( 'NONE', #18789, #20783, #1425 ) ;
#6860=CARTESIAN_POINT ( 'NONE',  ( -0.3572819248074391996, 0.1213180142433954029, -3.100567304031768057 ) ) ;
#6870=CARTESIAN_POINT ( 'NONE',  ( 0.2577577458591218673, 0.4472135058506045424, 1.766732283464566899 ) ) ;
#6873=CARTESIAN_POINT ( 'NONE',  ( -0.1327036767659477978, -0.4954415918530775120, 1.747047244094488194 ) ) ;
#6880=CARTESIAN_POINT ( 'NONE',  ( 0.02438677169350735724, -0.3726024258163779246, -3.115157480314960647 ) ) ;
#6884=CARTESIAN_POINT ( 'NONE',  ( -0.3239425792934415571, -0.08676778863010886633, 1.953740157480315043 ) ) ;
#6894=EDGE_CURVE ( 'NONE', #1047, #1806, #21030, .T. ) ;
#6897=CARTESIAN_POINT ( 'NONE',  ( -0.5511811023268710086, 0.000000000000000000, 1.747047244094488194 ) ) ;
#6904=AXIS2_PLACEMENT_3D ( 'NONE', #26516, #15269, #13123 ) ;
#6912=CARTESIAN_POINT ( 'NONE',  ( 0.2268096725222374654, 0.4600326175560591202, 1.766732283464566899 ) ) ;
#6920=CARTESIAN_POINT ( 'NONE',  ( 0.09842519685039370636, 0.5905905511811023745, -3.272637795275590733 ) ) ;
#6925=CARTESIAN_POINT ( 'NONE',  ( -0.5476281405333195407, -0.07214854559197286799, 0.9202755905511811330 ) ) ;
#6945=CARTESIAN_POINT ( 'NONE',  ( -0.5708661417322835607, -0.03736310157554036115, 0.9399606299212598381 ) ) ;
#6946=CARTESIAN_POINT ( 'NONE',  ( 0.06699590632655393063, -0.5118110236220473341, 1.766732283464566677 ) ) ;
#6971=CARTESIAN_POINT ( 'NONE',  ( -0.06699507805604322519, 0.5085118447796660446, -1.550196850393700920 ) ) ;
#6973=CARTESIAN_POINT ( 'NONE',  ( 0.03001016326913580681, 0.4585215200179055817, -1.928289503579156516 ) ) ;
#6975=CARTESIAN_POINT ( 'NONE',  ( 0.3030032861724964444, -0.3454440660767522098, -1.928289503579156516 ) ) ;
#6976=CARTESIAN_POINT ( 'NONE',  ( -0.1775991818008739453, 0.5230301363771271417, 0.9202755905511811330 ) ) ;
#6999=CARTESIAN_POINT ( 'NONE',  ( 0.3644697409450263215, 0.09762295995069791843, -3.100567304031765836 ) ) ;
#7004=CARTESIAN_POINT ( 'NONE',  ( -0.4921259842519685179, 3.013402556957069934E-17, -1.569881889763779625 ) ) ;
#7007=CARTESIAN_POINT ( 'NONE',  ( -0.2297883689023225706, -0.3979194638820617858, -1.928289503579150077 ) ) ;
#7012=CARTESIAN_POINT ( 'NONE',  ( -0.3855916753051397139, 0.3382184156732160329, 1.747047244094488194 ) ) ;
#7017=CARTESIAN_POINT ( 'NONE',  ( 0.1867299569291683836, 0.3233561589689052940, -3.115157480314960647 ) ) ;
#7021=CARTESIAN_POINT ( 'NONE',  ( 0.08676778863011423704, 0.3239425792934499948, 1.953740157480315043 ) ) ;
#7028=EDGE_CURVE ( 'NONE', #724, #18101, #4952, .T. ) ;
#7031=FACE_OUTER_BOUND ( 'NONE', #4030, .T. ) ;
#7036=CARTESIAN_POINT ( 'NONE',  ( -0.3184841198566451537, -0.1570220809524492667, 1.953740157480315043 ) ) ;
#7056=EDGE_CURVE ( 'NONE', #14958, #1047, #22672, .T. ) ;
#7058=CARTESIAN_POINT ( 'NONE',  ( -0.3642352168757148623, 0.4152525734086685016, 0.9399606299212598381 ) ) ;
#7072=CARTESIAN_POINT ( 'NONE',  ( 0.3007905576423755556, -0.1482986320106471911, 1.953740157480315043 ) ) ;
#7077=CARTESIAN_POINT ( 'NONE',  ( 0.4954156765914815574, -0.2860899518037339773, 0.9399606299212598381 ) ) ;
#7078=CARTESIAN_POINT ( 'NONE',  ( 0.3145317858139327627, -0.4092783051644229841, 1.766732283464566899 ) ) ;
#7090=ADVANCED_FACE ( 'NONE', ( #24122 ), #23591, .T. ) ;
#7091=CARTESIAN_POINT ( 'NONE',  ( -0.4599954779395757920, 0.2268956277328612881, -1.550196850393700920 ) ) ;
#7101=CYLINDRICAL_SURFACE ( 'NONE', #15711, 0.4921259842519685179 ) ;
#7103=CARTESIAN_POINT ( 'NONE',  ( -0.3979194638820449104, -0.2297883689023288989, -1.928289503579160513 ) ) ;
#7118=VERTEX_POINT ( 'NONE', #17622 ) ;
#7119=CARTESIAN_POINT ( 'NONE',  ( 0.2341075107471200512, 0.2669897767696595703, 1.953740157480315043 ) ) ;
#7121=CARTESIAN_POINT ( 'NONE',  ( 0.4382752542995623779, 0.1173917140416305405, -1.934055118110236338 ) ) ;
#7129=CARTESIAN_POINT ( 'NONE',  ( -0.3349073414798397486, -0.1651192144506304638, -3.115157480314960647 ) ) ;
#7144=CARTESIAN_POINT ( 'NONE',  ( -0.2564944395515793563, -0.4441657790107725323, 1.747047244094488194 ) ) ;
#7148=CARTESIAN_POINT ( 'NONE',  ( -0.1867299569291685502, -0.3233561589689051829, -3.115157480314960647 ) ) ;
#7153=CARTESIAN_POINT ( 'NONE',  ( 0.2211428102655795813, -0.2521176338356631019, 1.953740157480315043 ) ) ;
#7161=CARTESIAN_POINT ( 'NONE',  ( -0.01027864967283271050, 0.1968503937007874127, -3.626971312343105325 ) ) ;
#7164=CARTESIAN_POINT ( 'NONE',  ( -0.01027864967366022390, 0.1968503937007874127, -3.193900446201109578 ) ) ;
#7167=CARTESIAN_POINT ( 'NONE',  ( -0.02576258704323624443, 0.2165354330708661457, -3.176774342847608512 ) ) ;
#7169=CARTESIAN_POINT ( 'NONE',  ( 0.2161381151963039093, -0.2817310484609168442, 1.953740157480315043 ) ) ;
#7175=CARTESIAN_POINT ( 'NONE',  ( 0.06699507805368110080, -0.5085118447801203478, 1.747047244094488194 ) ) ;
#7183=CARTESIAN_POINT ( 'NONE',  ( 0.09193072188197352890, -0.3429848536917953217, 1.953740157480315043 ) ) ;
#7186=CARTESIAN_POINT ( 'NONE',  ( -0.3912931228432220410, 0.3001918266902144361, -1.569881889763779625 ) ) ;
#7190=CARTESIAN_POINT ( 'NONE',  ( -0.5417097841048968965, 0.1839420097223028183, 0.9399606299212598381 ) ) ;
#7206=CARTESIAN_POINT ( 'NONE',  ( -0.3145317858139328737, -0.4092783051644231507, 1.766732283464567121 ) ) ;
#7215=CARTESIAN_POINT ( 'NONE',  ( -0.07874015747999545123, 0.1968503937007873850, -3.558537267005807525 ) ) ;
#7224=CARTESIAN_POINT ( 'NONE',  ( 0.04928528614549729930, 0.3765118517642103702, -3.100567304031763172 ) ) ;
#7227=CARTESIAN_POINT ( 'NONE',  ( 0.1078280746904042159, 0.3175540113612283499, 1.973425196850393970 ) ) ;
#7228=CARTESIAN_POINT ( 'NONE',  ( 0.4423390553432353656, -0.2180862235769564228, -1.550196850393700920 ) ) ;
#7230=CARTESIAN_POINT ( 'NONE',  ( 0.4585215200179055817, 0.03001016326913595253, -1.928289503579156516 ) ) ;
#7232=CARTESIAN_POINT ( 'NONE',  ( -0.5230301363771709955, 0.1775991818008312573, 0.9399606299212598381 ) ) ;
#7233=CARTESIAN_POINT ( 'NONE',  ( -0.07874015748031511219, 0.1968503937007874127, -3.548228346456693050 ) ) ;
#7237=CARTESIAN_POINT ( 'NONE',  ( -0.3912931228432220410, 0.3001918266902144361, -1.569881889763779625 ) ) ;
#7247=CARTESIAN_POINT ( 'NONE',  ( 0.3075341118175934363, 0.1775236553382197324, 1.953740157480314821 ) ) ;
#7250=CARTESIAN_POINT ( 'NONE',  ( 0.05926487674659523808, -0.4498374011143459472, -1.934055118110236338 ) ) ;
#7261=CARTESIAN_POINT ( 'NONE',  ( -0.3267488823401686893, 0.1886891683789005680, -3.100567304031762284 ) ) ;
#7264=ORIENTED_EDGE ( 'NONE', *, *, #12244, .T. ) ;
#7267=ADVANCED_FACE ( 'NONE', ( #668 ), #23367, .T. ) ;
#7276=CARTESIAN_POINT ( 'NONE',  ( 0.3855916753051394363, 0.3382184156732163660, 1.747047244094488194 ) ) ;
#7280=CARTESIAN_POINT ( 'NONE',  ( -0.3740848232703756771, 0.04928467685643712209, -3.100567304031759175 ) ) ;
#7285=ORIENTED_EDGE ( 'NONE', *, *, #11966, .F. ) ;
#7293=EDGE_LOOP ( 'NONE', ( #10418, #11662, #26327, #25967 ) ) ;
#7297=CARTESIAN_POINT ( 'NONE',  ( -0.04841158226283256288, 0.1968503937007874127, -3.209690007240762366 ) ) ;
#7303=CARTESIAN_POINT ( 'NONE',  ( 0.02319089060378159983, 0.3543307086614173596, 1.953740157480315043 ) ) ;
#7312=CARTESIAN_POINT ( 'NONE',  ( -0.5314960629921260393, -0.03478633594543723700, 1.747047244094488194 ) ) ;
#7313=FACE_OUTER_BOUND ( 'NONE', #13168, .T. ) ;
#7323=CARTESIAN_POINT ( 'NONE',  ( -0.4669911931914798586, -0.1585706980422492696, -1.569881889763779625 ) ) ;
#7326=CARTESIAN_POINT ( 'NONE',  ( -0.3362148458988341582, -0.4382482975805541692, 0.9399606299212598381 ) ) ;
#7343=CARTESIAN_POINT ( 'NONE',  ( 0.1078280746903870629, -0.3175540113612215221, 1.953740157480315043 ) ) ;
#7372=CARTESIAN_POINT ( 'NONE',  ( -0.2211428102655751127, -0.2521176338356575508, 1.973425196850393970 ) ) ;
#7373=CARTESIAN_POINT ( 'NONE',  ( -0.4954415918535620134, 0.1327036767636087800, -1.550196850393700920 ) ) ;
#7374=CARTESIAN_POINT ( 'NONE',  ( -0.5368353335967093187, 0.1442704874421232575, 0.9202755905511812440 ) ) ;
#7379=CARTESIAN_POINT ( 'NONE',  ( -0.4423390553432505201, 0.2180862235769355506, -1.569881889763779625 ) ) ;
#7393=CARTESIAN_POINT ( 'NONE',  ( 0.2761764805255846333, -0.3599896729929844552, -1.934055118110236338 ) ) ;
#7404=CARTESIAN_POINT ( 'NONE',  ( -0.4303639208847589437, -0.1153623459797714496, -1.934055118110236560 ) ) ;
#7405=CARTESIAN_POINT ( 'NONE',  ( -0.3765118517642104257, 0.000000000000000000, -3.100567304031763172 ) ) ;
#7406=CARTESIAN_POINT ( 'NONE',  ( 0.000000000000000000, 0.000000000000000000, 1.914370078775489148 ) ) ;
#7409=CARTESIAN_POINT ( 'NONE',  ( -0.4446020952038907681, -0.02909913904661340714, -1.934055118110236338 ) ) ;
#7414=CARTESIAN_POINT ( 'NONE',  ( 0.3855916753051445989, -0.3382184156732112590, 1.766732283464566899 ) ) ;
#7417=CARTESIAN_POINT ( 'NONE',  ( -0.2836590635674511307, -0.2488091035917043836, -3.100567304031761395 ) ) ;
#7422=CARTESIAN_POINT ( 'NONE',  ( 0.3239425792934414461, -0.08676778863010961573, 1.953740157480315043 ) ) ;
#7438=CARTESIAN_POINT ( 'NONE',  ( 0.000000000000000000, 0.000000000000000000, 1.953740157480315043 ) ) ;
#7441=CARTESIAN_POINT ( 'NONE',  ( -0.2161381151963043257, -0.2817310484609166221, 1.953740157480315043 ) ) ;
#7447=DIRECTION ( 'NONE',  ( 1.000000000000000000, 0.000000000000000000, 0.000000000000000000 ) ) ;
#7449=CARTESIAN_POINT ( 'NONE',  ( -0.2355331214654103611, -0.4777261797697372470, 1.747047244094488194 ) ) ;
#7455=VERTEX_POINT ( 'NONE', #15521 ) ;
#7458=EDGE_CURVE ( 'NONE', #7455, #4928, #5959, .T. ) ;
#7464=CARTESIAN_POINT ( 'NONE',  ( -0.4763861460130329739, 0.1275996891957754675, -1.569881889763779625 ) ) ;
#7466=CARTESIAN_POINT ( 'NONE',  ( -0.2860899518037490763, 0.4954156765914824456, 0.9399606299212598381 ) ) ;
#7481=CARTESIAN_POINT ( 'NONE',  ( -0.2660793235464293804, -0.2041304421298503202, 1.953740157480315043 ) ) ;
#7499=CARTESIAN_POINT ( 'NONE',  ( 0.07870736599822267254, 0.2165354330708661457, -3.608715228723538893 ) ) ;
#7509=DIRECTION ( 'NONE',  ( -1.000000000000000000, 0.000000000000000000, 0.000000000000000000 ) ) ;
#7514=CARTESIAN_POINT ( 'NONE',  ( -0.4600326175569863785, 0.2268096725200117181, -1.550196850393700920 ) ) ;
#7517=CARTESIAN_POINT ( 'NONE',  ( -0.2442565704126265502, 0.4954197419817717996, 0.9399606299212598381 ) ) ;
#7523=CARTESIAN_POINT ( 'NONE',  ( 0.3252100150720242944, 0.3707612262533179215, -1.569881889763779625 ) ) ;
#7543=ORIENTED_EDGE ( 'NONE', *, *, #3094, .T. ) ;
#7547=CARTESIAN_POINT ( 'NONE',  ( -0.3765118517642104257, 0.000000000000000000, -3.100567304031763172 ) ) ;
#7552=CARTESIAN_POINT ( 'NONE',  ( -0.4527559054764770385, 0.02963280468031418563, -1.934055118110236338 ) ) ;
#7560=CARTESIAN_POINT ( 'NONE',  ( 0.1649135259617203753, -0.4856708409200670151, 1.747047244094488194 ) ) ;
#7563=CARTESIAN_POINT ( 'NONE',  ( 0.2296683860596776539, 0.2993674444872277962, -3.100567304031764060 ) ) ;
#7567=CARTESIAN_POINT ( 'NONE',  ( -0.03359157810797404331, 0.5118124425185099913, -1.550196850393700920 ) ) ;
#7571=CARTESIAN_POINT ( 'NONE',  ( 0.05819755867303724045, 0.4417361510194101615, -1.934055118110236338 ) ) ;
#7587=CARTESIAN_POINT ( 'NONE',  ( -0.06048688188729484105, 0.2165354330708661457, -3.193930428897817198 ) ) ;
#7591=CARTESIAN_POINT ( 'NONE',  ( -0.3362336590883612808, 0.1141709026133623794, 1.953740157480315043 ) ) ;
#7593=ORIENTED_EDGE ( 'NONE', *, *, #27111, .F. ) ;
#7601=CARTESIAN_POINT ( 'NONE',  ( 0.1327036767659768302, -0.4954415918531079877, 1.747047244094488194 ) ) ;
#7603=CARTESIAN_POINT ( 'NONE',  ( 0.3121994997598600552, -0.4069448477555897004, 1.766732283464566899 ) ) ;
#7611=CARTESIAN_POINT ( 'NONE',  ( -0.3858397471888794783, 0.2228126397720086582, -1.934055118110236338 ) ) ;
#7616=CARTESIAN_POINT ( 'NONE',  ( -0.4423390553432507977, -0.2180862235769348567, -1.569881889763779625 ) ) ;
#7630=CARTESIAN_POINT ( 'NONE',  ( 0.04380447413658805633, -0.3324885138898231451, 1.953740157480315043 ) ) ;
#7647=CARTESIAN_POINT ( 'NONE',  ( -0.4442189740295497402, 0.2564173815260738509, -1.550196850393700920 ) ) ;
#7658=CARTESIAN_POINT ( 'NONE',  ( 0.3381512095065888901, -0.3856568748492107401, -1.550196850393700920 ) ) ;
#7660=CARTESIAN_POINT ( 'NONE',  ( 0.2904160862623631489, 0.1677079028045434517, 1.973425196850393970 ) ) ;
#7663=CARTESIAN_POINT ( 'NONE',  ( -0.1442704874421230077, 0.5368353335967094297, 0.9202755905511812440 ) ) ;
#7670=CARTESIAN_POINT ( 'NONE',  ( 0.3912931228432083297, 0.3001918266902350307, -1.569881889763779625 ) ) ;
#7673=VERTEX_POINT ( 'NONE', #8420 ) ;
#7675=CARTESIAN_POINT ( 'NONE',  ( 0.2356240016490815659, 0.4776900717921119810, 1.747047244094488194 ) ) ;
#7676=DIRECTION ( 'NONE',  ( -0.000000000000000000, -0.000000000000000000, 1.000000000000000000 ) ) ;
#7700=CARTESIAN_POINT ( 'NONE',  ( -0.1791085948260308092, -0.3102804211135123946, -3.115157480314960203 ) ) ;
#7704=CARTESIAN_POINT ( 'NONE',  ( -0.3411003281196917092, 0.2991932138496784521, -1.934055118110236338 ) ) ;
#7712=CARTESIAN_POINT ( 'NONE',  ( -0.3242071728275120468, 0.4225965726692976765, 1.747047244094488194 ) ) ;
#7714=ORIENTED_EDGE ( 'NONE', *, *, #17953, .F. ) ;
#7716=CARTESIAN_POINT ( 'NONE',  ( -0.04928467685644277035, -0.3740848232703729015, -3.100567304031765392 ) ) ;
#7724=CARTESIAN_POINT ( 'NONE',  ( 0.3535065162672724748, -0.2712027394948692827, -1.934055118110236338 ) ) ;
#7746=CARTESIAN_POINT ( 'NONE',  ( -0.1712563538833044852, 0.5043504886477827576, 1.747047244094488194 ) ) ;
#7747=CARTESIAN_POINT ( 'NONE',  ( 0.2268096725222443211, -0.4600326175560562336, 1.766732283464566899 ) ) ;
#7751=CARTESIAN_POINT ( 'NONE',  ( -0.1791601451668828893, 0.3102476824511414266, -3.115157480314960647 ) ) ;
#7759=CARTESIAN_POINT ( 'NONE',  ( 0.2466292688015061796, 0.4270824798167727199, -1.569881889763779625 ) ) ;
#7763=EDGE_CURVE ( 'NONE', #2791, #3990, #5720, .T. ) ;
#7779=CARTESIAN_POINT ( 'NONE',  ( -0.4921259842519685179, 3.013402556957069934E-17, -1.569881889763779625 ) ) ;
#7789=EDGE_CURVE ( 'NONE', #1806, #22055, #90, .T. ) ;
#7790=DIRECTION ( 'NONE',  ( 0.000000000000000000, 0.000000000000000000, 1.000000000000000000 ) ) ;
#7798=ORIENTED_EDGE ( 'NONE', *, *, #15691, .T. ) ;
#7801=CARTESIAN_POINT ( 'NONE',  ( -0.2268096725200377806, -0.4600326175569655618, -1.550196850393700920 ) ) ;
#7806=CARTESIAN_POINT ( 'NONE',  ( -0.5335524835332334792, -0.1429116519061227608, 0.9202755905511811330 ) ) ;
#7807=CARTESIAN_POINT ( 'NONE',  ( 6.136516277395897527E-17, 0.2165354330708661457, -3.646653543307086576 ) ) ;
#7841=CARTESIAN_POINT ( 'NONE',  ( -0.2181214148710382827, -0.2842163005027896761, -3.115157480314960203 ) ) ;
#7846=CARTESIAN_POINT ( 'NONE',  ( 0.2938049579018460755, 0.3349573549949649842, -1.934055118110236338 ) ) ;
#7849=CARTESIAN_POINT ( 'NONE',  ( -0.5043504886477523375, 0.1712563538833050680, 1.747047244094488194 ) ) ;
#7852=ORIENTED_EDGE ( 'NONE', *, *, #522, .F. ) ;
#7855=CARTESIAN_POINT ( 'NONE',  ( 0.3384212623783103835, 0.1668516812751408562, -3.100567304031765392 ) ) ;
#7860=CARTESIAN_POINT ( 'NONE',  ( 0.01288382760289894825, 0.2165354330708661457, -3.646653543307086576 ) ) ;
#7865=AXIS2_PLACEMENT_3D ( 'NONE', #13421, #17661, #26839 ) ;
#7867=CARTESIAN_POINT ( 'NONE',  ( -0.09269288654273742656, -0.3460635936745020680, -3.115157480314960647 ) ) ;
#7870=DIRECTION ( 'NONE',  ( 0.000000000000000000, 0.000000000000000000, -1.000000000000000000 ) ) ;
#7879=CARTESIAN_POINT ( 'NONE',  ( -0.5672097974520583508, 0.07461436618597647175, 0.9399606299212600602 ) ) ;
#7885=CARTESIAN_POINT ( 'NONE',  ( 0.04956879728060044343, 0.2165354330708660624, -3.634230943735654140 ) ) ;
#7898=CARTESIAN_POINT ( 'NONE',  ( 0.4423390553432353656, -0.2180862235769564228, -1.550196850393700920 ) ) ;
#7923=DIRECTION ( 'NONE',  ( 1.000000000000000000, 0.000000000000000000, 0.000000000000000000 ) ) ;
#7942=CARTESIAN_POINT ( 'NONE',  ( 0.2904160862623596517, -0.1677079028045486975, 1.973425196850393970 ) ) ;
#7946=CARTESIAN_POINT ( 'NONE',  ( -0.03607471876262562799, -0.5511811023622048555, 0.9399606299212598381 ) ) ;
#7980=VERTEX_POINT ( 'NONE', #26891 ) ;
#7981=CARTESIAN_POINT ( 'NONE',  ( 0.3858397471888846408, -0.2228126397719881469, -1.934055118110236338 ) ) ;
#7991=CARTESIAN_POINT ( 'NONE',  ( 0.2564944395515637576, -0.4441657790108029524, 1.747047244094488194 ) ) ;
#7994=CARTESIAN_POINT ( 'NONE',  ( -0.4539000224940974992, -0.3482225189666513510, 0.9399606299212598381 ) ) ;
#8000=CARTESIAN_POINT ( 'NONE',  ( -0.3362336590883612808, 0.1141709026133623794, 1.953740157480315043 ) ) ;
#8005=CARTESIAN_POINT ( 'NONE',  ( -0.3289909311256231650, -0.1896185148830505374, -3.100567304031763616 ) ) ;
#8006=CARTESIAN_POINT ( 'NONE',  ( -0.3482225189666627863, 0.4539000224941008854, 0.9399606299212598381 ) ) ;
#8011=CARTESIAN_POINT ( 'NONE',  ( -0.02339816079119098197, 0.3574975638436101444, -3.115157480314960647 ) ) ;
#8017=DIRECTION ( 'NONE',  ( -0.000000000000000000, -0.000000000000000000, 1.000000000000000000 ) ) ;
#8025=CARTESIAN_POINT ( 'NONE',  ( -0.03746919241557482988, 0.5708675606921427281, 0.9399606299212600602 ) ) ;
#8027=CARTESIAN_POINT ( 'NONE',  ( 0.5118110236220472231, 3.133938659235352953E-17, 1.766732283464566899 ) ) ;
#8029=CARTESIAN_POINT ( 'NONE',  ( 0.000000000000000000, 0.000000000000000000, 0.9399606299212598381 ) ) ;
#8032=CARTESIAN_POINT ( 'NONE',  ( -0.06957181182499248828, -0.5280699926562971713, 1.747047244094488194 ) ) ;
#8033=CARTESIAN_POINT ( 'NONE',  ( -0.5118110236220472231, -0.03349795313264326835, 1.766732283464566899 ) ) ;
#8036=CARTESIAN_POINT ( 'NONE',  ( -0.3102476824511312681, 0.1791601451669032896, -3.115157480314960647 ) ) ;
#8038=CARTESIAN_POINT ( 'NONE',  ( -0.4465874321618644172, -0.1200170377978878600, -1.928289503579156960 ) ) ;
#8041=CARTESIAN_POINT ( 'NONE',  ( -0.2521176338356575508, 0.2211428102655751127, 1.973425196850393970 ) ) ;
#8044=CARTESIAN_POINT ( 'NONE',  ( -0.06441834428466408635, -0.4889536969035170877, -1.550196850393700920 ) ) ;
#8085=CARTESIAN_POINT ( 'NONE',  ( 0.5085315017394973491, -0.06690352886883006722, -1.550196850393700476 ) ) ;
#8087=CARTESIAN_POINT ( 'NONE',  ( 0.08676778863011423704, 0.3239425792934499948, 1.953740157480315043 ) ) ;
#8088=CARTESIAN_POINT ( 'NONE',  ( 0.5118110236220473341, -0.03349795313024152288, -1.550196850393700920 ) ) ;
#8090=CARTESIAN_POINT ( 'NONE',  ( 0.03607471876262387245, -0.5511811023622048555, 0.9399606299212598381 ) ) ;
#8096=AXIS2_PLACEMENT_3D ( 'NONE', #18577, #7870, #22992 ) ;
#8099=CARTESIAN_POINT ( 'NONE',  ( -0.4069448477569480582, 0.3121994997578198539, -1.550196850393700920 ) ) ;
#8112=EDGE_LOOP ( 'NONE', ( #20430, #3640, #7264, #7852 ) ) ;
#8117=CARTESIAN_POINT ( 'NONE',  ( -0.2361997806693948987, -0.2693761163849906493, -3.115157480314960647 ) ) ;
#8119=CARTESIAN_POINT ( 'NONE',  ( 0.2180862235769348290, -0.4423390553432507977, -1.569881889763779625 ) ) ;
#8121=CARTESIAN_POINT ( 'NONE',  ( -0.2761764805255463306, -0.3599896729929341621, -1.934055118110236338 ) ) ;
#8122=CARTESIAN_POINT ( 'NONE',  ( -0.4585215200179055817, 0.03001016326912889221, -1.928289503579156516 ) ) ;
#8123=ORIENTED_EDGE ( 'NONE', *, *, #15837, .T. ) ;
#8126=CARTESIAN_POINT ( 'NONE',  ( 0.3765118517642104257, -2.263258471485603576E-17, -3.100567304031763172 ) ) ;
#8127=CARTESIAN_POINT ( 'NONE',  ( -0.5314960629921260393, 0.03478633594543736884, 1.747047244094488194 ) ) ;
#8134=CARTESIAN_POINT ( 'NONE',  ( -0.1775220790476026711, -0.3075317527318737199, 1.953740157480315043 ) ) ;
#8137=B_SPLINE_CURVE_WITH_KNOTS ( 'NONE', 3,
 ( #22007, #162, #22273, #24125 ),
 .UNSPECIFIED., .F., .F.,
 ( 4, 4 ),
 ( 0.000000000000000000, 1.000000000000000000 ),
 .UNSPECIFIED. ) ;
#8138=CARTESIAN_POINT ( 'NONE',  ( 0.2341512108694265570, -0.2669480828848097009, 1.953740157480315043 ) ) ;
#8146=CARTESIAN_POINT ( 'NONE',  ( -0.4539000224941007744, 0.3482225189667277343, 0.9399606299212598381 ) ) ;
#8159=CARTESIAN_POINT ( 'NONE',  ( 0.3429980251342297226, -0.09187177619658888628, 1.953740157480315043 ) ) ;
#8168=CARTESIAN_POINT ( 'NONE',  ( 0.4856708409200598542, 0.1649135259617023896, 1.747047244094488194 ) ) ;
#8171=CARTESIAN_POINT ( 'NONE',  ( -2.685748425196850164E-17, 0.000000000000000000, -3.666338582670846780 ) ) ;
#8175=CARTESIAN_POINT ( 'NONE',  ( 0.1677079028045456166, 0.2904160862623617056, 1.973425196850393970 ) ) ;
#8176=ORIENTED_EDGE ( 'NONE', *, *, #26211, .T. ) ;
#8177=CARTESIAN_POINT ( 'NONE',  ( -0.2180862235769436830, 0.4423390553432706707, -1.550196850393700920 ) ) ;
#8199=DIRECTION ( 'NONE',  ( 0.000000000000000000, 0.000000000000000000, -1.000000000000000000 ) ) ;
#8201=DIRECTION ( 'NONE',  ( -0.000000000000000000, -1.000000000000000000, -0.000000000000000000 ) ) ;
#8207=CARTESIAN_POINT ( 'NONE',  ( -0.5118110236220473341, 0.000000000000000000, -1.550196850393700920 ) ) ;
#8219=DIRECTION ( 'NONE',  ( 0.000000000000000000, 0.000000000000000000, -1.000000000000000000 ) ) ;
#8224=CARTESIAN_POINT ( 'NONE',  ( 0.2660793235464301021, -0.2041304421298313909, 1.973425196850393970 ) ) ;
#8225=CARTESIAN_POINT ( 'NONE',  ( 0.4856708409191422549, -0.1649135259639211148, -1.550196850393700920 ) ) ;
#8227=CARTESIAN_POINT ( 'NONE',  ( 0.2762247810518927427, -0.4783323773986943306, 0.9399606299212598381 ) ) ;
#8230=B_SPLINE_SURFACE_WITH_KNOTS ( 'NONE', 2, 3, ( 
 ( #4567, #23426, #24060, #13321, #6833, #17687, #27792, #1929, #6318, #14949, #2573, #17570, #26311, #6976, #13448, #26438, #2705, #11338, #24326, #2838, #19955, #4975, #13588, #5254, #24741, #9623, #20514, #26574, #22921, #891, #1172, #16282, #20793, #18074, #13875, #18366, #17941, #26718, #3394, #20231, #14169, #2976, #5104, #20653, #24885, #22493, #3255, #3123, #27019, #9771, #16412, #1305, #27162, #22632, #22769, #12037, #9914, #18514, #9478, #15999, #24453, #11750, #7806, #5403, #11895, #25027 ),
 ( #5691, #3540, #20371, #12168, #7232, #9335, #13729, #22351, #1029, #14021, #18227, #26865, #7517, #8373, #14756, #25457, #27865, #12602, #4129, #3686, #10182, #16986, #21223, #23209, #25598, #14608, #17122, #21363, #8502, #15018, #23498, #12734, #25739, #6391, #3841, #1580, #19234, #23633, #1865, #10470, #27295, #5835, #19088, #8227, #18656, #27586, #12315, #21070, #8090, #7946, #16847, #1719, #18801, #2000, #27436, #10331, #12874, #10049, #20936, #1438, #23363, #16547, #16703, #6254, #25165, #18951 ),
 ( #23068, #6121, #27727, #14459, #3987, #14889, #10611, #25314, #5973, #2274, #8772, #21503, #332, #19663, #11038, #15436, #4406, #4946, #15693, #13012, #17534, #6526, #4666, #6804, #24296, #13417, #15158, #17261, #4802, #26411, #19516, #22044, #26014, #17395, #26149, #21776, #13294, #10758, #7077, #21643, #21917, #19790, #2143, #10898, #6669, #2544, #74, #205, #15567, #23767, #26279, #15301, #25879, #2678, #453, #23907, #24027, #4545, #11170, #9044, #579, #11307, #19926, #17658, #6945, #24167 ) ),
 .UNSPECIFIED., .F., .T., .F.,
 ( 3, 3 ),
 ( 4, 2, 2, 2, 2, 2, 2, 2, 2, 2, 2, 2, 2, 2, 2, 2, 2, 2, 2, 2, 2, 2, 2, 2, 2, 2, 2, 2, 2, 2, 2, 2, 4 ),
 ( 0.000000000000000000, 1.000000000000000000 ),
 ( 0.000000000000000000, 0.1963495408493620697, 0.3926990816987241395, 0.5890486225480862092, 0.7853981633974482790, 0.9817477042468103487, 1.178097245096172418, 1.374446785945534488, 1.570796326794896558, 1.767145867644258628, 1.963495408493620697, 2.159844949342982545, 2.356194490192344837, 2.552544031041707129, 2.748893571891068976, 2.945243112740430824, 3.141592653589793116, 3.337942194439155408, 3.534291735288517255, 3.730641276137879103, 3.926990816987241395, 4.123340357836603687, 4.319689898685965090, 4.516039439535327382, 4.712388980384689674, 4.908738521234051966, 5.105088062083414258, 5.301437602932775661, 5.497787143782137953, 5.694136684631500245, 5.890486225480861648, 6.086835766330223940, 6.283185307179586232 ),
 .UNSPECIFIED. ) ;
#8234=CARTESIAN_POINT ( 'NONE',  ( 0.5280918803863992039, 0.06946904943156809176, 1.747047244094488860 ) ) ;
#8237=CARTESIAN_POINT ( 'NONE',  ( -0.5085118447796660446, 0.06699507805605008082, -1.550196850393700920 ) ) ;
#8242=CARTESIAN_POINT ( 'NONE',  ( 0.1379032889623779401, -0.5144765700550301135, 1.747047244094488194 ) ) ;
#8246=CARTESIAN_POINT ( 'NONE',  ( -0.09776456083825368903, 0.2994062042887761232, -3.259552405628561189 ) ) ;
#8249=EDGE_LOOP ( 'NONE', ( #301, #23582, #13785, #6351 ) ) ;
#8254=CARTESIAN_POINT ( 'NONE',  ( 0.09842519685039370636, 0.2165354330708661457, -3.272637795275590733 ) ) ;
#8256=CARTESIAN_POINT ( 'NONE',  ( -0.4121342552748409327, 0.2031943647053852109, -1.928289503579154074 ) ) ;
#8273=EDGE_CURVE ( 'NONE', #15380, #10004, #23976, .T. ) ;
#8278=CARTESIAN_POINT ( 'NONE',  ( -0.2341512108694372152, -0.2669480828848191933, 1.953740157480315043 ) ) ;
#8290=CARTESIAN_POINT ( 'NONE',  ( 0.3460635936744816399, 0.09269288654273792616, -3.115157480314960647 ) ) ;
#8291=CARTESIAN_POINT ( 'NONE',  ( 6.136516277395897527E-17, 0.2165354330708661457, -3.646653543307086576 ) ) ;
#8298=CARTESIAN_POINT ( 'NONE',  ( 0.3362336590883814313, -0.1141709026133623794, 1.953740157480315043 ) ) ;
#8308=CARTESIAN_POINT ( 'NONE',  ( 0.08600259727896249207, 0.2165354330708661457, -3.597797143737292647 ) ) ;
#8313=CARTESIAN_POINT ( 'NONE',  ( 0.2842490391651530390, 0.2180698645301770711, -3.115157480314960647 ) ) ;
#8317=CARTESIAN_POINT ( 'NONE',  ( 0.2904160862623596517, -0.1677079028045486975, 1.973425196850393970 ) ) ;
#8320=CARTESIAN_POINT ( 'NONE',  ( 0.4921259842519685179, -0.03220957031753991784, -1.550196850393700920 ) ) ;
#8340=CARTESIAN_POINT ( 'NONE',  ( 0.4006498629591506155, 0.2309201403895323190, -1.928289503579156960 ) ) ;
#8344=CARTESIAN_POINT ( 'NONE',  ( 0.09586345222254785692, 0.1968503937007873850, -3.246875207736358515 ) ) ;
#8363=CARTESIAN_POINT ( 'NONE',  ( -0.5314960629921260393, 6.402768735150616610E-17, 1.747047244094488194 ) ) ;
#8366=CARTESIAN_POINT ( 'NONE',  ( -0.07874015748031495954, 0.1968503937007873850, -3.456364829396327831 ) ) ;
#8369=DIRECTION ( 'NONE',  ( 1.000000000000000000, 0.000000000000000000, 0.000000000000000000 ) ) ;
#8373=CARTESIAN_POINT ( 'NONE',  ( -0.1775991818008579581, 0.5230301363771275858, 0.9399606299212598381 ) ) ;
#8380=CARTESIAN_POINT ( 'NONE',  ( 0.2564944395535760924, 0.4441657790094617475, -1.550196850393700920 ) ) ;
#8398=CARTESIAN_POINT ( 'NONE',  ( -0.4921259842519685179, 0.000000000000000000, -1.569881889763779625 ) ) ;
#8399=CARTESIAN_POINT ( 'NONE',  ( -0.2991932138496239402, -0.3411003281196705594, -1.934055118110236338 ) ) ;
#8408=ORIENTED_EDGE ( 'NONE', *, *, #19019, .F. ) ;
#8413=CARTESIAN_POINT ( 'NONE',  ( -0.3429980251342298336, -0.09187177619659059324, 1.953740157480315043 ) ) ;
#8420=CARTESIAN_POINT ( 'NONE',  ( -1.452994488188976472E-16, 0.3149606299212598381, -3.646653543307086576 ) ) ;
#8423=CARTESIAN_POINT ( 'NONE',  ( 0.2807137536170459802, 0.2462256503456008716, -3.115157480314960647 ) ) ;
#8432=CARTESIAN_POINT ( 'NONE',  ( -0.5708661417322834497, 0.03749087971309117417, 0.9399606299212597271 ) ) ;
#8438=CARTESIAN_POINT ( 'NONE',  ( -0.4856708409200606313, -0.1649135259617140470, 1.766732283464566899 ) ) ;
#8442=CARTESIAN_POINT ( 'NONE',  ( -0.06002032661671168751, -0.4585215200179056372, -1.928289503579156516 ) ) ;
#8444=CARTESIAN_POINT ( 'NONE',  ( 0.08676778863010990717, 0.3239425792934408910, 1.973425196850393970 ) ) ;
#8447=CARTESIAN_POINT ( 'NONE',  ( 0.2180862235769456536, -0.4423390553432768879, -1.550196850393700920 ) ) ;
#8457=CARTESIAN_POINT ( 'NONE',  ( -0.006553447611498987302, 0.3149606299212598381, -3.646653543307087020 ) ) ;
#8460=B_SPLINE_SURFACE_WITH_KNOTS ( 'NONE', 2, 3, ( 
 ( #25708, #19207, #1447, #10732, #6359, #1972, #23877, #10582, #14993, #8881, #20800, #17499, #19480, #25986, #46, #2376, #23738, #6224 ),
 ( #15265, #11008, #8344, #27692, #306, #19346, #23607, #8609, #4373, #25847, #6497, #26120, #2243, #174, #17092, #10865, #27835, #15410 ),
 ( #8749, #23471, #10056, #4242, #17369, #12843, #18662, #16957, #25572, #14860, #12705, #21338, #8472, #2116, #4512, #13121, #9415, #13394 ) ),
 .UNSPECIFIED., .F., .F., .F.,
 ( 3, 3 ),
 ( 4, 2, 2, 2, 2, 2, 2, 2, 4 ),
 ( 0.000000000000000000, 1.000000000000000000 ),
 ( 1.570796326794896558, 1.963495408493620697, 2.356194490192344837, 2.748893571891068976, 3.141592653589793116, 3.534291735288517255, 3.926990816987241395, 4.319689898685965090, 4.712388980384689674 ),
 .UNSPECIFIED. ) ;
#8462=CARTESIAN_POINT ( 'NONE',  ( -0.4776900717921101491, 0.2356240016489475342, 1.747047244094488638 ) ) ;
#8470=FACE_OUTER_BOUND ( 'NONE', #19491, .T. ) ;
#8471=B_SPLINE_CURVE_WITH_KNOTS ( 'NONE', 3,
 ( #6442, #6588, #4188, #19292, #15714, #601, #4824, #23691, #10534, #8291 ),
 .UNSPECIFIED., .F., .F.,
 ( 4, 2, 2, 2, 4 ),
 ( 0.000000000000000000, 0.1250000000000000000, 0.2500000000000000000, 0.3750000000000000000, 0.5000000000000000000 ),
 .UNSPECIFIED. ) ;
#8472=CARTESIAN_POINT ( 'NONE',  ( -0.04838950581350995317, 0.1968503937007873850, -3.209671902477075900 ) ) ;
#8481=CARTESIAN_POINT ( 'NONE',  ( 0.5476281405333178753, -0.07214854559198131956, 0.9202755905511811330 ) ) ;
#8502=CARTESIAN_POINT ( 'NONE',  ( 0.4954197419817713000, 0.2442565704126274662, 0.9399606299212598381 ) ) ;
#8505=CARTESIAN_POINT ( 'NONE',  ( 0.1151343661286149123, 0.3392608232659918288, -3.115157480314960647 ) ) ;
#8508=VERTEX_POINT ( 'NONE', #1601 ) ;
#8509=CONICAL_SURFACE ( 'NONE', #17949, 0.4527559054764771496, 0.7853981642949022790 ) ;
#8510=CARTESIAN_POINT ( 'NONE',  ( 0.2564944395535923571, -0.4441657790094409863, -1.550196850393700920 ) ) ;
#8511=CARTESIAN_POINT ( 'NONE',  ( 0.5708647227724241713, -0.03746919241596944478, 0.9399606299212595051 ) ) ;
#8514=CARTESIAN_POINT ( 'NONE',  ( 0.2662790972926426525, -0.4613045817969299023, 1.747047244094488416 ) ) ;
#8518=EDGE_CURVE ( 'NONE', #4351, #7455, #11155, .T. ) ;
#8525=ORIENTED_EDGE ( 'NONE', *, *, #6267, .T. ) ;
#8532=CARTESIAN_POINT ( 'NONE',  ( 0.4069519308877023178, -0.2006393256663573099, -1.934055118110236338 ) ) ;
#8544=CARTESIAN_POINT ( 'NONE',  ( 0.000000000000000000, 0.000000000000000000, -1.550196850393700920 ) ) ;
#8548=CARTESIAN_POINT ( 'NONE',  ( -0.1970988029427959420, 0.3995913070737888706, -1.934055118110236338 ) ) ;
#8550=CARTESIAN_POINT ( 'NONE',  ( -0.1141709026133645999, 0.3362336590883638343, 1.953740157480315043 ) ) ;
#8558=CARTESIAN_POINT ( 'NONE',  ( -2.685748425196850164E-17, 0.000000000000000000, -3.036417322828325105 ) ) ;
#8561=CARTESIAN_POINT ( 'NONE',  ( -0.2272836761398000505, 0.2962590301041647667, -3.115157480314960647 ) ) ;
#8575=FACE_OUTER_BOUND ( 'NONE', #1694, .T. ) ;
#8576=CARTESIAN_POINT ( 'NONE',  ( -0.3382184156732166436, 0.3855916753051391033, 1.747047244094488194 ) ) ;
#8580=CARTESIAN_POINT ( 'NONE',  ( 0.3213305936751379432, -0.1584254766472190656, -3.115157480314960647 ) ) ;
#8583=CARTESIAN_POINT ( 'NONE',  ( -0.2817828961649163078, -0.3666644560843326794, -1.928289503579157405 ) ) ;
#8586=CARTESIAN_POINT ( 'NONE',  ( 0.1677079028045344034, -0.2904160862623691997, 1.973425196850393970 ) ) ;
#8596=DIRECTION ( 'NONE',  ( -0.7071067818211439482, 0.000000000000000000, -0.7071067805519510863 ) ) ;
#8603=CARTESIAN_POINT ( 'NONE',  ( -0.4121342552748326060, -0.2031943647053980340, -1.928289503579156960 ) ) ;
#8609=CARTESIAN_POINT ( 'NONE',  ( 0.02576258753919729791, 0.1968503937007873850, -3.176774343053085481 ) ) ;
#8622=CARTESIAN_POINT ( 'NONE',  ( -0.5511811023622048555, 0.03607471876259065596, 0.9399606299212598381 ) ) ;
#8629=CARTESIAN_POINT ( 'NONE',  ( -0.09842519685039366473, 0.1968503937007873850, -3.548228346456693050 ) ) ;
#8637=CARTESIAN_POINT ( 'NONE',  ( 0.06690297524255699180, -0.5085287184740814315, -1.550196850393700920 ) ) ;
#8647=CARTESIAN_POINT ( 'NONE',  ( 0.5118110236220473341, -0.03349795313024152288, -1.550196850393700920 ) ) ;
#8648=CARTESIAN_POINT ( 'NONE',  ( -0.3483099419450385037, -0.4538399017590776796, 0.9399606299212598381 ) ) ;
#8662=ORIENTED_EDGE ( 'NONE', *, *, #22533, .F. ) ;
#8665=CARTESIAN_POINT ( 'NONE',  ( -0.2466292688015410683, 0.4270824798167730529, -1.550196850393700920 ) ) ;
#8668=CARTESIAN_POINT ( 'NONE',  ( 0.3929158813954871654, 0.2268989272875732710, -1.934055118110236338 ) ) ;
#8701=AXIS2_PLACEMENT_3D ( 'NONE', #3175, #1088, #20709 ) ;
#8708=CARTESIAN_POINT ( 'NONE',  ( 0.3145317858139327627, 0.4092783051644230397, 1.766732283464566899 ) ) ;
#8710=CARTESIAN_POINT ( 'NONE',  ( 0.1327036767659630079, 0.4954415918530855056, 1.766732283464566899 ) ) ;
#8716=CARTESIAN_POINT ( 'NONE',  ( 0.3574975638436101444, 0.02339816079119100625, -3.115157480314960647 ) ) ;
#8722=CARTESIAN_POINT ( 'NONE',  ( 0.3007905576423883232, 0.1482986320106616795, 1.953740157480315043 ) ) ;
#8724=ORIENTED_EDGE ( 'NONE', *, *, #22982, .F. ) ;
#8738=DIRECTION ( 'NONE',  ( -0.000000000000000000, -1.000000000000000000, -0.000000000000000000 ) ) ;
#8746=DIRECTION ( 'NONE',  ( 0.000000000000000000, 0.000000000000000000, -1.000000000000000000 ) ) ;
#8749=CARTESIAN_POINT ( 'NONE',  ( 0.07874015748031489015, 0.1968503937007873850, -3.272637795275590733 ) ) ;
#8750=ORIENTED_EDGE ( 'NONE', *, *, #7458, .T. ) ;
#8759=CARTESIAN_POINT ( 'NONE',  ( 0.1429116519061227053, -0.5335524835332334792, 0.9202755905511811330 ) ) ;
#8772=CARTESIAN_POINT ( 'NONE',  ( -0.3482225189666627863, 0.4539000224941008854, 0.9399606299212598381 ) ) ;
#8782=CARTESIAN_POINT ( 'NONE',  ( -0.2860025288253731923, -0.4954757973265057069, 0.9399606299212601712 ) ) ;
#8801=CARTESIAN_POINT ( 'NONE',  ( -0.4763861460130343062, -0.1275996891957688339, -1.569881889763779625 ) ) ;
#8804=CARTESIAN_POINT ( 'NONE',  ( -0.4585215200179055817, -0.03001016326912892690, -1.928289503579156516 ) ) ;
#8806=EDGE_CURVE ( 'NONE', #22294, #12664, #26679, .T. ) ;
#8829=CARTESIAN_POINT ( 'NONE',  ( -0.3233561589688984661, 0.1867299569291787087, -3.115157480314960647 ) ) ;
#8843=CARTESIAN_POINT ( 'NONE',  ( -0.06699507805369007973, 0.5085118447801436625, 1.766732283464566899 ) ) ;
#8849=CARTESIAN_POINT ( 'NONE',  ( 0.1200583359873108324, 0.3535721684717922364, -3.115157480314960647 ) ) ;
#8850=AXIS2_PLACEMENT_3D ( 'NONE', #17642, #22161, #24006 ) ;
#8854=CARTESIAN_POINT ( 'NONE',  ( 0.2660793235464212203, 0.2041304421298323901, 1.953740157480315043 ) ) ;
#8858=ORIENTED_EDGE ( 'NONE', *, *, #4888, .F. ) ;
#8881=CARTESIAN_POINT ( 'NONE',  ( -0.01288382760289588994, 0.2165354330708661457, -3.174212598425197207 ) ) ;
#8884=CARTESIAN_POINT ( 'NONE',  ( 0.3184623230426910645, -0.1570784101598338978, 1.953740157480315043 ) ) ;
#8894=CARTESIAN_POINT ( 'NONE',  ( 0.07214854559197284023, -0.5476281405333195407, 0.9202755905511811330 ) ) ;
#8914=CARTESIAN_POINT ( 'NONE',  ( 0.5118124425185632820, 0.03359157810808711259, -1.550196850393701142 ) ) ;
#8920=LINE ( 'NONE', #10911, #3799 ) ;
#8936=DIRECTION ( 'NONE',  ( 1.000000000000000000, 0.000000000000000000, 0.000000000000000000 ) ) ;
#8938=CARTESIAN_POINT ( 'NONE',  ( 0.3979194638820595098, 0.2297883689023132170, -1.928289503579157183 ) ) ;
#8952=CARTESIAN_POINT ( 'NONE',  ( 0.3543307086614173596, 0.000000000000000000, 1.953740157480315043 ) ) ;
#8959=DIRECTION ( 'NONE',  ( 0.000000000000000000, 0.000000000000000000, -1.000000000000000000 ) ) ;
#8964=CARTESIAN_POINT ( 'NONE',  ( -0.1200583359873055728, 0.3535721684717720859, -3.115157480314960647 ) ) ;
#8972=CARTESIAN_POINT ( 'NONE',  ( 0.1339654526248285071, 0.4984899526255159308, 1.766732283464566899 ) ) ;
#8974=CARTESIAN_POINT ( 'NONE',  ( -0.3121994997598287469, 0.4069448477556107946, 1.766732283464566899 ) ) ;
#8975=CARTESIAN_POINT ( 'NONE',  ( -0.2268096725222598919, -0.4600326175560532915, 1.747047244094488194 ) ) ;
#8982=CARTESIAN_POINT ( 'NONE',  ( 0.2272836761397900307, -0.2962590301041579388, -3.115157480314960647 ) ) ;
#8988=CARTESIAN_POINT ( 'NONE',  ( 0.02190250779246093876, -0.3346456692913385988, 1.953740157480315043 ) ) ;
#8991=B_SPLINE_CURVE_WITH_KNOTS ( 'NONE', 2,
 ( #24380, #5026, #13644 ),
 .UNSPECIFIED., .F., .F.,
 ( 3, 3 ),
 ( 0.000000000000000000, 1.000000000000000000 ),
 .UNSPECIFIED. ) ;
#9003=EDGE_CURVE ( 'NONE', #23265, #21357, #14570, .T. ) ;
#9006=CARTESIAN_POINT ( 'NONE',  ( -0.3149606299212598381, 3.857155272905049219E-17, -3.666338582670846780 ) ) ;
#9024=DIRECTION ( 'NONE',  ( 0.000000000000000000, 0.000000000000000000, 1.000000000000000000 ) ) ;
#9026=CARTESIAN_POINT ( 'NONE',  ( -0.1429116519061139623, 0.5335524835332415838, 0.9399606299212598381 ) ) ;
#9044=CARTESIAN_POINT ( 'NONE',  ( -0.4954156765914849991, -0.2860899518037616773, 0.9399606299212598381 ) ) ;
#9045=CARTESIAN_POINT ( 'NONE',  ( -0.4472135058506043759, -0.2577577458591217008, 1.766732283464566677 ) ) ;
#9046=CARTESIAN_POINT ( 'NONE',  ( -0.09842519685039366473, 0.1968503937007873850, -3.548228346456693050 ) ) ;
#9068=EDGE_LOOP ( 'NONE', ( #15802, #5351 ) ) ;
#9070=CARTESIAN_POINT ( 'NONE',  ( 0.3707612262533033776, -0.3252100150720387273, -1.550196850393700920 ) ) ;
#9071=CARTESIAN_POINT ( 'NONE',  ( -0.1188866373884876204, 0.4438564651657459503, -1.928289503579154740 ) ) ;
#9078=FACE_OUTER_BOUND ( 'NONE', #21718, .T. ) ;
#9089=CARTESIAN_POINT ( 'NONE',  ( -0.4382752542996525835, 0.1173917140416343985, -1.934055118110236338 ) ) ;
#9095=CARTESIAN_POINT ( 'NONE',  ( 0.3384212623783103835, 0.1668516812751408562, -3.100567304031765392 ) ) ;
#9107=CARTESIAN_POINT ( 'NONE',  ( -0.3346456692913385988, 0.000000000000000000, 2.504921259842519898 ) ) ;
#9109=CARTESIAN_POINT ( 'NONE',  ( 0.5085118447801426633, -0.06699507805369582514, 1.766732283464566899 ) ) ;
#9113=CARTESIAN_POINT ( 'NONE',  ( -0.02438677169350799909, 0.3726024258163779246, -3.115157480314960647 ) ) ;
#9117=CARTESIAN_POINT ( 'NONE',  ( 0.1677079028045370679, 0.2904160862623488826, 1.953740157480315043 ) ) ;
#9126=CARTESIAN_POINT ( 'NONE',  ( -0.06294778803469826267, 0.1968503937007874127, -3.596639928719705281 ) ) ;
#9135=FACE_OUTER_BOUND ( 'NONE', #8112, .T. ) ;
#9137=CARTESIAN_POINT ( 'NONE',  ( -0.2669480828848088128, -0.2341512108694275007, 1.953740157480315043 ) ) ;
#9158=CARTESIAN_POINT ( 'NONE',  ( 0.4382482975805209735, 0.3362148458989007715, 0.9399606299212598381 ) ) ;
#9166=CARTESIAN_POINT ( 'NONE',  ( 0.3346456692913385988, 0.000000000000000000, 1.953740157480315043 ) ) ;
#9170=CARTESIAN_POINT ( 'NONE',  ( -0.3175540113612215221, -0.1078280746903921422, 1.953740157480315043 ) ) ;
#9176=CARTESIAN_POINT ( 'NONE',  ( 0.5118110236220473341, 6.402768735150616610E-17, -1.550196850393700920 ) ) ;
#9179=AXIS2_PLACEMENT_3D ( 'NONE', #15657, #5040, #4903 ) ;
#9193=CARTESIAN_POINT ( 'NONE',  ( -0.4585215200179055817, 2.807634559150536355E-17, -1.928289503579156516 ) ) ;
#9200=CARTESIAN_POINT ( 'NONE',  ( -0.2031943647053778002, -0.4121342552748231136, -1.928289503579173614 ) ) ;
#9208=( LENGTH_UNIT ( ) NAMED_UNIT ( * ) SI_UNIT ( $, .METRE. ) ) ;
#9219=CARTESIAN_POINT ( 'NONE',  ( 0.3411003281197161341, 0.2991932138496539162, -1.934055118110236338 ) ) ;
#9225=CARTESIAN_POINT ( 'NONE',  ( 0.2836590635674658412, -0.2488091035916875082, -3.100567304031767168 ) ) ;
#9229=ORIENTED_EDGE ( 'NONE', *, *, #12850, .F. ) ;
#9239=CARTESIAN_POINT ( 'NONE',  ( -0.06699507805371239522, -0.5085118447801502128, 1.747047244094488194 ) ) ;
#9241=CARTESIAN_POINT ( 'NONE',  ( 0.1200583359873109851, -0.3535721684717733071, -3.115157480314960647 ) ) ;
#9244=CARTESIAN_POINT ( 'NONE',  ( -0.2660793235464293804, -0.2041304421298503202, 1.953740157480315043 ) ) ;
#9246=ORIENTED_EDGE ( 'NONE', *, *, #14281, .T. ) ;
#9259=CARTESIAN_POINT ( 'NONE',  ( -0.3574975638436101444, 0.02339816079122976691, -3.115157480314960647 ) ) ;
#9264=CARTESIAN_POINT ( 'NONE',  ( -0.01288382813972197179, 0.2165354330708661734, -3.174212598425197207 ) ) ;
#9265=CARTESIAN_POINT ( 'NONE',  ( -0.09187177619658884464, -0.3429980251342297226, 1.953740157480315043 ) ) ;
#9268=CARTESIAN_POINT ( 'NONE',  ( -2.685748425196850164E-17, 0.000000000000000000, -1.934055118110236338 ) ) ;
#9278=CARTESIAN_POINT ( 'NONE',  ( 0.1570773243920708662, -0.3184597017670454666, 1.953740157480315043 ) ) ;
#9286=CARTESIAN_POINT ( 'NONE',  ( 0.5417097841048850171, 0.1839420097223152528, 0.9399606299212598381 ) ) ;
#9290=DIRECTION ( 'NONE',  ( 0.000000000000000000, 0.000000000000000000, -1.000000000000000000 ) ) ;
#9291=PRODUCT_DEFINITION_FORMATION_WITH_SPECIFIED_SOURCE ( 'ANY', '', #14568, .NOT_KNOWN. ) ;
#9303=CARTESIAN_POINT ( 'NONE',  ( 0.3362336590883683307, 0.1141709026133588128, 1.953740157480315043 ) ) ;
#9317=CARTESIAN_POINT ( 'NONE',  ( 0.5118110236220472231, 6.267877318470705905E-17, 1.914370078775489148 ) ) ;
#9318=CARTESIAN_POINT ( 'NONE',  ( 0.08600259748440255980, 0.1968503937007873850, -3.597797143241302287 ) ) ;
#9323=B_SPLINE_CURVE_WITH_KNOTS ( 'NONE', 3,
 ( #27599, #21518, #5848, #84, #14769, #25327, #10347, #2013, #10197, #10624, #23079, #8514, #27742, #17134, #8242, #16863, #25179, #19105, #18816, #25473, #23224, #6137, #3857, #12617, #3706, #21237, #1875, #10484, #25611, #6266, #25755, #15033, #23646, #4281 ),
 .UNSPECIFIED., .F., .F.,
 ( 4, 2, 2, 2, 2, 2, 2, 2, 2, 2, 2, 2, 2, 2, 2, 2, 4 ),
 ( 0.000000000000000000, 0.03124999999999999306, 0.06249999999999998612, 0.09374999999999997224, 0.1249999999999999722, 0.1562499999999999722, 0.1874999999999999722, 0.2187500000000000000, 0.2500000000000000555, 0.2812500000000000555, 0.3125000000000000555, 0.3437500000000000555, 0.3750000000000000000, 0.4062500000000000000, 0.4375000000000000000, 0.4687500000000000000, 0.5000000000000000000 ),
 .UNSPECIFIED. ) ;
#9329=CARTESIAN_POINT ( 'NONE',  ( 0.2660793235464269380, 0.2041304421298361926, 1.973425196850393970 ) ) ;
#9331=CARTESIAN_POINT ( 'NONE',  ( -0.3382184156749268311, 0.3855916753034290823, -1.550196850393700920 ) ) ;
#9333=CARTESIAN_POINT ( 'NONE',  ( -0.4351030398461813720, -0.1477428134820238381, -1.928289503579156294 ) ) ;
#9335=CARTESIAN_POINT ( 'NONE',  ( -0.4954197419817281123, 0.2442565704126535286, 0.9399606299212598381 ) ) ;
#9339=CARTESIAN_POINT ( 'NONE',  ( -0.2796934465393912106, 0.3645739570812651653, -1.928289503579152742 ) ) ;
#9340=CARTESIAN_POINT ( 'NONE',  ( 0.1585706980422248169, 0.4669911931914899617, -1.569881889763779625 ) ) ;
#9354=CARTESIAN_POINT ( 'NONE',  ( 0.1570784101600835037, 0.3184623230425051577, 1.953740157480315043 ) ) ;
#9356=CARTESIAN_POINT ( 'NONE',  ( 0.3411003281197156900, -0.2991932138496291582, -1.934055118110236338 ) ) ;
#9364=EDGE_CURVE ( 'NONE', #10805, #25987, #10495, .T. ) ;
#9365=DIRECTION ( 'NONE',  ( 0.000000000000000000, 0.000000000000000000, -1.000000000000000000 ) ) ;
#9367=CARTESIAN_POINT ( 'NONE',  ( 0.2488091035917030791, 0.2836590635674509642, -3.100567304031764948 ) ) ;
#9371=CARTESIAN_POINT ( 'NONE',  ( -0.3535065162672771932, 0.2712027394948494652, -1.934055118110236338 ) ) ;
#9378=CARTESIAN_POINT ( 'NONE',  ( -0.3382184156732166436, 0.3855916753051391033, 1.747047244094488194 ) ) ;
#9382=CARTESIAN_POINT ( 'NONE',  ( -0.3233561589689049609, -0.1867299569291588357, -3.115157480314960647 ) ) ;
#9385=EDGE_CURVE ( 'NONE', #19099, #13505, #13802, .T. ) ;
#9399=DIRECTION ( 'NONE',  ( -1.000000000000000000, 0.000000000000000000, 0.000000000000000000 ) ) ;
#9403=CARTESIAN_POINT ( 'NONE',  ( 0.09586345242798377519, 0.2165354330708661734, -3.246875208232353760 ) ) ;
#9404=CARTESIAN_POINT ( 'NONE',  ( 0.08759279594700326854, -0.3259357382551449911, 1.973425196850394192 ) ) ;
#9405=CARTESIAN_POINT ( 'NONE',  ( 0.2341512108694336625, 0.2669480828848126985, 1.953740157480315043 ) ) ;
#9412=DIRECTION ( 'NONE',  ( -1.000000000000000000, 0.000000000000000000, 0.000000000000000000 ) ) ;
#9413=CARTESIAN_POINT ( 'NONE',  ( -0.06957181182498481387, 0.5280699926563169333, 1.747047244094488194 ) ) ;
#9415=CARTESIAN_POINT ( 'NONE',  ( -0.07874015747999536796, 0.1968503937007873850, -3.262328874726528660 ) ) ;
#9424=ORIENTED_EDGE ( 'NONE', *, *, #15837, .F. ) ;
#9426=CARTESIAN_POINT ( 'NONE',  ( 0.3707612262533184766, 0.3252100150720236282, -1.569881889763779625 ) ) ;
#9429=CARTESIAN_POINT ( 'NONE',  ( -0.5511811023622048555, 0.000000000000000000, 0.9399606299212598381 ) ) ;
#9431=FACE_BOUND ( 'NONE', #27164, .T. ) ;
#9432=CIRCLE ( 'NONE', #21181, 0.4724409448465559103 ) ;
#9433=CARTESIAN_POINT ( 'NONE',  ( 0.000000000000000000, 0.000000000000000000, 1.747047244094488194 ) ) ;
#9442=CARTESIAN_POINT ( 'NONE',  ( -0.02190250779245987017, -0.3346456692913385988, 1.953740157480315043 ) ) ;
#9463=CARTESIAN_POINT ( 'NONE',  ( 0.06048688226684503788, 0.2165354330708661457, -3.626935712454915972 ) ) ;
#9468=CARTESIAN_POINT ( 'NONE',  ( -0.5118110236220472231, -0.03359871295763396104, -1.550196850393701142 ) ) ;
#9473=CARTESIAN_POINT ( 'NONE',  ( -0.3346456692913385988, -0.02190250779246036283, 1.973425196850393970 ) ) ;
#9474=CARTESIAN_POINT ( 'NONE',  ( -0.4669911931914537129, -0.1585706980422384171, -1.550196850393700920 ) ) ;
#9475=CARTESIAN_POINT ( 'NONE',  ( -0.4816145447621891784, 0.2775852647713620280, 0.9202755905511810219 ) ) ;
#9478=CARTESIAN_POINT ( 'NONE',  ( -0.4382482975805320757, -0.3362148458988418187, 0.9202755905511811330 ) ) ;
#9483=CARTESIAN_POINT ( 'NONE',  ( 0.2466292688015061796, 0.4270824798167727199, -1.569881889763779625 ) ) ;
#9492=CARTESIAN_POINT ( 'NONE',  ( 0.000000000000000000, 0.000000000000000000, -1.550196850393700920 ) ) ;
#9495=CARTESIAN_POINT ( 'NONE',  ( -0.09193072188187405291, 0.3429848536918321256, 1.953740157480315043 ) ) ;
#9498=CARTESIAN_POINT ( 'NONE',  ( 0.1458850421962362143, -0.4296318976989931815, -1.934055118110236338 ) ) ;
#9506=CARTESIAN_POINT ( 'NONE',  ( 0.3740848232703729015, -0.04928467685644277729, -3.100567304031765392 ) ) ;
#9510=CARTESIAN_POINT ( 'NONE',  ( -0.4218945342797526532, -0.1432577568504610210, -1.934055118110236338 ) ) ;
#9517=ORIENTED_EDGE ( 'NONE', *, *, #5794, .F. ) ;
#9522=CARTESIAN_POINT ( 'NONE',  ( 0.4600326175560556230, -0.2268096725222457644, 1.766732283464566899 ) ) ;
#9525=CARTESIAN_POINT ( 'NONE',  ( 0.2836590635674519634, 0.2488091035917033567, -3.100567304031761395 ) ) ;
#9527=CARTESIAN_POINT ( 'NONE',  ( -0.4585215200179055817, 0.000000000000000000, -1.928289503579156516 ) ) ;
#9535=CARTESIAN_POINT ( 'NONE',  ( 0.4446020952038907681, -0.02909913904662010317, -1.934055118110236338 ) ) ;
#9538=CARTESIAN_POINT ( 'NONE',  ( 0.04841158226352236527, 0.1968503937007874127, -3.611176134491095091 ) ) ;
#9542=CARTESIAN_POINT ( 'NONE',  ( 0.3346456692913385988, 0.04380501567505457050, 1.973425196850394192 ) ) ;
#9548=CARTESIAN_POINT ( 'NONE',  ( -0.3520466617656974884, -0.04638120790932648285, 1.953740157480315043 ) ) ;
#9556=CARTESIAN_POINT ( 'NONE',  ( -0.4004221243553298115, -0.3512268162760094348, 1.747047244094488194 ) ) ;
#9565=CARTESIAN_POINT ( 'NONE',  ( 0.03220957031753916844, -0.4921259842519686289, -1.569881889763779625 ) ) ;
#9567=CARTESIAN_POINT ( 'NONE',  ( -0.5131133041953912510, 0.2529800193559492705, 0.9399606299212598381 ) ) ;
#9583=CARTESIAN_POINT ( 'NONE',  ( 0.3543307086614173596, 0.000000000000000000, 1.953740157480315043 ) ) ;
#9590=DIRECTION ( 'NONE',  ( 0.000000000000000000, 0.000000000000000000, 1.000000000000000000 ) ) ;
#9604=CARTESIAN_POINT ( 'NONE',  ( 0.02576258753917241504, 0.1968503937008544147, -3.644091798679202299 ) ) ;
#9619=CARTESIAN_POINT ( 'NONE',  ( 0.09842519685039358146, 0.2991866959364303802, -3.548228346456693050 ) ) ;
#9620=CARTESIAN_POINT ( 'NONE',  ( -0.4921259842519685179, 0.000000000000000000, -1.550196850393700920 ) ) ;
#9623=CARTESIAN_POINT ( 'NONE',  ( 0.4152525734086276454, 0.3642352168757554964, 0.9202755905511811330 ) ) ;
#9646=CARTESIAN_POINT ( 'NONE',  ( 0.4296318976989619842, -0.1458850421962461508, -1.934055118110236338 ) ) ;
#9659=CARTESIAN_POINT ( 'NONE',  ( -0.2488091035917009419, 0.2836590635674538508, -3.100567304031763172 ) ) ;
#9666=CARTESIAN_POINT ( 'NONE',  ( 0.3535065162672720307, 0.2712027394948698378, -1.934055118110236338 ) ) ;
#9667=CARTESIAN_POINT ( 'NONE',  ( -0.4438564651657478377, 0.1188866373884873845, -1.928289503579152742 ) ) ;
#9673=CARTESIAN_POINT ( 'NONE',  ( 0.4441657790107856330, -0.2564944395515579845, 1.766732283464566899 ) ) ;
#9677=CARTESIAN_POINT ( 'NONE',  ( -0.2993674444872274076, -0.2296683860596782090, -3.100567304031764060 ) ) ;
#9687=CARTESIAN_POINT ( 'NONE',  ( -0.1432577568504724008, -0.4218945342797531528, -1.934055118110236338 ) ) ;
#9700=CARTESIAN_POINT ( 'NONE',  ( -0.3346456692913385988, 2.134256245050205639E-17, 1.973425196850393970 ) ) ;
#9701=CARTESIAN_POINT ( 'NONE',  ( 0.02319089060378217229, -0.3543307086614173596, 1.953740157480315043 ) ) ;
#9705=LINE ( 'NONE', #13955, #10999 ) ;
#9710=CARTESIAN_POINT ( 'NONE',  ( 0.4004221243553300891, 0.3512268162760394108, 1.747047244094488194 ) ) ;
#9712=CARTESIAN_POINT ( 'NONE',  ( 0.3121994997598087074, 0.4069448477555728250, 1.747047244094488194 ) ) ;
#9715=CARTESIAN_POINT ( 'NONE',  ( -0.2180698645301862859, 0.2842490391651604775, -3.115157480314960647 ) ) ;
#9723=CARTESIAN_POINT ( 'NONE',  ( 0.1275996891957757451, -0.4763861460130329184, -1.569881889763779625 ) ) ;
#9738=CARTESIAN_POINT ( 'NONE',  ( -0.1482986320106521871, -0.3007905576423956506, 1.953740157480315043 ) ) ;
#9767=CARTESIAN_POINT ( 'NONE',  ( -0.1482986320106401412, 0.3007905576423888783, 1.973425196850393970 ) ) ;
#9768=CARTESIAN_POINT ( 'NONE',  ( 0.4441657790094327707, -0.2564944395535760369, -1.550196850393700920 ) ) ;
#9769=FACE_OUTER_BOUND ( 'NONE', #16732, .T. ) ;
#9771=CARTESIAN_POINT ( 'NONE',  ( -0.03607471876262562105, -0.5511811023622046335, 0.9202755905511811330 ) ) ;
#9778=CARTESIAN_POINT ( 'NONE',  ( -0.06441834428466612639, 0.4889536969035325753, -1.569881889763779625 ) ) ;
#9780=CARTESIAN_POINT ( 'NONE',  ( 0.3289909311256231095, -0.1896185148830507317, -3.100567304031763172 ) ) ;
#9784=CARTESIAN_POINT ( 'NONE',  ( -0.06947618719668695320, 0.5280904602948609528, 1.747047244094488416 ) ) ;
#9785=SURFACE_SIDE_STYLE ('',( #27030 ) ) ;
#9794=CARTESIAN_POINT ( 'NONE',  ( 0.2991932138496291582, 0.3411003281196904324, -1.934055118110236338 ) ) ;
#9797=CARTESIAN_POINT ( 'NONE',  ( 0.09842519685039370636, 0.2991866959364303802, -3.272637795275590733 ) ) ;
#9804=CARTESIAN_POINT ( 'NONE',  ( -0.3765118517642104257, -0.02464264302297883638, -3.100567304031763172 ) ) ;
#9807=CARTESIAN_POINT ( 'NONE',  ( -0.2268989272875546748, 0.3929158813954828355, -1.934055118110236338 ) ) ;
#9821=CARTESIAN_POINT ( 'NONE',  ( -0.1886891683788906593, -0.3267488823401751841, -3.100567304031762284 ) ) ;
#9828=CARTESIAN_POINT ( 'NONE',  ( 0.4218945342797225662, -0.1432577568504558585, -1.934055118110236338 ) ) ;
#9830=ORIENTED_EDGE ( 'NONE', *, *, #14866, .T. ) ;
#9835=CARTESIAN_POINT ( 'NONE',  ( 0.5368353335967094297, -0.1442704874421229522, 0.9202755905511812440 ) ) ;
#9837=CARTESIAN_POINT ( 'NONE',  ( 0.2676050456844303316, 0.2056553984168022209, 1.973425196850393970 ) ) ;
#9840=CARTESIAN_POINT ( 'NONE',  ( -0.09842519685039378963, 0.2165354330708661457, -3.259753967135868624 ) ) ;
#9850=CARTESIAN_POINT ( 'NONE',  ( 0.03478633594543729946, 0.5314960629921260393, 1.747047244094488194 ) ) ;
#9862=EDGE_LOOP ( 'NONE', ( #7543, #20401, #18259, #17249 ) ) ;
#9864=CARTESIAN_POINT ( 'NONE',  ( 0.4889536969035315206, 0.06441834428467128892, -1.569881889763779625 ) ) ;
#9896=AXIS2_PLACEMENT_3D ( 'NONE', #23491, #25593, #13140 ) ;
#9897=CARTESIAN_POINT ( 'NONE',  ( 0.01030706208231913640, 0.1968503937007873850, -3.626968503937007871 ) ) ;
#9909=CARTESIAN_POINT ( 'NONE',  ( -0.2564944395535628252, -0.4441657790094413749, -1.550196850393700920 ) ) ;
#9911=CARTESIAN_POINT ( 'NONE',  ( 0.5511811023622047445, 0.07214943758244277139, 0.9202755905511812440 ) ) ;
#9914=CARTESIAN_POINT ( 'NONE',  ( -0.3642352168757361786, -0.4152525734086467968, 0.9202755905511811330 ) ) ;
#9919=CARTESIAN_POINT ( 'NONE',  ( 0.04928528614549709808, -0.3765118517642105367, -3.100567304031763616 ) ) ;
#9943=CARTESIAN_POINT ( 'NONE',  ( 0.1151354519024844064, -0.3392634445560540057, -3.115157480314960203 ) ) ;
#9946=CARTESIAN_POINT ( 'NONE',  ( 0.2228126397719810137, -0.3858397471888643793, -1.934055118110236338 ) ) ;
#9973=EDGE_CURVE ( 'NONE', #21357, #23265, #23632, .T. ) ;
#9974=CARTESIAN_POINT ( 'NONE',  ( 0.3551931031211721379, 0.04679574315772513232, -3.115157480314960647 ) ) ;
#9976=CARTESIAN_POINT ( 'NONE',  ( 0.04380501567505448723, 0.3346456692913385988, 1.973425196850394192 ) ) ;
#9979=FACE_OUTER_BOUND ( 'NONE', #16010, .T. ) ;
#9981=DIRECTION ( 'NONE',  ( 0.000000000000000000, 0.000000000000000000, -1.000000000000000000 ) ) ;
#9987=CARTESIAN_POINT ( 'NONE',  ( -0.4301590433675065994, 0.3771696032820260336, 0.9399606299212601712 ) ) ;
#9992=CARTESIAN_POINT ( 'NONE',  ( 0.3512268162760394108, 0.4004221243553300891, 1.747047244094488194 ) ) ;
#9993=CARTESIAN_POINT ( 'NONE',  ( -0.09842519685039370636, 0.2165354330708661457, -3.272637795275590733 ) ) ;
#9994=CARTESIAN_POINT ( 'NONE',  ( -0.4069448477556107946, -0.3121994997598286914, 1.766732283464566899 ) ) ;
#10001=CARTESIAN_POINT ( 'NONE',  ( -0.4303822302054170490, 0.1152775731717081975, -1.934055118110236338 ) ) ;
#10004=VERTEX_POINT ( 'NONE', #11744 ) ;
#10008=CARTESIAN_POINT ( 'NONE',  ( -0.4270824798167697223, -0.2466292688015108703, -1.569881889763779625 ) ) ;
#10016=B_SPLINE_SURFACE_WITH_KNOTS ( 'NONE', 2, 3, ( 
 ( #13270, #4780, #21894, #7464, #16092, #15942, #22440, #7186, #13976, #2929, #14111, #22722, #27113, #18609, #11992, #3493, #24686, #15805, #18463, #24411, #3350, #20322, #7759, #20607, #5199, #9426, #5057, #18027, #20174, #5500, #13826, #9864, #24976, #1260, #16371, #20465, #5349, #18174, #3064, #22875, #24835, #18323, #24545, #11699, #13678, #979, #9723, #26668, #9565, #26815, #22295, #22585, #3210, #11843, #5637, #1123, #26968, #12125, #11558, #10008, #7616, #7323, #16235, #14267, #836, #20749 ),
 ( #1390, #12411, #21024, #10705, #21169, #14409, #10278, #23017, #2093, #1812, #6341, #3935, #8177, #4217, #19039, #27251, #4077, #12552, #21455, #12823, #6209, #21312, #14702, #17071, #10420, #20885, #23448, #19183, #25688, #3637, #23308, #27391, #16502, #8320, #12265, #14970, #16939, #7898, #23585, #6067, #27814, #3791, #16792, #25549, #8447, #1532, #25120, #10139, #5785, #1671, #8044, #18892, #16652, #5925, #14560, #23157, #25404, #5985, #2282, #18811, #19246, #27738, #4277, #27594, #25322, #23778 ),
 ( #18958, #12470, #8237, #3999, #6402, #23220, #15029, #8099, #12881, #21373, #19386, #21233, #1872, #16709, #12743, #14619, #10480, #3852, #21652, #2009, #25889, #23507, #8380, #4420, #10620, #21083, #21515, #4136, #13024, #1731, #25750, #2152, #6261, #8647, #27876, #10343, #82, #6535, #15167, #16859, #14898, #25469, #6131, #8510, #19100, #16995, #17130, #25607, #6814, #11314, #24036, #4674, #25003, #22903, #27272, #11874, #27703, #23189, #23045, #25435, #6233, #6101, #3820, #1700, #10307, #8207 ) ),
 .UNSPECIFIED., .F., .T., .F.,
 ( 3, 3 ),
 ( 4, 2, 2, 2, 2, 2, 2, 2, 2, 2, 2, 2, 2, 2, 2, 2, 2, 2, 2, 2, 2, 2, 2, 2, 2, 2, 2, 2, 2, 2, 2, 2, 4 ),
 ( 0.000000000000000000, 1.000000000000000000 ),
 ( 0.000000000000000000, 0.1963495408493620697, 0.3926990816987241395, 0.5890486225480862092, 0.7853981633974482790, 0.9817477042468103487, 1.178097245096172418, 1.374446785945534488, 1.570796326794896558, 1.767145867644258628, 1.963495408493620697, 2.159844949342982545, 2.356194490192344837, 2.552544031041707129, 2.748893571891068976, 2.945243112740430824, 3.141592653589793116, 3.337942194439155408, 3.534291735288517255, 3.730641276137879103, 3.926990816987241395, 4.123340357836603687, 4.319689898685965090, 4.516039439535327382, 4.712388980384689674, 4.908738521234051966, 5.105088062083414258, 5.301437602932775661, 5.497787143782137953, 5.694136684631500245, 5.890486225480861648, 6.086835766330223940, 6.283185307179586232 ),
 .UNSPECIFIED. ) ;
#10026=FACE_OUTER_BOUND ( 'NONE', #2017, .T. ) ;
#10030=VERTEX_POINT ( 'NONE', #2830 ) ;
#10045=CARTESIAN_POINT ( 'NONE',  ( 0.2211428102655695338, -0.2521176338356630464, 1.973425196850393970 ) ) ;
#10049=CARTESIAN_POINT ( 'NONE',  ( -0.4152525734085961151, -0.3642352168756899933, 0.9399606299212598381 ) ) ;
#10056=CARTESIAN_POINT ( 'NONE',  ( 0.07669076177804119709, 0.1968503937007873850, -3.252027725244190481 ) ) ;
#10057=CARTESIAN_POINT ( 'NONE',  ( 0.5314960629921261503, 0.03490580340508878110, 1.747047244094489304 ) ) ;
#10068=AXIS2_PLACEMENT_3D ( 'NONE', #885, #22487, #7509 ) ;
#10083=CARTESIAN_POINT ( 'NONE',  ( 0.3392608232658640977, -0.1151343661288334597, -3.115157480314961091 ) ) ;
#10085=CARTESIAN_POINT ( 'NONE',  ( -0.1432577568504724008, -0.4218945342797531528, -1.934055118110236338 ) ) ;
#10086=CARTESIAN_POINT ( 'NONE',  ( -0.4527559054764770385, -0.02963280468031422032, -1.934055118110236338 ) ) ;
#10093=CARTESIAN_POINT ( 'NONE',  ( 0.5314960629921260393, 0.000000000000000000, 1.747047244094488194 ) ) ;
#10098=CARTESIAN_POINT ( 'NONE',  ( 0.3765118517642104257, -0.02464264302293790732, -3.100567304031763172 ) ) ;
#10100=CARTESIAN_POINT ( 'NONE',  ( 0.000000000000000000, 0.000000000000000000, -1.550196850393700920 ) ) ;
#10102=CARTESIAN_POINT ( 'NONE',  ( -0.2161381151962937508, 0.2817310484609270027, 1.953740157480315043 ) ) ;
#10106=CARTESIAN_POINT ( 'NONE',  ( 0.2762247810518927427, -0.4783323773986943306, 0.9399606299212598381 ) ) ;
#10112=ADVANCED_FACE ( 'NONE', ( #22760, #3385 ), #12593, .T. ) ;
#10113=VECTOR ( 'NONE', #4270, 39.37007874015748143 ) ;
#10115=CARTESIAN_POINT ( 'NONE',  ( -0.1151913129404333325, 0.3392387706403566239, -3.115157480314960647 ) ) ;
#10125=CYLINDRICAL_SURFACE ( 'NONE', #6305, 0.5905511811023621549 ) ;
#10128=CARTESIAN_POINT ( 'NONE',  ( 0.2663596103035382745, -0.4612490782035122416, 1.747047244094488194 ) ) ;
#10130=CARTESIAN_POINT ( 'NONE',  ( 0.5085118447801136865, 0.06699507805368522251, 1.747047244094488194 ) ) ;
#10135=CARTESIAN_POINT ( 'NONE',  ( 0.4465874321618643061, -0.1200170377978880404, -1.928289503579156960 ) ) ;
#10137=CARTESIAN_POINT ( 'NONE',  ( 0.2211428102655695338, -0.2521176338356630464, 1.973425196850393970 ) ) ;
#10139=CARTESIAN_POINT ( 'NONE',  ( 0.06441834428465775808, -0.4889536969034878333, -1.550196850393700920 ) ) ;
#10141=VERTEX_POINT ( 'NONE', #8363 ) ;
#10173=CARTESIAN_POINT ( 'NONE',  ( -0.09842519685039385902, 0.2165354330708661457, -3.548228346456693050 ) ) ;
#10176=CARTESIAN_POINT ( 'NONE',  ( 0.3122781343789127195, -0.4068940122751822930, -1.550196850393700476 ) ) ;
#10178=CARTESIAN_POINT ( 'NONE',  ( 0.2211428102655656758, 0.2521176338356670432, 1.953740157480315043 ) ) ;
#10179=CARTESIAN_POINT ( 'NONE',  ( 0.4069448477569521661, 0.3121994997578569353, -1.550196850393700920 ) ) ;
#10182=CARTESIAN_POINT ( 'NONE',  ( 0.1775991818008583745, 0.5230301363771922007, 0.9399606299212598381 ) ) ;
#10197=CARTESIAN_POINT ( 'NONE',  ( 0.4004902621173889732, -0.3511566718594057446, 1.747047244094488416 ) ) ;
#10198=CARTESIAN_POINT ( 'NONE',  ( -0.2268967137093978459, 0.4599980997182848141, -1.550196850393700476 ) ) ;
#10214=CARTESIAN_POINT ( 'NONE',  ( 0.09275248786854008165, -0.3460502918090608282, -3.115157480314960647 ) ) ;
#10216=EDGE_LOOP ( 'NONE', ( #20135, #5151 ) ) ;
#10217=CARTESIAN_POINT ( 'NONE',  ( -0.2268989272875881757, -0.3929158813954942153, -1.934055118110236338 ) ) ;
#10224=CARTESIAN_POINT ( 'NONE',  ( -0.1712563538833044852, 0.5043504886477827576, 1.747047244094488194 ) ) ;
#10233=ADVANCED_FACE ( 'NONE', ( #1572 ), #4173, .T. ) ;
#10234=CARTESIAN_POINT ( 'NONE',  ( 0.2161381151963039093, -0.2817310484609168442, 1.953740157480315043 ) ) ;
#10239=CARTESIAN_POINT ( 'NONE',  ( 0.1429116519061152946, -0.5335524835331961757, 0.9399606299212598381 ) ) ;
#10244=CARTESIAN_POINT ( 'NONE',  ( 0.3460635936745020680, -0.09269288654273737105, -3.115157480314960647 ) ) ;
#10245=CARTESIAN_POINT ( 'NONE',  ( 0.4407612517155324316, -0.3387265385688509323, 0.9202755905511812440 ) ) ;
#10250=DIRECTION ( 'NONE',  ( -0.000000000000000000, -1.000000000000000000, -0.000000000000000000 ) ) ;
#10257=CARTESIAN_POINT ( 'NONE',  ( 0.1481194149833036655, 0.5525858403826197085, 0.9399606299212600602 ) ) ;
#10265=CARTESIAN_POINT ( 'NONE',  ( -0.4069448477556103505, 0.3121994997598293020, 1.766732283464566899 ) ) ;
#10273=CARTESIAN_POINT ( 'NONE',  ( -0.4446020952038907681, 0.02909913904661337244, -1.934055118110236338 ) ) ;
#10276=CARTESIAN_POINT ( 'NONE',  ( 0.02190250779246093876, -0.3346456692913385433, 1.973425196850393970 ) ) ;
#10278=CARTESIAN_POINT ( 'NONE',  ( -0.4270824798167728864, 0.2466292688015120915, -1.550196850393700920 ) ) ;
#10289=VECTOR ( 'NONE', #8596, 39.37007874015748143 ) ;
#10294=CARTESIAN_POINT ( 'NONE',  ( 0.06002032661671171526, 0.4585215200179057482, -1.928289503579156516 ) ) ;
#10296=ADVANCED_FACE ( 'NONE', ( #12295 ), #25602, .T. ) ;
#10298=CARTESIAN_POINT ( 'NONE',  ( -0.4793172621399190425, 0.1288129352161815067, -1.569881889763779625 ) ) ;
#10302=ORIENTED_EDGE ( 'NONE', *, *, #13330, .T. ) ;
#10307=CARTESIAN_POINT ( 'NONE',  ( -0.5118110236220763110, -0.03349795313034512750, -1.550196850393700920 ) ) ;
#10327=CARTESIAN_POINT ( 'NONE',  ( 0.1078280746903962500, -0.3175540113612315696, 1.973425196850393970 ) ) ;
#10331=CARTESIAN_POINT ( 'NONE',  ( -0.3362148458988341582, -0.4382482975805541692, 0.9399606299212598381 ) ) ;
#10341=CARTESIAN_POINT ( 'NONE',  ( -0.2356229156547619552, 0.4776874499716828870, 1.747047244094488416 ) ) ;
#10343=CARTESIAN_POINT ( 'NONE',  ( 0.4954415918535723939, -0.1327036767636087800, -1.550196850393700920 ) ) ;
#10347=CARTESIAN_POINT ( 'NONE',  ( 0.4613022222206614176, -0.2662775206743260847, 1.747047244094488194 ) ) ;
#10348=ORIENTED_EDGE ( 'NONE', *, *, #19068, .T. ) ;
#10350=VERTEX_POINT ( 'NONE', #22871 ) ;
#10364=CARTESIAN_POINT ( 'NONE',  ( -0.4069519308876702324, -0.2006393256663696334, -1.934055118110236338 ) ) ;
#10370=CARTESIAN_POINT ( 'NONE',  ( 0.2355331214654129424, 0.4777261797697872625, 1.747047244094488194 ) ) ;
#10378=CARTESIAN_POINT ( 'NONE',  ( 0.1153557615288998417, 0.4303681241740018315, -1.934055118110236116 ) ) ;
#10380=CARTESIAN_POINT ( 'NONE',  ( -0.3429980251342297226, 0.09187177619658862260, 1.953740157480315043 ) ) ;
#10385=CARTESIAN_POINT ( 'NONE',  ( 0.4300830224589536899, -0.3772436174784755680, 0.9399606299212598381 ) ) ;
#10393=CARTESIAN_POINT ( 'NONE',  ( 0.09269288654274054906, 0.3460635936744927976, -3.115157480314960647 ) ) ;
#10396=DIRECTION ( 'NONE',  ( 1.000000000000000000, 0.000000000000000000, 0.000000000000000000 ) ) ;
#10404=DIRECTION ( 'NONE',  ( 1.000000000000000000, 0.000000000000000000, 0.000000000000000000 ) ) ;
#10408=CARTESIAN_POINT ( 'NONE',  ( 0.4777261797697372470, -0.2355331214654103889, 1.747047244094488194 ) ) ;
#10413=CARTESIAN_POINT ( 'NONE',  ( 0.3574975638436101444, -0.02339816079119092299, -3.115157480314960647 ) ) ;
#10414=CARTESIAN_POINT ( 'NONE',  ( -0.4006498629591503935, -0.2309201403895324023, -1.928289503579156516 ) ) ;
#10416=CARTESIAN_POINT ( 'NONE',  ( -0.02190250779246035590, 0.3346456692913385988, 1.973425196850393970 ) ) ;
#10418=ORIENTED_EDGE ( 'NONE', *, *, #11791, .F. ) ;
#10420=CARTESIAN_POINT ( 'NONE',  ( 0.3252100150720097504, 0.3707612262533033776, -1.550196850393700920 ) ) ;
#10422=CARTESIAN_POINT ( 'NONE',  ( -0.5511811023622048555, 0.000000000000000000, 0.9399606299212598381 ) ) ;
#10440=CARTESIAN_POINT ( 'NONE',  ( 0.4585215200179055817, -2.840735999735804609E-17, -1.928289503579156516 ) ) ;
#10441=CARTESIAN_POINT ( 'NONE',  ( 0.2478439864030018702, 0.4300129863948118913, -1.569881889763779625 ) ) ;
#10446=CARTESIAN_POINT ( 'NONE',  ( 0.4921259842519685179, 0.000000000000000000, -1.934055118110236338 ) ) ;
#10453=CARTESIAN_POINT ( 'NONE',  ( 0.4152525734086276454, 0.3642352168757554964, 0.9202755905511811330 ) ) ;
#10456=CARTESIAN_POINT ( 'NONE',  ( 0.000000000000000000, 0.000000000000000000, 1.747047244094488194 ) ) ;
#10467=CARTESIAN_POINT ( 'NONE',  ( 0.1078280746903977072, 0.3175540113612247972, 1.953740157480315043 ) ) ;
#10470=CARTESIAN_POINT ( 'NONE',  ( 0.4382482975805214731, -0.3362148458988676314, 0.9399606299212598381 ) ) ;
#10474=CARTESIAN_POINT ( 'NONE',  ( 0.2842139414040969481, 0.2181198385715675259, -3.115157480314960647 ) ) ;
#10480=CARTESIAN_POINT ( 'NONE',  ( -0.03349795313024159921, 0.5118110236220473341, -1.550196850393700920 ) ) ;
#10481=CARTESIAN_POINT ( 'NONE',  ( 0.07462095020297215830, -0.5672055940108892136, 0.9399606299212598381 ) ) ;
#10484=CARTESIAN_POINT ( 'NONE',  ( -0.4613045817967623696, -0.2662790972929528488, 1.747047244094487972 ) ) ;
#10495=CIRCLE ( 'NONE', #25384, 0.2938622683360631593 ) ;
#10503=CARTESIAN_POINT ( 'NONE',  ( 0.4296318976989615401, 0.1458850421962473720, -1.934055118110236338 ) ) ;
#10506=CARTESIAN_POINT ( 'NONE',  ( 0.3726024258163779246, 4.695363739110452099E-17, -3.115157480314960647 ) ) ;
#10507=CARTESIAN_POINT ( 'NONE',  ( 0.5043504886477717664, -0.1712563538833085097, 1.747047244094488194 ) ) ;
#10517=CARTESIAN_POINT ( 'NONE',  ( 0.2227458012931471387, 0.3858827008519146728, -1.934055118110236560 ) ) ;
#10520=CARTESIAN_POINT ( 'NONE',  ( -0.1775730735577452091, -0.3074993854542726335, 1.953740157480315043 ) ) ;
#10525=CARTESIAN_POINT ( 'NONE',  ( 0.5417097841048533757, -0.1839420097223136985, 0.9399606299212598381 ) ) ;
#10533=CARTESIAN_POINT ( 'NONE',  ( 0.09660931395005890876, 0.3606853515406323596, -3.115157480314960647 ) ) ;
#10534=CARTESIAN_POINT ( 'NONE',  ( -0.01288382813972184689, 0.2165354330708661457, -3.646653543307086576 ) ) ;
#10539=ORIENTED_EDGE ( 'NONE', *, *, #11383, .F. ) ;
#10540=CARTESIAN_POINT ( 'NONE',  ( 0.4954734376820387198, 0.2860009521624328754, 0.9399606299212598381 ) ) ;
#10545=CARTESIAN_POINT ( 'NONE',  ( -0.4954415918530846175, -0.1327036767659680039, 1.766732283464566899 ) ) ;
#10549=CARTESIAN_POINT ( 'NONE',  ( -0.3460635936744816399, -0.09269288654274071559, -3.115157480314960647 ) ) ;
#10556=CARTESIAN_POINT ( 'NONE',  ( 0.04380447413659065842, -0.3324885138898235892, 1.973425196850393970 ) ) ;
#10568=CARTESIAN_POINT ( 'NONE',  ( -0.02573449447784514899, 0.3139714872872414464, -3.643448523124805050 ) ) ;
#10577=CARTESIAN_POINT ( 'NONE',  ( -0.09842519685039370636, 0.2165354330708661457, -3.548228346456693050 ) ) ;
#10582=CARTESIAN_POINT ( 'NONE',  ( 0.02576258753921353492, 0.2165354330708661457, -3.176774343053047733 ) ) ;
#10590=CARTESIAN_POINT ( 'NONE',  ( 0.3362148458988273303, 0.4382482975805419012, 0.9202755905511811330 ) ) ;
#10611=CARTESIAN_POINT ( 'NONE',  ( -0.4954156765914823346, 0.2860899518036844058, 0.9399606299212598381 ) ) ;
#10614=CARTESIAN_POINT ( 'NONE',  ( -0.1791101711253741402, 0.3102827802123027667, -3.115157480314961980 ) ) ;
#10620=CARTESIAN_POINT ( 'NONE',  ( 0.3382184156748877513, 0.3855916753034390188, -1.550196850393700920 ) ) ;
#10621=CARTESIAN_POINT ( 'NONE',  ( -0.1838445375782518376, -0.5417516942599310825, 0.9399606299212600602 ) ) ;
#10624=CARTESIAN_POINT ( 'NONE',  ( 0.3511586785139784728, -0.4004922687719658647, 1.747047244094488416 ) ) ;
#10629=CARTESIAN_POINT ( 'NONE',  ( -0.07874186976011487982, 0.3051029058891214230, -3.212186138815604330 ) ) ;
#10640=CARTESIAN_POINT ( 'NONE',  ( -0.06441834428466709783, -0.4889536969035322977, -1.569881889763779625 ) ) ;
#10644=CARTESIAN_POINT ( 'NONE',  ( -0.2006393256663304703, -0.4069519308876202168, -1.934055118110236338 ) ) ;
#10653=CARTESIAN_POINT ( 'NONE',  ( 0.5314960629921260393, -0.03478633594540021801, 1.747047244094488194 ) ) ;
#10665=CARTESIAN_POINT ( 'NONE',  ( -0.3482225189666507403, -0.4539000224941303063, 0.9399606299212598381 ) ) ;
#10672=CARTESIAN_POINT ( 'NONE',  ( -0.1651192144506243575, -0.3349073414798197645, -3.115157480314960647 ) ) ;
#10689=CARTESIAN_POINT ( 'NONE',  ( 0.3242071728275346953, -0.4225965726692721969, 1.747047244094488194 ) ) ;
#10690=CARTESIAN_POINT ( 'NONE',  ( -0.2564944395515788567, -0.4441657790107717552, 1.766732283464566899 ) ) ;
#10697=CARTESIAN_POINT ( 'NONE',  ( 0.1791601451668921319, 0.3102476824511487541, -3.115157480314960647 ) ) ;
#10702=CARTESIAN_POINT ( 'NONE',  ( 0.04380447413659061678, 0.3324885138898235892, 1.973425196850393970 ) ) ;
#10705=CARTESIAN_POINT ( 'NONE',  ( -0.4763861460130593972, 0.1275996891957734969, -1.550196850393700920 ) ) ;
#10717=B_SPLINE_SURFACE_WITH_KNOTS ( 'NONE', 2, 3, ( 
 ( #823, #11412, #26655, #26252, #24676, #13525, #15933, #24535, #22571, #22149, #2777, #5187, #6912, #683, #13816, #22019, #22431, #4771, #15535, #3053, #11689, #20310, #26803, #5336, #24134, #14396, #10265, #14546, #21011, #5773, #18744, #27379, #1520, #8033, #3338, #24826, #18310, #11978, #23006, #9994, #18453, #20453, #1380, #24964, #20596, #23145, #1248, #5626, #27525, #11832, #6057, #20739, #27101, #7747, #16637, #7603, #25251, #1113, #5912, #3627, #3778, #16360, #14254, #14688, #12251, #26956 ),
 ( #20872, #18879, #10130, #12112, #8168, #12397, #16778, #14099, #25391, #3198, #9712, #1659, #16223, #18594, #5487, #22713, #22862, #3484, #27236, #21713, #14825, #19309, #4067, #25673, #8576, #23571, #17467, #9, #26081, #6743, #17194, #10832, #4203, #12809, #2340, #23294, #6601, #25811, #21437, #3920, #6460, #12944, #21574, #19447, #8975, #18119, #6873, #2883, #22470, #18592, #7175, #7601, #16078, #11977, #15931, #13666, #12110, #22430, #13815, #1112, #5483, #22711, #27098, #15796, #20595, #3482 ),
 ( #20736, #24674, #1379, #24963, #26654, #14097, #24399, #1246, #9710, #9992, #5047, #3196, #22283, #22570, #18309, #3337, #9850, #18451, #9413, #13962, #7746, #18016, #5185, #16359, #26954, #966, #5623, #20309, #22861, #14252, #2919, #11548, #20163, #7312, #822, #3052, #5335, #24823, #11688, #11829, #9556, #18162, #26802, #20451, #7449, #16222, #27523, #8032, #14541, #27235, #6054, #25388, #16775, #21153, #10128, #10689, #21434, #18742, #14686, #12250, #10408, #12538, #2075, #19165, #20869, #23002 ) ),
 .UNSPECIFIED., .F., .T., .F.,
 ( 3, 3 ),
 ( 4, 2, 2, 2, 2, 2, 2, 2, 2, 2, 2, 2, 2, 2, 2, 2, 2, 2, 2, 2, 2, 2, 2, 2, 2, 2, 2, 2, 2, 2, 2, 2, 4 ),
 ( 0.000000000000000000, 1.000000000000000000 ),
 ( 0.000000000000000000, 0.1963495408493620697, 0.3926990816987241395, 0.5890486225480862092, 0.7853981633974482790, 0.9817477042468103487, 1.178097245096172418, 1.374446785945534488, 1.570796326794896558, 1.767145867644258628, 1.963495408493620697, 2.159844949342982545, 2.356194490192344837, 2.552544031041707129, 2.748893571891068976, 2.945243112740430824, 3.141592653589793116, 3.337942194439155408, 3.534291735288517255, 3.730641276137879103, 3.926990816987241395, 4.123340357836603687, 4.319689898685965090, 4.516039439535327382, 4.712388980384689674, 4.908738521234051966, 5.105088062083414258, 5.301437602932775661, 5.497787143782137953, 5.694136684631500245, 5.890486225480861648, 6.086835766330223940, 6.283185307179586232 ),
 .UNSPECIFIED. ) ;
#10728=CARTESIAN_POINT ( 'NONE',  ( 0.1200170377978880126, 0.4465874321618644172, -1.928289503579157183 ) ) ;
#10729=EDGE_CURVE ( 'NONE', #22996, #24094, #22545, .T. ) ;
#10732=CARTESIAN_POINT ( 'NONE',  ( 0.08600259748440877705, 0.2165354330708661457, -3.223068998490982384 ) ) ;
#10734=CARTESIAN_POINT ( 'NONE',  ( 0.3362336590883683307, 0.1141709026133588128, 1.953740157480315043 ) ) ;
#10742=CARTESIAN_POINT ( 'NONE',  ( -0.07214854559198564943, -0.5476281405333169872, 0.9202755905511811330 ) ) ;
#10746=DIRECTION ( 'NONE',  ( -0.000000000000000000, -0.000000000000000000, -1.000000000000000000 ) ) ;
#10758=CARTESIAN_POINT ( 'NONE',  ( 0.5131133041954354379, -0.2529800193559368360, 0.9399606299212598381 ) ) ;
#10759=VECTOR ( 'NONE', #16829, 39.37007874015748143 ) ;
#10763=CARTESIAN_POINT ( 'NONE',  ( -0.1151354519025668821, 0.3392634445560395173, -3.115157480314961091 ) ) ;
#10789=CARTESIAN_POINT ( 'NONE',  ( -0.3979194638820524044, 0.2297883689023302312, -1.928289503579153630 ) ) ;
#10798=CARTESIAN_POINT ( 'NONE',  ( -0.2663596103035690277, -0.4612490782034817105, 1.747047244094488194 ) ) ;
#10804=CARTESIAN_POINT ( 'NONE',  ( -0.2712680014834641939, 0.3534612032198612974, -1.934055118110237004 ) ) ;
#10805=VERTEX_POINT ( 'NONE', #5457 ) ;
#10809=CARTESIAN_POINT ( 'NONE',  ( -0.4296318976990082805, 0.1458850421962457622, -1.934055118110236338 ) ) ;
#10813=CARTESIAN_POINT ( 'NONE',  ( -0.5708661417322835607, 0.000000000000000000, 0.9399606299212598381 ) ) ;
#10817=CARTESIAN_POINT ( 'NONE',  ( 0.2962590301041578278, 0.2272836761397798999, -3.115157480314960647 ) ) ;
#10832=CARTESIAN_POINT ( 'NONE',  ( -0.5085118447801413311, 0.06699507805369032953, 1.747047244094488194 ) ) ;
#10837=CARTESIAN_POINT ( 'NONE',  ( -0.2180698645301767380, -0.2842490391651532611, -3.115157480314960647 ) ) ;
#10843=CARTESIAN_POINT ( 'NONE',  ( -0.08676778863011123943, 0.3239425792934299553, 1.953740157480315043 ) ) ;
#10852=EDGE_CURVE ( 'NONE', #13505, #19099, #14110, .T. ) ;
#10860=CARTESIAN_POINT ( 'NONE',  ( -0.4465874321618641951, 0.1200170377978884984, -1.928289503579156960 ) ) ;
#10863=CARTESIAN_POINT ( 'NONE',  ( -0.5314974819112029403, 0.03488411621207041652, 1.747047244094488194 ) ) ;
#10865=CARTESIAN_POINT ( 'NONE',  ( -0.09586345222254787080, 0.1968503937007873850, -3.246875207736363844 ) ) ;
#10868=CARTESIAN_POINT ( 'NONE',  ( 0.3543307086614173596, 0.000000000000000000, 1.953740157480315043 ) ) ;
#10877=CARTESIAN_POINT ( 'NONE',  ( -0.3642352168757361786, -0.4152525734086467968, 0.9202755905511811330 ) ) ;
#10888=CARTESIAN_POINT ( 'NONE',  ( -0.2564173815256688971, -0.4442189740297868839, -1.550196850393701142 ) ) ;
#10896=CARTESIAN_POINT ( 'NONE',  ( -0.5118110236220472231, 6.402768735150616610E-17, 1.747047244094488194 ) ) ;
#10898=CARTESIAN_POINT ( 'NONE',  ( 0.2860899518037616773, -0.4954156765914850546, 0.9399606299212598381 ) ) ;
#10899=CARTESIAN_POINT ( 'NONE',  ( 0.1327957795771031180, -0.4954247181591464044, -1.550196850393700476 ) ) ;
#10909=CARTESIAN_POINT ( 'NONE',  ( -0.3771696032823899092, -0.4301590433674395419, 0.9399606299212597271 ) ) ;
#10911=CARTESIAN_POINT ( 'NONE',  ( -0.4527559054764771496, 5.544660704368294164E-17, -1.934055118110236338 ) ) ;
#10927=CARTESIAN_POINT ( 'NONE',  ( 0.4555658499976260600, 0.06001958459474954211, -1.928289503579140529 ) ) ;
#10951=CARTESIAN_POINT ( 'NONE',  ( 0.5708661417322835607, -0.03736310157557555522, 0.9399606299212598381 ) ) ;
#10953=DIRECTION ( 'NONE',  ( -0.7071067818211401734, 0.000000000000000000, -0.7071067805519547500 ) ) ;
#10956=CARTESIAN_POINT ( 'NONE',  ( -0.3726024258163779246, 0.000000000000000000, -3.115157480314960647 ) ) ;
#10969=CARTESIAN_POINT ( 'NONE',  ( 0.06699507805369657454, 0.5085118447801424413, 1.766732283464566899 ) ) ;
#10975=CARTESIAN_POINT ( 'NONE',  ( 0.2693339498142252042, 0.2362439534887496861, -3.115157480314960647 ) ) ;
#10977=VECTOR ( 'NONE', #8738, 39.37007874015748143 ) ;
#10982=CARTESIAN_POINT ( 'NONE',  ( -0.2041304421298407168, -0.2660793235464189999, 1.953740157480315043 ) ) ;
#10988=ORIENTED_EDGE ( 'NONE', *, *, #18348, .F. ) ;
#10999=VECTOR ( 'NONE', #2914, 39.37007874015748143 ) ;
#11004=DIRECTION ( 'NONE',  ( -1.000000000000000000, 0.000000000000000000, 0.000000000000000000 ) ) ;
#11008=CARTESIAN_POINT ( 'NONE',  ( 0.09842519684998451979, 0.1968503937008052596, -3.259751644589256703 ) ) ;
#11012=CARTESIAN_POINT ( 'NONE',  ( 0.3429876364231437824, -0.09193127540148529619, 1.953740157480314821 ) ) ;
#11014=CARTESIAN_POINT ( 'NONE',  ( -0.3010840436257778974, 0.2313841235333766178, -3.100567304031763172 ) ) ;
#11021=CARTESIAN_POINT ( 'NONE',  ( 0.1429116519061375268, 0.5335524835332416949, 0.9399606299212598381 ) ) ;
#11022=DIRECTION ( 'NONE',  ( 0.000000000000000000, 0.000000000000000000, 1.000000000000000000 ) ) ;
#11031=CARTESIAN_POINT ( 'NONE',  ( -0.07874015748031495954, 0.1968503937007873850, -3.548228346456693050 ) ) ;
#11033=FACE_OUTER_BOUND ( 'NONE', #20009, .T. ) ;
#11038=CARTESIAN_POINT ( 'NONE',  ( -0.1480156394741914683, 0.5526079293737398146, 0.9399606299212598381 ) ) ;
#11065=CARTESIAN_POINT ( 'NONE',  ( -0.3252100150720461658, 0.3707612262532960501, -1.550196850393700920 ) ) ;
#11068=CARTESIAN_POINT ( 'NONE',  ( 0.3030032861724964444, -0.3454440660767522098, -1.928289503579156516 ) ) ;
#11069=ADVANCED_FACE ( 'NONE', ( #1453 ), #24611, .T. ) ;
#11092=CARTESIAN_POINT ( 'NONE',  ( 0.3534635626042424428, -0.2712695779737102075, -1.934055118110236338 ) ) ;
#11093=CARTESIAN_POINT ( 'NONE',  ( -0.2807137536170428715, 0.2462256503456040635, -3.115157480314960647 ) ) ;
#11098=CARTESIAN_POINT ( 'NONE',  ( 0.06441914069860960046, -0.4921259842519685179, -1.569881889763779625 ) ) ;
#11111=CARTESIAN_POINT ( 'NONE',  ( -0.2962590301041579388, -0.2272836761397900585, -3.115157480314960647 ) ) ;
#11116=CARTESIAN_POINT ( 'NONE',  ( 0.02190250779246040100, 0.3346456692913385988, 1.953740157480315043 ) ) ;
#11122=ORIENTED_EDGE ( 'NONE', *, *, #14281, .F. ) ;
#11126=CARTESIAN_POINT ( 'NONE',  ( -0.06046497745473627949, 0.3092442853777944700, -3.626959870088829252 ) ) ;
#11145=EDGE_LOOP ( 'NONE', ( #5308, #25346, #20750, #22071 ) ) ;
#11146=DIRECTION ( 'NONE',  ( -0.000000000000000000, -1.000000000000000000, -0.000000000000000000 ) ) ;
#11152=CARTESIAN_POINT ( 'NONE',  ( -0.4382482975805320757, -0.3362148458988418187, 0.9202755905511811330 ) ) ;
#11155=B_SPLINE_CURVE_WITH_KNOTS ( 'NONE', 3,
 ( #3865, #5569, #12480, #14196 ),
 .UNSPECIFIED., .F., .F.,
 ( 4, 4 ),
 ( 0.000000000000000000, 1.000000000000000000 ),
 .UNSPECIFIED. ) ;
#11162=CARTESIAN_POINT ( 'NONE',  ( -0.06048688226688715697, 0.2165354330708661457, -3.626935712454874228 ) ) ;
#11170=CARTESIAN_POINT ( 'NONE',  ( -0.4539000224940974992, -0.3482225189666513510, 0.9399606299212598381 ) ) ;
#11220=EDGE_CURVE ( 'NONE', #25275, #10141, #9323, .T. ) ;
#11223=CARTESIAN_POINT ( 'NONE',  ( 0.09762295995069811272, -0.3644697409450263215, -3.100567304031765836 ) ) ;
#11229=ORIENTED_EDGE ( 'NONE', *, *, #17978, .T. ) ;
#11233=B_SPLINE_CURVE_WITH_KNOTS ( 'NONE', 3,
 ( #14989, #10863, #12433, #19625, #21599, #8462, #19471, #22834, #14466, #5701, #21079, #11906, #10341, #20524, #3267, #9784, #18376, #27029, #3698, #12177, #25318, #7675, #27590, #27171, #1317, #16557, #1586, #5980, #23217, #16290, #3849, #8234, #10057, #3404 ),
 .UNSPECIFIED., .F., .F.,
 ( 4, 2, 2, 2, 2, 2, 2, 2, 2, 2, 2, 2, 2, 2, 2, 2, 4 ),
 ( 0.5000000000000000000, 0.5312500000000000000, 0.5625000000000000000, 0.5937500000000000000, 0.6250000000000001110, 0.6562500000000001110, 0.6875000000000001110, 0.7187500000000001110, 0.7500000000000000000, 0.7812500000000000000, 0.8125000000000001110, 0.8437500000000001110, 0.8750000000000001110, 0.9062500000000002220, 0.9375000000000001110, 0.9687500000000001110, 1.000000000000000000 ),
 .UNSPECIFIED. ) ;
#11235=CARTESIAN_POINT ( 'NONE',  ( -0.3145317858139328182, 0.4092783051644229841, 1.766732283464566899 ) ) ;
#11236=CARTESIAN_POINT ( 'NONE',  ( 0.1649135259617042493, -0.4856708409200646281, 1.766732283464566899 ) ) ;
#11241=VECTOR ( 'NONE', #26043, 39.37007874015748143 ) ;
#11243=CARTESIAN_POINT ( 'NONE',  ( -0.3644697409450256553, 0.09762295995070000010, -3.100567304031767168 ) ) ;
#11249=APPLICATION_CONTEXT ( 'automotive_design' ) ;
#11252=CARTESIAN_POINT ( 'NONE',  ( -0.2521176338356522217, -0.2211428102655704220, 1.953740157480315043 ) ) ;
#11258=CARTESIAN_POINT ( 'NONE',  ( -0.1327952259510255528, -0.4954219348936245160, -1.550196850393701364 ) ) ;
#11262=CARTESIAN_POINT ( 'NONE',  ( 0.07874015748031495954, 0.1968503937007874127, -3.548228346456692162 ) ) ;
#11273=CARTESIAN_POINT ( 'NONE',  ( 0.1570220809524492389, -0.3184841198566451537, 1.953740157480315043 ) ) ;
#11279=DIRECTION ( 'NONE',  ( -1.000000000000000000, 0.000000000000000000, 0.000000000000000000 ) ) ;
#11282=DIRECTION ( 'NONE',  ( -0.000000000000000000, -0.000000000000000000, 1.000000000000000000 ) ) ;
#11290=CARTESIAN_POINT ( 'NONE',  ( -0.3346456692913385988, 2.134256245050205639E-17, 1.973425196850393970 ) ) ;
#11292=CARTESIAN_POINT ( 'NONE',  ( 0.03607471876262466348, 0.5511811023622048555, 0.9399606299212598381 ) ) ;
#11300=CARTESIAN_POINT ( 'NONE',  ( 0.07874015748031495954, 0.1968503937007874127, -3.548228346456692162 ) ) ;
#11307=CARTESIAN_POINT ( 'NONE',  ( -0.5417097841048799101, -0.1839420097223198047, 0.9399606299212598381 ) ) ;
#11314=CARTESIAN_POINT ( 'NONE',  ( -0.03349795313024241800, -0.5118110236220473341, -1.550196850393700920 ) ) ;
#11318=CARTESIAN_POINT ( 'NONE',  ( -0.4857079805365445146, 0.1648275707510890309, -1.550196850393700254 ) ) ;
#11333=DIRECTION ( 'NONE',  ( -0.000000000000000000, -0.000000000000000000, 1.000000000000000000 ) ) ;
#11335=CARTESIAN_POINT ( 'NONE',  ( 0.3001918266902036669, -0.3912931228432058872, -1.550196850393700920 ) ) ;
#11336=CARTESIAN_POINT ( 'NONE',  ( -0.1477428134820414352, -0.4351030398461918081, -1.928289503579139641 ) ) ;
#11338=CARTESIAN_POINT ( 'NONE',  ( 0.03607471876262465654, 0.5511811023622047445, 0.9202755905511811330 ) ) ;
#11341=CARTESIAN_POINT ( 'NONE',  ( 0.2297883689023126064, 0.3979194638820598984, -1.928289503579157183 ) ) ;
#11364=CARTESIAN_POINT ( 'NONE',  ( 0.4219236230596370985, -0.1431838228103867738, -1.934055118110236116 ) ) ;
#11365=CARTESIAN_POINT ( 'NONE',  ( 0.3267488823401750175, 0.1886891683788910201, -3.100567304031762284 ) ) ;
#11369=CARTESIAN_POINT ( 'NONE',  ( -0.3935368318888681771, -0.3024344094364740387, -1.569881889763780070 ) ) ;
#11377=CARTESIAN_POINT ( 'NONE',  ( -0.1649135259616916205, -0.4856708409200665155, 1.747047244094488194 ) ) ;
#11382=CARTESIAN_POINT ( 'NONE',  ( 0.2807137536170455361, -0.2462256503455606815, -3.115157480314960647 ) ) ;
#11383=EDGE_CURVE ( 'NONE', #17093, #5287, #13393, .T. ) ;
#11387=CARTESIAN_POINT ( 'NONE',  ( -0.3346456692913385988, 0.02190250779246044610, 1.953740157480315043 ) ) ;
#11395=CARTESIAN_POINT ( 'NONE',  ( 0.03962771305384435450, 0.1968503937007874127, -3.617038702773737402 ) ) ;
#11397=CARTESIAN_POINT ( 'NONE',  ( 0.06294778803456628491, 0.1968503937007874127, -3.224226213012447051 ) ) ;
#11399=AXIS2_PLACEMENT_3D ( 'NONE', #16563, #27312, #5270 ) ;
#11402=CARTESIAN_POINT ( 'NONE',  ( 0.09842519685039370636, 0.2165354330708661457, -3.272637795275590733 ) ) ;
#11412=CARTESIAN_POINT ( 'NONE',  ( 0.5118110236220472231, 0.03349795313260757468, 1.766732283464566899 ) ) ;
#11423=CARTESIAN_POINT ( 'NONE',  ( -0.2442565704126459791, -0.4954197419817803483, 0.9399606299212598381 ) ) ;
#11433=CARTESIAN_POINT ( 'NONE',  ( -1.452994488188976472E-16, 0.5905905511811023745, -3.548228346456693050 ) ) ;
#11435=CARTESIAN_POINT ( 'NONE',  ( -0.3007905576423960392, -0.1482986320106512990, 1.953740157480315043 ) ) ;
#11440=EDGE_CURVE ( 'NONE', #10350, #19648, #950, .T. ) ;
#11443=CARTESIAN_POINT ( 'NONE',  ( -0.5118110236220472231, -0.06699590632655398614, 1.766732283464566677 ) ) ;
#11444=CARTESIAN_POINT ( 'NONE',  ( -0.09842519685039370636, 0.2165354330708661457, -3.548228346456693050 ) ) ;
#11457=ORIENTED_EDGE ( 'NONE', *, *, #22449, .F. ) ;
#11463=B_SPLINE_CURVE_WITH_KNOTS ( 'NONE', 3,
 ( #538, #3184, #26642, #1097, #13380, #7297, #22418, #20016, #7164, #22005, #16064, #18143, #15916, #11397, #2638, #13799, #26787, #24656 ),
 .UNSPECIFIED., .F., .F.,
 ( 4, 2, 2, 2, 2, 2, 2, 2, 4 ),
 ( 0.000000000000000000, 0.1250000000000000000, 0.2500000000000000000, 0.3750000000000000000, 0.5000000000000000000, 0.6250000000000000000, 0.7500000000000000000, 0.8750000000000000000, 1.000000000000000000 ),
 .UNSPECIFIED. ) ;
#11470=CARTESIAN_POINT ( 'NONE',  ( 0.09842519685039360922, 0.2991866959364321565, -3.554782022675774922 ) ) ;
#11471=CARTESIAN_POINT ( 'NONE',  ( -0.5118110236220473341, 0.000000000000000000, -1.550196850393700920 ) ) ;
#11472=CARTESIAN_POINT ( 'NONE',  ( -0.2796934465393772773, -0.3645739570812616681, -1.928289503579163178 ) ) ;
#11479=AXIS2_PLACEMENT_3D ( 'NONE', #13389, #19756, #9412 ) ;
#11480=CARTESIAN_POINT ( 'NONE',  ( -0.3707612262532960501, 0.3252100150720461658, -1.569881889763779625 ) ) ;
#11494=CARTESIAN_POINT ( 'NONE',  ( 0.4527559054764770385, 0.02963280468032115228, -1.934055118110236338 ) ) ;
#11505=CARTESIAN_POINT ( 'NONE',  ( -0.02464264302293858039, -0.3765118517642103702, -3.100567304031763172 ) ) ;
#11516=CARTESIAN_POINT ( 'NONE',  ( 0.5118110236220472231, -0.03349795313260760937, 1.766732283464566899 ) ) ;
#11519=CARTESIAN_POINT ( 'NONE',  ( -0.2807137536170348779, -0.2462256503456018430, -3.115157480314960647 ) ) ;
#11537=FACE_OUTER_BOUND ( 'NONE', #26626, .T. ) ;
#11542=CARTESIAN_POINT ( 'NONE',  ( -0.2676050456844304426, -0.2056553984168022764, 1.973425196850394414 ) ) ;
#11545=DIRECTION ( 'NONE',  ( 0.000000000000000000, 0.000000000000000000, 1.000000000000000000 ) ) ;
#11548=CARTESIAN_POINT ( 'NONE',  ( -0.5280699926563169333, 0.06957181182499308503, 1.747047244094488194 ) ) ;
#11558=CARTESIAN_POINT ( 'NONE',  ( -0.3912931228432153796, -0.3001918266902245391, -1.569881889763779625 ) ) ;
#11561=CARTESIAN_POINT ( 'NONE',  ( 0.3642352168757231889, -0.4152525734085952269, 0.9399606299212598381 ) ) ;
#11576=EDGE_CURVE ( 'NONE', #19099, #26373, #5656, .T. ) ;
#11577=CARTESIAN_POINT ( 'NONE',  ( -0.2521176338356522217, -0.2211428102655704220, 1.953740157480315043 ) ) ;
#11588=AXIS2_PLACEMENT_3D ( 'NONE', #5229, #3665, #7923 ) ;
#11606=CARTESIAN_POINT ( 'NONE',  ( -0.2904160862623674788, 0.1677079028045369846, 1.973425196850393970 ) ) ;
#11607=CARTESIAN_POINT ( 'NONE',  ( 0.2466292688015316592, -0.4270824798167792147, -1.550196850393700920 ) ) ;
#11617=LINE ( 'NONE', #756, #24875 ) ;
#11624=CARTESIAN_POINT ( 'NONE',  ( 0.2816963220975960414, 0.2161875334158293027, 1.953740157480315043 ) ) ;
#11627=CARTESIAN_POINT ( 'NONE',  ( -0.2991932138496239402, -0.3411003281196705594, -1.934055118110236338 ) ) ;
#11631=DIRECTION ( 'NONE',  ( 0.000000000000000000, 0.000000000000000000, -1.000000000000000000 ) ) ;
#11633=DIRECTION ( 'NONE',  ( -1.000000000000000000, 0.000000000000000000, 0.000000000000000000 ) ) ;
#11639=CARTESIAN_POINT ( 'NONE',  ( -0.3765118517642104257, 0.02464264302297881210, -3.100567304031763172 ) ) ;
#11644=CARTESIAN_POINT ( 'NONE',  ( -0.1432577568504646015, 0.4218945342797250642, -1.934055118110236338 ) ) ;
#11654=CARTESIAN_POINT ( 'NONE',  ( 0.1327036767659691974, 0.4954415918531168139, 1.747047244094488194 ) ) ;
#11657=CARTESIAN_POINT ( 'NONE',  ( 0.3726024258163779246, -0.02438677169350792623, -3.115157480314960647 ) ) ;
#11662=ORIENTED_EDGE ( 'NONE', *, *, #13330, .F. ) ;
#11670=ADVANCED_FACE ( 'NONE', ( #17616 ), #5597, .F. ) ;
#11674=CARTESIAN_POINT ( 'NONE',  ( 0.09842519685039360922, 0.1968503937007873850, -3.272637795275590733 ) ) ;
#11678=DIRECTION ( 'NONE',  ( 0.000000000000000000, 0.000000000000000000, -1.000000000000000000 ) ) ;
#11681=CARTESIAN_POINT ( 'NONE',  ( -0.2817310484609166221, 0.2161381151963042424, 1.953740157480315043 ) ) ;
#11688=CARTESIAN_POINT ( 'NONE',  ( -0.4612490782034870396, -0.2663596103035605345, 1.747047244094488194 ) ) ;
#11689=CARTESIAN_POINT ( 'NONE',  ( -0.1649135259617042215, 0.4856708409200647392, 1.766732283464566899 ) ) ;
#11695=CARTESIAN_POINT ( 'NONE',  ( -0.2341075107471362049, -0.2669897767696617352, 1.953740157480315043 ) ) ;
#11699=CARTESIAN_POINT ( 'NONE',  ( 0.2466292688015208900, -0.4270824798167630054, -1.569881889763779625 ) ) ;
#11702=CARTESIAN_POINT ( 'NONE',  ( -0.03607471876262562799, -0.5511811023622048555, 0.9399606299212598381 ) ) ;
#11707=DIRECTION ( 'NONE',  ( -0.000000000000000000, -1.000000000000000000, -0.000000000000000000 ) ) ;
#11716=CARTESIAN_POINT ( 'NONE',  ( 0.08676778863011140597, -0.3239425792934415571, 1.953740157480315043 ) ) ;
#11736=CARTESIAN_POINT ( 'NONE',  ( -0.01030706208231915028, 0.1968503937007873850, -3.626968503937007871 ) ) ;
#11744=CARTESIAN_POINT ( 'NONE',  ( 0.5511811023622047445, 0.000000000000000000, -1.550196850393700920 ) ) ;
#11748=CARTESIAN_POINT ( 'NONE',  ( 0.4889536969034952718, -0.06441834428466330920, -1.550196850393700920 ) ) ;
#11750=CARTESIAN_POINT ( 'NONE',  ( -0.5230301363771269196, -0.1775991818008745282, 0.9202755905511811330 ) ) ;
#11768=CARTESIAN_POINT ( 'NONE',  ( -0.3543321272855304849, 0.02325127328527686055, 1.953740157480315709 ) ) ;
#11770=EDGE_LOOP ( 'NONE', ( #1007, #27039, #18557, #17960 ) ) ;
#11772=CARTESIAN_POINT ( 'NONE',  ( 0.3929158813954871654, 0.2268989272875732710, -1.934055118110236338 ) ) ;
#11781=CARTESIAN_POINT ( 'NONE',  ( -0.4417544603400644920, -0.05811278586497442555, -1.934055118110237004 ) ) ;
#11786=CARTESIAN_POINT ( 'NONE',  ( -0.1970259548081969847, -0.3996230174612658281, -1.934055118110236338 ) ) ;
#11788=CARTESIAN_POINT ( 'NONE',  ( -0.3979194638820449104, -0.2297883689023288989, -1.928289503579160513 ) ) ;
#11791=EDGE_CURVE ( 'NONE', #25, #5266, #8991, .T. ) ;
#11794=CARTESIAN_POINT ( 'NONE',  ( 0.07874015748031495954, 0.1968503937007873850, -3.364501312335955063 ) ) ;
#11796=CARTESIAN_POINT ( 'NONE',  ( 0.4954415918530851726, -0.1327036767659643957, 1.766732283464566899 ) ) ;
#11799=CARTESIAN_POINT ( 'NONE',  ( 0.2993674444872273521, 0.2296683860596781812, -3.100567304031764060 ) ) ;
#11807=FACE_OUTER_BOUND ( 'NONE', #6003, .T. ) ;
#11810=CARTESIAN_POINT ( 'NONE',  ( -0.1970259548081969847, -0.3996230174612658281, -1.934055118110236338 ) ) ;
#11816=CARTESIAN_POINT ( 'NONE',  ( -0.3102476824511312681, 0.1791601451669032896, -3.115157480314960647 ) ) ;
#11817=DIRECTION ( 'NONE',  ( 0.000000000000000000, 0.000000000000000000, -1.000000000000000000 ) ) ;
#11818=CARTESIAN_POINT ( 'NONE',  ( -0.2056553984168022209, 0.2676050456844303316, 1.973425196850394414 ) ) ;
#11822=CARTESIAN_POINT ( 'NONE',  ( 0.1141709026133613525, -0.3362336590883617249, 1.953740157480315043 ) ) ;
#11823=ORIENTED_EDGE ( 'NONE', *, *, #6894, .F. ) ;
#11829=CARTESIAN_POINT ( 'NONE',  ( -0.4225965726692976765, -0.3242071728275119913, 1.747047244094488194 ) ) ;
#11832=CARTESIAN_POINT ( 'NONE',  ( 0.03349795313264414959, -0.5118110236220471121, 1.766732283464566899 ) ) ;
#11843=CARTESIAN_POINT ( 'NONE',  ( -0.2180862235769562008, -0.4423390553432419714, -1.569881889763779625 ) ) ;
#11856=CARTESIAN_POINT ( 'NONE',  ( -0.3007905576423956506, 0.1482986320106521871, 1.953740157480315043 ) ) ;
#11862=CARTESIAN_POINT ( 'NONE',  ( -0.4984899526255159863, -0.1339654526248284516, 1.766732283464567121 ) ) ;
#11869=CARTESIAN_POINT ( 'NONE',  ( 0.5085287184740714395, 0.06690297524259165851, -1.550196850393700920 ) ) ;
#11874=CARTESIAN_POINT ( 'NONE',  ( -0.3121994997578409481, -0.4069448477569437284, -1.550196850393700920 ) ) ;
#11877=CARTESIAN_POINT ( 'NONE',  ( -0.02061007003135920460, 0.1968503937007873850, -3.624919108234672560 ) ) ;
#11891=CARTESIAN_POINT ( 'NONE',  ( -0.2041304421298332783, 0.2660793235464289364, 1.973425196850393970 ) ) ;
#11892=CARTESIAN_POINT ( 'NONE',  ( -0.1327036767636080028, -0.4954415918535519658, -1.550196850393700920 ) ) ;
#11895=CARTESIAN_POINT ( 'NONE',  ( -0.5511811023622047445, -0.03607471876259067678, 0.9202755905511811330 ) ) ;
#11906=CARTESIAN_POINT ( 'NONE',  ( -0.2662790972932065348, 0.4613045817965927831, 1.747047244094488638 ) ) ;
#11907=DIRECTION ( 'NONE',  ( -1.000000000000000000, 0.000000000000000000, 0.000000000000000000 ) ) ;
#11914=CARTESIAN_POINT ( 'NONE',  ( -0.2161875334158534223, 0.2816963220975619575, 1.953740157480314821 ) ) ;
#11918=CARTESIAN_POINT ( 'NONE',  ( 0.2268989272875507057, -0.3929158813954434226, -1.934055118110236338 ) ) ;
#11925=CARTESIAN_POINT ( 'NONE',  ( -2.685748425196850164E-17, 0.000000000000000000, -1.934055118110236338 ) ) ;
#11929=CARTESIAN_POINT ( 'NONE',  ( -0.3740848232703753440, -0.04928467685643751067, -3.100567304031760507 ) ) ;
#11930=CARTESIAN_POINT ( 'NONE',  ( 0.3213085410496531180, -0.1584824234588266545, -3.115157480314961091 ) ) ;
#11934=CARTESIAN_POINT ( 'NONE',  ( -0.4527559054764770385, 0.000000000000000000, -1.934055118110236338 ) ) ;
#11940=CARTESIAN_POINT ( 'NONE',  ( 0.09842519685039366473, 0.1968503937007873850, -3.364501312335956396 ) ) ;
#11942=CARTESIAN_POINT ( 'NONE',  ( 0.5144970376936013334, 0.1378076643338890239, 1.747047244094488194 ) ) ;
#11947=CARTESIAN_POINT ( 'NONE',  ( 0.02464264302293732445, -0.3765118517642105367, -3.100567304031763172 ) ) ;
#11955=CARTESIAN_POINT ( 'NONE',  ( 0.3996230174612959707, 0.1970259548082022305, -1.934055118110236338 ) ) ;
#11961=CARTESIAN_POINT ( 'NONE',  ( 0.04679574315772144777, 0.3551931031211610912, -3.115157480314960647 ) ) ;
#11966=EDGE_CURVE ( 'NONE', #1047, #7118, #22486, .T. ) ;
#11967=CARTESIAN_POINT ( 'NONE',  ( -0.08600259727896246431, 0.2165354330708661457, -3.223068997994991580 ) ) ;
#11968=CARTESIAN_POINT ( 'NONE',  ( -0.08759279594700329630, -0.3259357382551448246, 1.973425196850394192 ) ) ;
#11977=CARTESIAN_POINT ( 'NONE',  ( 0.2268096725222282783, -0.4600326175560538466, 1.747047244094488194 ) ) ;
#11978=CARTESIAN_POINT ( 'NONE',  ( -0.4600326175560602304, -0.2268096725222347454, 1.766732283464566899 ) ) ;
#11992=CARTESIAN_POINT ( 'NONE',  ( -0.1275996891957758561, 0.4763861460130329184, -1.569881889763779625 ) ) ;
#11994=ORIENTED_EDGE ( 'NONE', *, *, #11440, .F. ) ;
#12004=CARTESIAN_POINT ( 'NONE',  ( -0.2041304421298503480, 0.2660793235464394280, 1.953740157480315043 ) ) ;
#12012=CARTESIAN_POINT ( 'NONE',  ( -0.3024344094364738722, 0.3935368318888683437, -1.569881889763779625 ) ) ;
#12018=CARTESIAN_POINT ( 'NONE',  ( -0.4417502570507843007, 0.05811937031580000773, -1.934055118110236560 ) ) ;
#12021=CARTESIAN_POINT ( 'NONE',  ( -0.5511811023622047445, 6.750021727583836750E-17, -1.550196850393700920 ) ) ;
#12022=CARTESIAN_POINT ( 'NONE',  ( 0.01288382760289894131, 0.1968503937007873850, -3.646653543307086576 ) ) ;
#12035=CARTESIAN_POINT ( 'NONE',  ( -0.4856708409191258236, -0.1649135259639268325, -1.550196850393700920 ) ) ;
#12036=CARTESIAN_POINT ( 'NONE',  ( 0.5511811023622047445, 3.414809992080329023E-17, 0.9202755905511811330 ) ) ;
#12037=CARTESIAN_POINT ( 'NONE',  ( -0.3362148458988263311, -0.4382482975805425118, 0.9202755905511811330 ) ) ;
#12042=CARTESIAN_POINT ( 'NONE',  ( 0.4889536969035315206, 0.06441834428467128892, -1.569881889763779625 ) ) ;
#12046=ORIENTED_EDGE ( 'NONE', *, *, #2179, .F. ) ;
#12053=CARTESIAN_POINT ( 'NONE',  ( -0.3429876364231290164, 0.09193127540154458210, 1.953740157480315043 ) ) ;
#12057=CARTESIAN_POINT ( 'NONE',  ( 0.01308949271087063437, 0.3147523155727945943, -3.174873752692270124 ) ) ;
#12068=CARTESIAN_POINT ( 'NONE',  ( 0.2842163005028049971, -0.2181214148710412248, -3.115157480314961091 ) ) ;
#12070=CARTESIAN_POINT ( 'NONE',  ( 0.4417361510193959506, -0.05819755867303935681, -1.934055118110236338 ) ) ;
#12072=ORIENTED_EDGE ( 'NONE', *, *, #20343, .F. ) ;
#12077=CARTESIAN_POINT ( 'NONE',  ( -0.5280699926563170443, -0.06957181182498474448, 1.747047244094488194 ) ) ;
#12082=CARTESIAN_POINT ( 'NONE',  ( 0.2836590635674658412, -0.2488091035916875082, -3.100567304031767168 ) ) ;
#12089=CARTESIAN_POINT ( 'NONE',  ( -0.02909913904662018644, 0.4446020952038907681, -1.934055118110236338 ) ) ;
#12096=CARTESIAN_POINT ( 'NONE',  ( -0.04679574315772456333, -0.3551931031211519874, -3.115157480314960647 ) ) ;
#12097=CARTESIAN_POINT ( 'NONE',  ( 0.07214943758244279914, -0.5511811023622047445, 0.9202755905511812440 ) ) ;
#12102=CARTESIAN_POINT ( 'NONE',  ( 0.3259357382551448246, -0.08759279594700333793, 1.973425196850394192 ) ) ;
#12105=CARTESIAN_POINT ( 'NONE',  ( 0.5708661417322835607, 6.829619984160658046E-17, 0.9399606299212598381 ) ) ;
#12106=CARTESIAN_POINT ( 'NONE',  ( 0.000000000000000000, 0.000000000000000000, 2.504921259842519898 ) ) ;
#12110=CARTESIAN_POINT ( 'NONE',  ( 0.3382184156731939395, -0.3855916753051315538, 1.747047244094488194 ) ) ;
#12112=CARTESIAN_POINT ( 'NONE',  ( 0.4954415918531143714, 0.1327036767659736105, 1.747047244094488194 ) ) ;
#12122=ADVANCED_FACE ( 'NONE', ( #7313 ), #10717, .T. ) ;
#12125=CARTESIAN_POINT ( 'NONE',  ( -0.3707612262533165337, -0.3252100150720257932, -1.569881889763779625 ) ) ;
#12128=CARTESIAN_POINT ( 'NONE',  ( -0.3574975638436101444, 0.000000000000000000, -3.115157480314960647 ) ) ;
#12140=CARTESIAN_POINT ( 'NONE',  ( 0.5708661417322835607, 6.829619984160658046E-17, 0.9399606299212598381 ) ) ;
#12146=EDGE_CURVE ( 'NONE', #5072, #21621, #12382, .T. ) ;
#12153=CARTESIAN_POINT ( 'NONE',  ( 0.4954247181591565075, 0.1327957795770679794, -1.550196850393700476 ) ) ;
#12158=CARTESIAN_POINT ( 'NONE',  ( -0.4857053587577855880, -0.1648264847746778727, -1.550196850393700920 ) ) ;
#12168=CARTESIAN_POINT ( 'NONE',  ( -0.5335524835332036142, 0.1429116519061177371, 0.9399606299212598381 ) ) ;
#12177=CARTESIAN_POINT ( 'NONE',  ( 0.1379038425970668946, 0.5144793533648593931, 1.747047244094488194 ) ) ;
#12202=CARTESIAN_POINT ( 'NONE',  ( -0.3574975638436101444, -0.02348089843015294109, -3.115157480314960203 ) ) ;
#12204=CARTESIAN_POINT ( 'NONE',  ( 0.4270824798167637826, -0.2466292688015195855, -1.569881889763779625 ) ) ;
#12207=CARTESIAN_POINT ( 'NONE',  ( -0.05819755867304135522, -0.4417361510194244278, -1.934055118110236338 ) ) ;
#12217=CARTESIAN_POINT ( 'NONE',  ( -0.3512268162760389667, -0.4004221243553605092, 1.747047244094488194 ) ) ;
#12222=CARTESIAN_POINT ( 'NONE',  ( 0.02464264302293787262, 0.3765118517642104257, -3.100567304031763172 ) ) ;
#12224=CARTESIAN_POINT ( 'NONE',  ( -0.4921259842519685179, 6.026805113914139867E-17, -1.934055118110236338 ) ) ;
#12225=CARTESIAN_POINT ( 'NONE',  ( -0.09187177619658884464, -0.3429980251342297226, 1.953740157480315043 ) ) ;
#12229=CARTESIAN_POINT ( 'NONE',  ( 0.5230301363770953893, -0.1775991818008574585, 0.9399606299212598381 ) ) ;
#12237=CARTESIAN_POINT ( 'NONE',  ( 0.2693339498142349187, -0.2362439534887297299, -3.115157480314960647 ) ) ;
#12238=CARTESIAN_POINT ( 'NONE',  ( -0.4407612517155323206, -0.3387265385688508768, 0.9202755905511813550 ) ) ;
#12244=EDGE_CURVE ( 'NONE', #20990, #21275, #23863, .T. ) ;
#12250=CARTESIAN_POINT ( 'NONE',  ( 0.4612490782034816550, -0.2663596103035388296, 1.747047244094488194 ) ) ;
#12251=CARTESIAN_POINT ( 'NONE',  ( 0.5118110236220472231, -0.03349795313260760937, 1.766732283464566899 ) ) ;
#12260=FACE_OUTER_BOUND ( 'NONE', #25067, .T. ) ;
#12265=CARTESIAN_POINT ( 'NONE',  ( 0.4889536969034952718, -0.06441834428466330920, -1.550196850393700920 ) ) ;
#12278=EDGE_CURVE ( 'NONE', #22294, #16690, #4597, .T. ) ;
#12295=FACE_OUTER_BOUND ( 'NONE', #7293, .T. ) ;
#12308=CARTESIAN_POINT ( 'NONE',  ( 0.2660793235464212203, 0.2041304421298323901, 1.953740157480315043 ) ) ;
#12315=CARTESIAN_POINT ( 'NONE',  ( 0.1429116519061152946, -0.5335524835331961757, 0.9399606299212598381 ) ) ;
#12326=CARTESIAN_POINT ( 'NONE',  ( -0.2712027394948519632, -0.3535065162672669792, -1.934055118110236338 ) ) ;
#12327=CARTESIAN_POINT ( 'NONE',  ( -0.5905511811023621549, 7.232166136696967594E-17, 0.9399606299212598381 ) ) ;
#12328=CARTESIAN_POINT ( 'NONE',  ( -0.06690297524288160713, 0.5085287184739378796, -1.550196850393700476 ) ) ;
#12350=CARTESIAN_POINT ( 'NONE',  ( 0.1970259548082107792, -0.3996230174612653285, -1.934055118110236338 ) ) ;
#12357=CARTESIAN_POINT ( 'NONE',  ( 0.3382184156731939395, -0.3855916753051315538, 1.747047244094488194 ) ) ;
#12361=CARTESIAN_POINT ( 'NONE',  ( -0.1668516812751421607, 0.3384212623783116602, -3.100567304031759175 ) ) ;
#12362=AXIS2_PLACEMENT_3D ( 'NONE', #20394, #26743, #11631 ) ;
#12365=CARTESIAN_POINT ( 'NONE',  ( 0.1570220809524492389, -0.3184841198566451537, 1.953740157480315043 ) ) ;
#12369=CARTESIAN_POINT ( 'NONE',  ( -0.2313841235333770063, -0.3010840436257778419, -3.100567304031762284 ) ) ;
#12370=CARTESIAN_POINT ( 'NONE',  ( 0.4539000224941339701, 0.3482225189666781073, 0.9399606299212598381 ) ) ;
#12378=CARTESIAN_POINT ( 'NONE',  ( -0.3574975638436101444, 0.000000000000000000, -3.115157480314960647 ) ) ;
#12382=B_SPLINE_CURVE_WITH_KNOTS ( 'NONE', 3,
 ( #27377, #19024, #25535, #7885, #16634, #23142, #8308, #16490, #25249, #21297 ),
 .UNSPECIFIED., .F., .F.,
 ( 4, 2, 2, 2, 4 ),
 ( 0.5000000000000000000, 0.6250000000000000000, 0.7500000000000000000, 0.8750000000000000000, 1.000000000000000000 ),
 .UNSPECIFIED. ) ;
#12397=CARTESIAN_POINT ( 'NONE',  ( 0.4600326175560603970, 0.2268096725222477072, 1.747047244094488194 ) ) ;
#12402=ORIENTED_EDGE ( 'NONE', *, *, #16442, .F. ) ;
#12407=CARTESIAN_POINT ( 'NONE',  ( 0.2521176338356569957, 0.2211428102655756955, 1.973425196850393970 ) ) ;
#12411=CARTESIAN_POINT ( 'NONE',  ( -0.4921259842519395411, 0.03220957031763951872, -1.550196850393700920 ) ) ;
#12425=ORIENTED_EDGE ( 'NONE', *, *, #24266, .T. ) ;
#12433=CARTESIAN_POINT ( 'NONE',  ( -0.5280876769851563513, 0.06947563356136872426, 1.747047244094487972 ) ) ;
#12437=CARTESIAN_POINT ( 'NONE',  ( 0.4068940122748140875, 0.3122781343794410747, -1.550196850393701142 ) ) ;
#12444=LINE ( 'NONE', #12021, #10759 ) ;
#12445=CARTESIAN_POINT ( 'NONE',  ( 0.07214854559196579031, 0.5476281405333208729, 0.9202755905511811330 ) ) ;
#12455=CARTESIAN_POINT ( 'NONE',  ( -0.08600259748438122964, 0.2165354330708661457, -3.597797143241368456 ) ) ;
#12458=CARTESIAN_POINT ( 'NONE',  ( -0.04380447413658832695, 0.3324885138898346360, 1.953740157480315043 ) ) ;
#12459=CARTESIAN_POINT ( 'NONE',  ( -0.5118110236220473341, 0.000000000000000000, -1.550196850393700920 ) ) ;
#12465=CARTESIAN_POINT ( 'NONE',  ( -0.3460530745557111598, 0.09275304139139804727, -3.115157480314960203 ) ) ;
#12470=CARTESIAN_POINT ( 'NONE',  ( -0.5118110236220182463, 0.03349795313034509281, -1.550196850393700920 ) ) ;
#12480=CARTESIAN_POINT ( 'NONE',  ( 0.07874015748031495954, 0.1968503937007874127, -3.456364829396325167 ) ) ;
#12491=CARTESIAN_POINT ( 'NONE',  ( 0.2466292688015208900, -0.4270824798167630054, -1.569881889763779625 ) ) ;
#12495=CARTESIAN_POINT ( 'NONE',  ( 0.4527559054764770385, -0.02963280468032104126, -1.934055118110236338 ) ) ;
#12496=CARTESIAN_POINT ( 'NONE',  ( 0.3979194638820598984, -0.2297883689023126064, -1.928289503579157183 ) ) ;
#12502=CARTESIAN_POINT ( 'NONE',  ( 0.4441657790107724213, -0.2564944395515492137, 1.747047244094488194 ) ) ;
#12506=CARTESIAN_POINT ( 'NONE',  ( -0.09842519685039370636, 0.2165354330708661457, -3.364501312335958172 ) ) ;
#12511=CARTESIAN_POINT ( 'NONE',  ( 0.1141709026133643362, 0.3362336590883639453, 1.953740157480315043 ) ) ;
#12515=CARTESIAN_POINT ( 'NONE',  ( -0.5708661417322835607, -0.03736310157554036115, 0.9399606299212598381 ) ) ;
#12520=CARTESIAN_POINT ( 'NONE',  ( 0.02339816079119088829, 0.3574975638436101444, -3.115157480314960647 ) ) ;
#12525=EDGE_CURVE ( 'NONE', #17898, #7118, #23153, .T. ) ;
#12538=CARTESIAN_POINT ( 'NONE',  ( 0.5043504886477717664, -0.1712563538833085097, 1.747047244094488194 ) ) ;
#12543=CARTESIAN_POINT ( 'NONE',  ( 0.3551931031211519874, -0.04679574315772458415, -3.115157480314960647 ) ) ;
#12545=CARTESIAN_POINT ( 'NONE',  ( -0.4585215200179055817, 2.807634559150536355E-17, -1.928289503579156516 ) ) ;
#12549=CARTESIAN_POINT ( 'NONE',  ( -0.04380447413658627998, 0.3324885138898243664, 1.973425196850393970 ) ) ;
#12550=ORIENTED_EDGE ( 'NONE', *, *, #556, .T. ) ;
#12552=CARTESIAN_POINT ( 'NONE',  ( 0.03220957031753989008, 0.4921259842519685179, -1.550196850393700920 ) ) ;
#12555=AXIS2_PLACEMENT_3D ( 'NONE', #11925, #9365, #20116 ) ;
#12583=CARTESIAN_POINT ( 'NONE',  ( -0.1429116519061127688, 0.5335524835332354776, 0.9202755905511811330 ) ) ;
#12585=CARTESIAN_POINT ( 'NONE',  ( 0.000000000000000000, 0.000000000000000000, 2.504921259842519898 ) ) ;
#12586=ORIENTED_EDGE ( 'NONE', *, *, #6335, .F. ) ;
#12593=PLANE ( 'NONE',  #27676 ) ;
#12598=CARTESIAN_POINT ( 'NONE',  ( -0.08676778863011123943, 0.3239425792934299553, 1.953740157480315043 ) ) ;
#12602=CARTESIAN_POINT ( 'NONE',  ( 0.03607471876262466348, 0.5511811023622048555, 0.9399606299212598381 ) ) ;
#12606=CARTESIAN_POINT ( 'NONE',  ( 0.2361997806693254542, 0.2693761163850786344, -3.115157480314960647 ) ) ;
#12613=ORIENTED_EDGE ( 'NONE', *, *, #12244, .F. ) ;
#12614=CARTESIAN_POINT ( 'NONE',  ( -0.03746919241598681977, -0.5708647227724242823, 0.9399606299212600602 ) ) ;
#12617=CARTESIAN_POINT ( 'NONE',  ( -0.3242892624568586291, -0.4225434286519560989, 1.747047244094488194 ) ) ;
#12618=CARTESIAN_POINT ( 'NONE',  ( 0.1327952259511945843, 0.4954219348936774736, -1.550196850393700476 ) ) ;
#12631=CARTESIAN_POINT ( 'NONE',  ( 0.2761764805255614297, 0.3599896729929412120, -1.934055118110236338 ) ) ;
#12646=CARTESIAN_POINT ( 'NONE',  ( 0.04638120790932724613, 0.3520466617656882735, 1.953740157480315043 ) ) ;
#12655=CARTESIAN_POINT ( 'NONE',  ( 0.2272836761397900307, -0.2962590301041579388, -3.115157480314960647 ) ) ;
#12660=CARTESIAN_POINT ( 'NONE',  ( 0.4921259842519685179, 2.987958743070287587E-17, -1.569881889763779625 ) ) ;
#12664=VERTEX_POINT ( 'NONE', #21399 ) ;
#12665=CARTESIAN_POINT ( 'NONE',  ( -0.1838434515542552161, 0.5417490723636845251, 0.9399606299212600602 ) ) ;
#12676=CARTESIAN_POINT ( 'NONE',  ( -0.1791601451668923262, -0.3102476824511486986, -3.115157480314960647 ) ) ;
#12677=CARTESIAN_POINT ( 'NONE',  ( -0.3666644560843326794, -0.2817828961649162522, -1.928289503579156516 ) ) ;
#12679=CARTESIAN_POINT ( 'NONE',  ( -0.1677079028045458664, 0.2904160862623615391, 1.973425196850393970 ) ) ;
#12690=CARTESIAN_POINT ( 'NONE',  ( -0.07874642858611770324, 0.3051016904613214620, -3.608673911198624129 ) ) ;
#12701=CARTESIAN_POINT ( 'NONE',  ( -0.4585215200179055817, 2.807634559150536355E-17, -1.928289503579156516 ) ) ;
#12705=CARTESIAN_POINT ( 'NONE',  ( -0.02061007003135897908, 0.1968503937007873850, -3.195947033497543721 ) ) ;
#12711=MANIFOLD_SOLID_BREP ( 'Cam Shaft', #2849 ) ;
#12726=ORIENTED_EDGE ( 'NONE', *, *, #12146, .F. ) ;
#12734=CARTESIAN_POINT ( 'NONE',  ( 0.5476281405333119912, 0.07214854559198101425, 0.9399606299212598381 ) ) ;
#12738=CARTESIAN_POINT ( 'NONE',  ( -0.2693761163850975637, 0.2361997806693252044, -3.115157480314961091 ) ) ;
#12743=CARTESIAN_POINT ( 'NONE',  ( -0.1327036767636164405, 0.4954415918535620134, -1.550196850393700920 ) ) ;
#12745=CARTESIAN_POINT ( 'NONE',  ( -0.5417490723642327533, -0.1838434515534312919, 0.9399606299212597271 ) ) ;
#12746=LINE ( 'NONE', #17545, #23758 ) ;
#12749=EDGE_CURVE ( 'NONE', #5588, #20420, #11617, .T. ) ;
#12750=CARTESIAN_POINT ( 'NONE',  ( 0.2268956277329844951, 0.4599954779395432625, -1.550196850393701364 ) ) ;
#12753=ORIENTED_EDGE ( 'NONE', *, *, #18277, .T. ) ;
#12766=EDGE_CURVE ( 'NONE', #10805, #1064, #4981, .T. ) ;
#12768=CARTESIAN_POINT ( 'NONE',  ( 0.3599896729929407679, 0.2761764805255620403, -1.934055118110236338 ) ) ;
#12774=CARTESIAN_POINT ( 'NONE',  ( 0.4612490782034816550, -0.2663596103035388296, 1.747047244094488194 ) ) ;
#12780=CARTESIAN_POINT ( 'NONE',  ( -0.3534635626044764778, 0.2712695779735687651, -1.934055118110236116 ) ) ;
#12782=CARTESIAN_POINT ( 'NONE',  ( -0.1570220809524502104, -0.3184841198566448206, 1.953740157480315043 ) ) ;
#12790=CARTESIAN_POINT ( 'NONE',  ( 0.2529800193559499921, -0.5131133041954075713, 0.9399606299212598381 ) ) ;
#12796=CARTESIAN_POINT ( 'NONE',  ( 0.3702005978258383068, -0.04877294052296102245, -3.115157480314960647 ) ) ;
#12805=CARTESIAN_POINT ( 'NONE',  ( 0.4921259842519685179, 5.975917486140575174E-17, -1.550196850393700920 ) ) ;
#12808=CARTESIAN_POINT ( 'NONE',  ( -0.3855916753051542023, -0.3382184156732014890, 1.766732283464566899 ) ) ;
#12809=CARTESIAN_POINT ( 'NONE',  ( -0.5118110236220472231, -0.03349795313264326835, 1.747047244094488194 ) ) ;
#12810=VERTEX_POINT ( 'NONE', #4102 ) ;
#12813=CARTESIAN_POINT ( 'NONE',  ( 0.2842490391651533721, -0.2180698645301867300, -3.115157480314960647 ) ) ;
#12814=ORIENTED_EDGE ( 'NONE', *, *, #7789, .T. ) ;
#12815=CARTESIAN_POINT ( 'NONE',  ( 0.4585215200179055817, -2.840735999735804609E-17, -1.928289503579156516 ) ) ;
#12819=CARTESIAN_POINT ( 'NONE',  ( -0.2904160862623646477, -0.1677079028045411757, 1.973425196850393970 ) ) ;
#12823=CARTESIAN_POINT ( 'NONE',  ( 0.1275996891957731083, 0.4763861460130595082, -1.550196850393700920 ) ) ;
#12840=CARTESIAN_POINT ( 'NONE',  ( 0.1288129352161813124, 0.4793172621399190980, -1.569881889763779625 ) ) ;
#12843=CARTESIAN_POINT ( 'NONE',  ( 0.04838950581351087604, 0.1968503937007873850, -3.209671902477004402 ) ) ;
#12850=EDGE_CURVE ( 'NONE', #12810, #88, #21045, .T. ) ;
#12866=ORIENTED_EDGE ( 'NONE', *, *, #18277, .F. ) ;
#12874=CARTESIAN_POINT ( 'NONE',  ( -0.3642352168757849173, -0.4152525734086955356, 0.9399606299212598381 ) ) ;
#12876=CARTESIAN_POINT ( 'NONE',  ( -0.3574975638436101444, 0.000000000000000000, -3.115157480314960647 ) ) ;
#12881=CARTESIAN_POINT ( 'NONE',  ( -0.3855916753034290823, 0.3382184156749268311, -1.550196850393700920 ) ) ;
#12888=EDGE_CURVE ( 'NONE', #5007, #19599, #5551, .T. ) ;
#12903=CARTESIAN_POINT ( 'NONE',  ( -0.4527559054764770385, 0.000000000000000000, -1.934055118110236338 ) ) ;
#12905=CARTESIAN_POINT ( 'NONE',  ( 0.2268967137093004516, -0.4599980997183342746, -1.550196850393700920 ) ) ;
#12917=CARTESIAN_POINT ( 'NONE',  ( -0.2937497900409605234, 0.3350145293473837382, -1.934055118110236338 ) ) ;
#12922=CARTESIAN_POINT ( 'NONE',  ( -0.5417097841048799101, -0.1839420097223198047, 0.9399606299212598381 ) ) ;
#12926=CARTESIAN_POINT ( 'NONE',  ( -0.1153557615297513411, -0.4303681241737880026, -1.934055118110236338 ) ) ;
#12927=CARTESIAN_POINT ( 'NONE',  ( -0.02438677169350799909, 0.3726024258163779246, -3.115157480314960647 ) ) ;
#12929=CARTESIAN_POINT ( 'NONE',  ( -0.4724409448465559103, 0.000000000000000000, 1.953740157480315043 ) ) ;
#12942=CARTESIAN_POINT ( 'NONE',  ( 0.03349795313264414959, -0.5118110236220471121, 1.766732283464566899 ) ) ;
#12944=CARTESIAN_POINT ( 'NONE',  ( -0.3382184156732160329, -0.3855916753051698009, 1.747047244094488194 ) ) ;
#12946=ORIENTED_EDGE ( 'NONE', *, *, #4001, .F. ) ;
#12949=CARTESIAN_POINT ( 'NONE',  ( -0.3574975638436101444, 0.000000000000000000, -3.115157480314960647 ) ) ;
#12955=CARTESIAN_POINT ( 'NONE',  ( 0.2660793235464269380, 0.2041304421298361926, 1.973425196850393970 ) ) ;
#12961=ORIENTED_EDGE ( 'NONE', *, *, #18615, .F. ) ;
#12970=B_SPLINE_SURFACE_WITH_KNOTS ( 'NONE', 2, 3, ( 
 ( #14350, #11794, #22963, #5583 ),
 ( #25069, #11940, #5147, #1073 ),
 ( #13774, #27058, #26911, #5733 ) ),
 .UNSPECIFIED., .F., .F., .F.,
 ( 3, 3 ),
 ( 4, 4 ),
 ( 0.000000000000000000, 1.000000000000000000 ),
 ( -0.006999999999999992339, -1.387778780781445676E-17 ),
 .UNSPECIFIED. ) ;
#12980=ADVANCED_FACE ( 'NONE', ( #9979 ), #22312, .F. ) ;
#12992=CARTESIAN_POINT ( 'NONE',  ( -0.1775991818008590406, -0.5230301363771331369, 0.9202755905511811330 ) ) ;
#13012=CARTESIAN_POINT ( 'NONE',  ( 0.1480156394741987402, 0.5526079293737075071, 0.9399606299212598381 ) ) ;
#13024=CARTESIAN_POINT ( 'NONE',  ( 0.4600326175570071952, 0.2268096725200290653, -1.550196850393700920 ) ) ;
#13025=CARTESIAN_POINT ( 'NONE',  ( -0.5130740159360542840, -0.2530785775248223235, 0.9399606299212598381 ) ) ;
#13044=CARTESIAN_POINT ( 'NONE',  ( 0.03220957031753989008, 0.4921259842519685179, -1.550196850393700920 ) ) ;
#13047=CARTESIAN_POINT ( 'NONE',  ( 0.1458850421962665789, 0.4296318976990154970, -1.934055118110236338 ) ) ;
#13059=CARTESIAN_POINT ( 'NONE',  ( -0.3543307086614173596, 4.268512490100411279E-17, 1.953740157480315043 ) ) ;
#13064=CARTESIAN_POINT ( 'NONE',  ( 0.3429980251342297226, -0.09187177619658888628, 1.953740157480315043 ) ) ;
#13066=CARTESIAN_POINT ( 'NONE',  ( -0.1458850421962410715, 0.4296318976989903504, -1.934055118110236338 ) ) ;
#13075=CARTESIAN_POINT ( 'NONE',  ( 0.3233561589689049054, 0.1867299569291689110, -3.115157480314960647 ) ) ;
#13082=CARTESIAN_POINT ( 'NONE',  ( 0.4921259842519685179, 2.987958743070287587E-17, -1.569881889763779625 ) ) ;
#13087=CARTESIAN_POINT ( 'NONE',  ( 0.06699590632655395839, 0.5118110236220472231, 1.766732283464566899 ) ) ;
#13088=CARTESIAN_POINT ( 'NONE',  ( -0.4954415918530857832, 0.1327036767659614813, 1.766732283464566899 ) ) ;
#13092=CARTESIAN_POINT ( 'NONE',  ( -0.2462256503455939050, 0.2807137536170327685, -3.115157480314960647 ) ) ;
#13097=CARTESIAN_POINT ( 'NONE',  ( -0.04380447413658625222, -0.3324885138898230341, 1.953740157480315043 ) ) ;
#13121=CARTESIAN_POINT ( 'NONE',  ( -0.07669076177803968442, 0.1968503937007873850, -3.252027725244194922 ) ) ;
#13122=EDGE_LOOP ( 'NONE', ( #26926, #12425, #22002, #20164 ) ) ;
#13123=DIRECTION ( 'NONE',  ( -1.000000000000000000, 0.000000000000000000, 0.000000000000000000 ) ) ;
#13125=CARTESIAN_POINT ( 'NONE',  ( -0.3289909311256229429, 0.1896185148830510925, -3.100567304031763172 ) ) ;
#13131=CARTESIAN_POINT ( 'NONE',  ( 0.2762247810519068980, 0.4783323773986306038, 0.9399606299212598381 ) ) ;
#13140=DIRECTION ( 'NONE',  ( 1.000000000000000000, 0.000000000000000000, 0.000000000000000000 ) ) ;
#13168=EDGE_LOOP ( 'NONE', ( #14160, #12613, #13302, #9424 ) ) ;
#13169=CARTESIAN_POINT ( 'NONE',  ( 0.07874328603165660356, 0.3051025194879752878, -3.608678036488587093 ) ) ;
#13173=CARTESIAN_POINT ( 'NONE',  ( -0.1477428134820341077, 0.4351030398461640525, -1.928289503579168285 ) ) ;
#13174=FACE_OUTER_BOUND ( 'NONE', #2081, .T. ) ;
#13176=EDGE_CURVE ( 'NONE', #88, #24094, #3931, .T. ) ;
#13182=CARTESIAN_POINT ( 'NONE',  ( -0.3242071728275051634, -0.4225965726693019509, 1.747047244094488194 ) ) ;
#13193=CARTESIAN_POINT ( 'NONE',  ( 0.3520466617656973218, -0.04638120790932973719, 1.953740157480315043 ) ) ;
#13206=CARTESIAN_POINT ( 'NONE',  ( -0.3535721684717625934, 0.1200583359873131500, -3.115157480314960647 ) ) ;
#13225=CARTESIAN_POINT ( 'NONE',  ( 0.3233561589689052385, -0.1867299569291582528, -3.115157480314960647 ) ) ;
#13233=CARTESIAN_POINT ( 'NONE',  ( -0.3007905576423960392, -0.1482986320106512990, 1.953740157480315043 ) ) ;
#13246=CARTESIAN_POINT ( 'NONE',  ( -0.08582672153403875237, 0.3030863606044028602, -3.598133626470924273 ) ) ;
#13270=CARTESIAN_POINT ( 'NONE',  ( -0.4921259842519685179, 0.000000000000000000, -1.569881889763779625 ) ) ;
#13276=CARTESIAN_POINT ( 'NONE',  ( -0.2442565704126240245, -0.4954197419817664150, 0.9202755905511811330 ) ) ;
#13285=CARTESIAN_POINT ( 'NONE',  ( -0.07870736599818195511, 0.2165354330708661457, -3.608715228723579305 ) ) ;
#13294=CARTESIAN_POINT ( 'NONE',  ( 0.5417097841048533757, -0.1839420097223136985, 0.9399606299212598381 ) ) ;
#13299=ADVANCED_FACE ( 'NONE', ( #22110 ), #15023, .T. ) ;
#13302=ORIENTED_EDGE ( 'NONE', *, *, #19376, .T. ) ;
#13317=CARTESIAN_POINT ( 'NONE',  ( -0.1585706980422252055, -0.4669911931914896841, -1.569881889763779625 ) ) ;
#13320=CARTESIAN_POINT ( 'NONE',  ( 0.1477428134820237549, -0.4351030398461813720, -1.928289503579156294 ) ) ;
#13321=CARTESIAN_POINT ( 'NONE',  ( -0.5335524835332333682, 0.1429116519061236767, 0.9202755905511811330 ) ) ;
#13330=EDGE_CURVE ( 'NONE', #10350, #25, #14031, .T. ) ;
#13345=CARTESIAN_POINT ( 'NONE',  ( -0.2836590635674538508, 0.2488091035917008864, -3.100567304031763172 ) ) ;
#13351=CARTESIAN_POINT ( 'NONE',  ( -0.4446020952038907681, 0.02909913904661337244, -1.934055118110236338 ) ) ;
#13356=CARTESIAN_POINT ( 'NONE',  ( 0.5118110236220472231, 3.133938659235352953E-17, 1.766732283464566899 ) ) ;
#13357=CARTESIAN_POINT ( 'NONE',  ( -0.4069448477556027455, 0.3121994997598392940, 1.747047244094488194 ) ) ;
#13363=CARTESIAN_POINT ( 'NONE',  ( -0.3349073414798397486, -0.1651192144506304638, -3.115157480314960647 ) ) ;
#13367=ORIENTED_EDGE ( 'NONE', *, *, #25098, .F. ) ;
#13374=CARTESIAN_POINT ( 'NONE',  ( -0.2268956277328164628, -0.4599954779396636662, -1.550196850393700920 ) ) ;
#13379=DIRECTION ( 'NONE',  ( 1.000000000000000000, 0.000000000000000000, 0.000000000000000000 ) ) ;
#13380=CARTESIAN_POINT ( 'NONE',  ( -0.06294381634922237290, 0.1968503937007874127, -3.224230184698364976 ) ) ;
#13389=CARTESIAN_POINT ( 'NONE',  ( 0.000000000000000000, 0.000000000000000000, 2.504921259842519898 ) ) ;
#13393=B_SPLINE_CURVE_WITH_KNOTS ( 'NONE', 3,
 ( #10868, #21890, #21752, #11012, #310, #8884, #19764, #17504, #15414, #4639, #431, #15541, #9278, #20036, #7183, #13671, #22291, #14510, #974, #23111, #26663, #27486, #8134, #23257, #11695, #20316, #16088, #13969, #25641, #21540, #17164, #15194, #23806, #13059 ),
 .UNSPECIFIED., .F., .F.,
 ( 4, 2, 2, 2, 2, 2, 2, 2, 2, 2, 2, 2, 2, 2, 2, 2, 4 ),
 ( 0.000000000000000000, 0.03125000000000000000, 0.06250000000000000000, 0.09375000000000000000, 0.1250000000000000000, 0.1562500000000000000, 0.1875000000000000000, 0.2187500000000000278, 0.2500000000000000555, 0.2812500000000000555, 0.3125000000000000555, 0.3437500000000000555, 0.3750000000000000555, 0.4062500000000000555, 0.4375000000000000555, 0.4687500000000000555, 0.5000000000000000000 ),
 .UNSPECIFIED. ) ;
#13394=CARTESIAN_POINT ( 'NONE',  ( -0.07874015748031502893, 0.1968503937007873850, -3.272637795275590733 ) ) ;
#13402=CARTESIAN_POINT ( 'NONE',  ( -0.4783323773986625782, 0.2762247810518428381, 0.9399606299212598381 ) ) ;
#13410=DIRECTION ( 'NONE',  ( -1.000000000000000000, 0.000000000000000000, 0.000000000000000000 ) ) ;
#13417=CARTESIAN_POINT ( 'NONE',  ( 0.4300830224589218820, 0.3772436174784425389, 0.9399606299212598381 ) ) ;
#13418=CARTESIAN_POINT ( 'NONE',  ( 0.5118110236220472231, 3.133938659235352953E-17, 1.766732283464566899 ) ) ;
#13421=CARTESIAN_POINT ( 'NONE',  ( -2.685748425196850164E-17, 0.000000000000000000, -3.745078740157480546 ) ) ;
#13433=ADVANCED_FACE ( 'NONE', ( #9769 ), #6007, .T. ) ;
#13445=CARTESIAN_POINT ( 'NONE',  ( -0.2466292688015021273, -0.4270824798167794922, -1.550196850393700920 ) ) ;
#13447=CARTESIAN_POINT ( 'NONE',  ( 0.4438564651657277427, 0.1188866373884867045, -1.928289503579172726 ) ) ;
#13448=CARTESIAN_POINT ( 'NONE',  ( -0.1429116519061127688, 0.5335524835332354776, 0.9202755905511811330 ) ) ;
#13450=FACE_OUTER_BOUND ( 'NONE', #175, .T. ) ;
#13453=CARTESIAN_POINT ( 'NONE',  ( -0.2297883689023087483, 0.3979194638820583441, -1.928289503579160513 ) ) ;
#13473=CARTESIAN_POINT ( 'NONE',  ( 0.02917857698710651232, -0.4446006764000813294, -1.934055118110236338 ) ) ;
#13474=CARTESIAN_POINT ( 'NONE',  ( -0.1886891683788859964, 0.3267488823401775155, -3.100567304031764948 ) ) ;
#13476=DIRECTION ( 'NONE',  ( 1.000000000000000000, 0.000000000000000000, 0.000000000000000000 ) ) ;
#13479=B_SPLINE_CURVE_WITH_KNOTS ( 'NONE', 3,
 ( #4828, #22067, #19949, #2698, #15332, #23929, #4563, #13169, #21801, #20511, #5099, #17938, #11470, #9619 ),
 .UNSPECIFIED., .F., .F.,
 ( 4, 2, 2, 2, 2, 2, 4 ),
 ( -0.002956005455613042350, -0.002463754750849624520, -0.001971504046086206691, -0.0009870026365593714650, -2.501227032536239292E-06, 0.0004897494777309002387, 0.0009820001824943367166 ),
 .UNSPECIFIED. ) ;
#13483=CARTESIAN_POINT ( 'NONE',  ( -0.4438564651657384008, -0.1188866373884874261, -1.928289503579162067 ) ) ;
#13484=CARTESIAN_POINT ( 'NONE',  ( 0.4465874321618643061, 0.1200170377978878322, -1.928289503579156516 ) ) ;
#13489=CARTESIAN_POINT ( 'NONE',  ( -0.3382184156732160329, -0.3855916753051698009, 1.747047244094488194 ) ) ;
#13495=CARTESIAN_POINT ( 'NONE',  ( 0.2462256503455907131, -0.2807137536170764003, -3.115157480314960647 ) ) ;
#13498=CARTESIAN_POINT ( 'NONE',  ( 0.1482986320106464417, 0.3007905576423925420, 1.953740157480315043 ) ) ;
#13505=VERTEX_POINT ( 'NONE', #23067 ) ;
#13510=CARTESIAN_POINT ( 'NONE',  ( -0.5118110236220473341, 0.000000000000000000, -1.550196850393700920 ) ) ;
#13516=CARTESIAN_POINT ( 'NONE',  ( -0.1141709026133645999, 0.3362336590883638343, 1.953740157480315043 ) ) ;
#13525=CARTESIAN_POINT ( 'NONE',  ( 0.4600326175560556230, 0.2268096725222457644, 1.766732283464566899 ) ) ;
#13537=FACE_OUTER_BOUND ( 'NONE', #5434, .T. ) ;
#13539=CARTESIAN_POINT ( 'NONE',  ( -0.07472527936312116370, 0.5671862884094760471, 0.9399606299212598381 ) ) ;
#13545=FACE_OUTER_BOUND ( 'NONE', #1168, .T. ) ;
#13553=B_SPLINE_CURVE_WITH_KNOTS ( 'NONE', 3,
 ( #9176, #8914, #11869, #12153, #1703, #14028, #18778, #12437, #25474, #6138, #4005, #5309, #12750, #26927, #12618, #6268, #18132, #7567, #12328, #21377, #16195, #10198, #4424, #19675, #13712, #27001, #19940, #7647, #7091, #11318, #13571, #26559, #24584, #18211 ),
 .UNSPECIFIED., .F., .F.,
 ( 4, 2, 2, 2, 2, 2, 2, 2, 2, 2, 2, 2, 2, 2, 2, 2, 4 ),
 ( 0.5000000000000000000, 0.5312500000000000000, 0.5624999999999998890, 0.5937499999999998890, 0.6249999999999998890, 0.6562499999999997780, 0.6874999999999997780, 0.7187499999999997780, 0.7499999999999997780, 0.7812499999999997780, 0.8124999999999997780, 0.8437499999999997780, 0.8749999999999997780, 0.9062499999999997780, 0.9374999999999997780, 0.9687500000000000000, 1.000000000000000000 ),
 .UNSPECIFIED. ) ;
#13557=CARTESIAN_POINT ( 'NONE',  ( -0.2904160862623610950, -0.1677079028045287690, 1.953740157480315043 ) ) ;
#13571=CARTESIAN_POINT ( 'NONE',  ( -0.4954205147796584829, 0.1328023637707214100, -1.550196850393700476 ) ) ;
#13583=CARTESIAN_POINT ( 'NONE',  ( 0.04380447413659061678, 0.3324885138898235892, 1.973425196850393970 ) ) ;
#13585=CARTESIAN_POINT ( 'NONE',  ( 0.06441834428465775808, -0.4889536969034878333, -1.550196850393700920 ) ) ;
#13587=CARTESIAN_POINT ( 'NONE',  ( 0.1188866373884869265, 0.4438564651657460614, -1.928289503579154740 ) ) ;
#13588=CARTESIAN_POINT ( 'NONE',  ( 0.2762247810519147251, 0.4783323773986423166, 0.9202755905511811330 ) ) ;
#13592=CARTESIAN_POINT ( 'NONE',  ( 0.3030032861725032167, 0.3454440660767328364, -1.928289503579165620 ) ) ;
#13593=CARTESIAN_POINT ( 'NONE',  ( -0.4921259842519685179, 0.03220957031763950484, -1.569881889763779625 ) ) ;
#13597=CARTESIAN_POINT ( 'NONE',  ( 0.2938622683360631593, 0.000000000000000000, -3.745078740157480546 ) ) ;
#13605=LINE ( 'NONE', #18384, #5240 ) ;
#13609=CARTESIAN_POINT ( 'NONE',  ( 0.02325127328499142915, 0.3543321272855671222, 1.953740157480314821 ) ) ;
#13620=CARTESIAN_POINT ( 'NONE',  ( 0.04928467685643989765, -0.3740848232703748444, -3.100567304031760507 ) ) ;
#13625=VECTOR ( 'NONE', #2846, 39.37007874015748854 ) ;
#13630=CARTESIAN_POINT ( 'NONE',  ( -0.4856708409200505283, -0.1649135259617098836, 1.747047244094488194 ) ) ;
#13635=CARTESIAN_POINT ( 'NONE',  ( -0.1867299569291481776, 0.3233561589688985771, -3.115157480314960647 ) ) ;
#13638=CARTESIAN_POINT ( 'NONE',  ( -0.4585215200179055817, -0.03001016326912892690, -1.928289503579156516 ) ) ;
#13640=EDGE_CURVE ( 'NONE', #21275, #10141, #22421, .T. ) ;
#13644=CARTESIAN_POINT ( 'NONE',  ( 0.5708661417322835607, 6.829619984160658046E-17, 0.9399606299212598381 ) ) ;
#13647=CARTESIAN_POINT ( 'NONE',  ( 0.1432577568504648236, 0.4218945342797248421, -1.934055118110236338 ) ) ;
#13657=CARTESIAN_POINT ( 'NONE',  ( 0.09842519685039365085, 0.2165354330708660902, -3.259753967135868180 ) ) ;
#13659=CARTESIAN_POINT ( 'NONE',  ( -0.04638120790932924453, 0.3520466617657084796, 1.953740157480315043 ) ) ;
#13666=CARTESIAN_POINT ( 'NONE',  ( 0.3121994997598398491, -0.4069448477555819843, 1.747047244094488194 ) ) ;
#13671=CARTESIAN_POINT ( 'NONE',  ( 0.04632226222394355414, -0.3520598332081320558, 1.953740157480315043 ) ) ;
#13678=CARTESIAN_POINT ( 'NONE',  ( 0.2180862235769348290, -0.4423390553432507977, -1.569881889763779625 ) ) ;
#13679=CARTESIAN_POINT ( 'NONE',  ( -0.3543307086614173596, 4.268512490100411279E-17, 1.953740157480315043 ) ) ;
#13681=CARTESIAN_POINT ( 'NONE',  ( -0.5511811023622048555, -0.03607471876259069760, 0.9399606299212598381 ) ) ;
#13693=CARTESIAN_POINT ( 'NONE',  ( -0.3175540113612211890, 0.1078280746903930443, 1.953740157480315043 ) ) ;
#13698=LINE ( 'NONE', #24855, #18886 ) ;
#13699=CARTESIAN_POINT ( 'NONE',  ( 0.1339654526248284794, -0.4984899526255159308, 1.766732283464566899 ) ) ;
#13710=CARTESIAN_POINT ( 'NONE',  ( 0.09842519685039363697, 0.2165354330708661457, -3.561114497143034630 ) ) ;
#13712=CARTESIAN_POINT ( 'NONE',  ( -0.3381512095065914991, 0.3856568748492081866, -1.550196850393700920 ) ) ;
#13724=CARTESIAN_POINT ( 'NONE',  ( -0.02190250779246035590, 0.3346456692913385988, 1.973425196850393970 ) ) ;
#13726=CARTESIAN_POINT ( 'NONE',  ( -0.4270824798167792147, -0.2466292688015026546, -1.550196850393700920 ) ) ;
#13729=CARTESIAN_POINT ( 'NONE',  ( -0.4783323773986625782, 0.2762247810518428381, 0.9399606299212598381 ) ) ;
#13730=CARTESIAN_POINT ( 'NONE',  ( -0.09842519685039373412, 0.2991866959364303802, -3.272637795275590733 ) ) ;
#13733=CARTESIAN_POINT ( 'NONE',  ( -0.3454440660767217341, 0.3030032861725395210, -1.928289503579147635 ) ) ;
#13735=FACE_OUTER_BOUND ( 'NONE', #17737, .T. ) ;
#13746=ORIENTED_EDGE ( 'NONE', *, *, #18095, .T. ) ;
#13749=CARTESIAN_POINT ( 'NONE',  ( 0.2268989272875726881, 0.3929158813954875540, -1.934055118110236338 ) ) ;
#13752=CARTESIAN_POINT ( 'NONE',  ( 0.09842519685039365085, 0.2991866959364303802, -3.266084890085740877 ) ) ;
#13762=CARTESIAN_POINT ( 'NONE',  ( 0.3765118517642104257, 0.02464264302293800099, -3.100567304031763172 ) ) ;
#13766=CARTESIAN_POINT ( 'NONE',  ( -0.1970259548082058665, 0.3996230174612936392, -1.934055118110236338 ) ) ;
#13769=CARTESIAN_POINT ( 'NONE',  ( -0.1970259548082058665, 0.3996230174612936392, -1.934055118110236338 ) ) ;
#13770=B_SPLINE_CURVE_WITH_KNOTS ( 'NONE', 3,
 ( #14766, #16860, #15030, #25608, #12745, #13025, #21234, #2283, #23371, #10909, #8648, #8782, #2010, #10621, #4000, #17271, #12614, #27877, #10481, #19102, #25890, #4137, #27739, #23643, #6262, #19530, #15315, #215, #14899, #23509, #19247, #4278, #8511, #6536 ),
 .UNSPECIFIED., .F., .F.,
 ( 4, 2, 2, 2, 2, 2, 2, 2, 2, 2, 2, 2, 2, 2, 2, 2, 4 ),
 ( 0.000000000000000000, 0.03125000000000002776, 0.06250000000000005551, 0.09375000000000008327, 0.1250000000000001110, 0.1562500000000001388, 0.1875000000000001388, 0.2187500000000001388, 0.2500000000000001110, 0.2812500000000001110, 0.3125000000000001665, 0.3437500000000001665, 0.3750000000000001665, 0.4062500000000001110, 0.4375000000000001110, 0.4687500000000000555, 0.5000000000000000000 ),
 .UNSPECIFIED. ) ;
#13774=CARTESIAN_POINT ( 'NONE',  ( 0.09842519685039370636, 0.2165354330708661457, -3.272637795275590733 ) ) ;
#13776=CARTESIAN_POINT ( 'NONE',  ( 0.2268096725222443211, -0.4600326175560562336, 1.766732283464566899 ) ) ;
#13778=CARTESIAN_POINT ( 'NONE',  ( -0.5905511811023621549, 7.232166136696967594E-17, 0.9399606299212598381 ) ) ;
#13780=CARTESIAN_POINT ( 'NONE',  ( 0.04877294052296175797, -0.3702005978258584573, -3.115157480314960647 ) ) ;
#13785=ORIENTED_EDGE ( 'NONE', *, *, #5181, .F. ) ;
#13791=CARTESIAN_POINT ( 'NONE',  ( 0.3858397471888842523, 0.2228126397719887297, -1.934055118110236338 ) ) ;
#13799=CARTESIAN_POINT ( 'NONE',  ( 0.07668265949372614354, 0.1968503937007874127, -3.252000825552965324 ) ) ;
#13802=B_SPLINE_CURVE_WITH_KNOTS ( 'NONE', 3,
 ( #4460, #17713, #21697, #258, #11364, #23319, #123, #11092, #25932, #21833, #502, #17314, #26335, #3943, #4858, #381, #13473, #19579, #26067, #12926, #19714, #19980, #636, #15360, #23953, #2326, #5134, #17845, #24624, #16026, #7404, #11781, #778, #1335 ),
 .UNSPECIFIED., .F., .F.,
 ( 4, 2, 2, 2, 2, 2, 2, 2, 2, 2, 2, 2, 2, 2, 2, 2, 4 ),
 ( 0.5000000000000000000, 0.5312500000000000000, 0.5625000000000000000, 0.5937500000000000000, 0.6250000000000001110, 0.6562500000000001110, 0.6875000000000000000, 0.7187500000000001110, 0.7500000000000001110, 0.7812500000000001110, 0.8125000000000002220, 0.8437500000000002220, 0.8750000000000002220, 0.9062500000000002220, 0.9375000000000001110, 0.9687500000000001110, 1.000000000000000000 ),
 .UNSPECIFIED. ) ;
#13807=CARTESIAN_POINT ( 'NONE',  ( -0.2669480828848092013, 0.2341512108694271399, 1.953740157480315043 ) ) ;
#13815=CARTESIAN_POINT ( 'NONE',  ( 0.4069448477556118493, -0.3121994997598555033, 1.747047244094488194 ) ) ;
#13816=CARTESIAN_POINT ( 'NONE',  ( 0.1327036767659630079, 0.4954415918530855056, 1.766732283464566899 ) ) ;
#13826=CARTESIAN_POINT ( 'NONE',  ( 0.4763861460130340286, 0.1275996891957706103, -1.569881889763779625 ) ) ;
#13828=CARTESIAN_POINT ( 'NONE',  ( -0.4300830224589641260, 0.3772436174784328244, 0.9399606299212598381 ) ) ;
#13830=PLANE ( 'NONE',  #1789 ) ;
#13831=CARTESIAN_POINT ( 'NONE',  ( 0.09842519685039355370, 0.5905905511811023745, -3.548228346456693050 ) ) ;
#13841=CARTESIAN_POINT ( 'NONE',  ( 0.3175540113612412840, -0.1078280746903980958, 1.953740157480315043 ) ) ;
#13868=ORIENTED_EDGE ( 'NONE', *, *, #12749, .F. ) ;
#13870=CARTESIAN_POINT ( 'NONE',  ( -0.1482986320106437217, -0.3007905576423873795, 1.973425196850393970 ) ) ;
#13871=CARTESIAN_POINT ( 'NONE',  ( -0.1275996891957763835, -0.4763861460130486281, -1.550196850393700920 ) ) ;
#13875=CARTESIAN_POINT ( 'NONE',  ( 0.5476281405333178753, -0.07214854559198131956, 0.9202755905511811330 ) ) ;
#13880=CARTESIAN_POINT ( 'NONE',  ( 0.1896185148830505929, -0.3289909311256231650, -3.100567304031763172 ) ) ;
#13887=CYLINDRICAL_SURFACE ( 'NONE', #324, 0.5511811023622047445 ) ;
#13892=CARTESIAN_POINT ( 'NONE',  ( -0.3362554559023691048, 0.1141145734058716110, 1.953740157480314599 ) ) ;
#13895=CARTESIAN_POINT ( 'NONE',  ( 0.3599896729929407679, 0.2761764805255620403, -1.934055118110236338 ) ) ;
#13898=CARTESIAN_POINT ( 'NONE',  ( -0.03189542488298714729, 0.3133998791825584607, -3.179296722889725757 ) ) ;
#13900=VECTOR ( 'NONE', #1152, 39.37007874015748854 ) ;
#13908=CARTESIAN_POINT ( 'NONE',  ( -0.1213180142433868958, -0.3572819248074448062, -3.100567304031760951 ) ) ;
#13913=CARTESIAN_POINT ( 'NONE',  ( -0.4069519308876554664, 0.2006393256663590030, -1.934055118110236338 ) ) ;
#13922=CARTESIAN_POINT ( 'NONE',  ( 0.4069448477555986377, -0.3121994997598466770, 1.766732283464566899 ) ) ;
#13924=CARTESIAN_POINT ( 'NONE',  ( 0.3267488823401750175, 0.1886891683788910201, -3.100567304031762284 ) ) ;
#13936=CARTESIAN_POINT ( 'NONE',  ( 0.02909913904661943010, -0.4446020952038907681, -1.934055118110236338 ) ) ;
#13938=LINE ( 'NONE', #3180, #25376 ) ;
#13946=DIRECTION ( 'NONE',  ( 1.000000000000000000, 0.000000000000000000, 0.000000000000000000 ) ) ;
#13951=B_SPLINE_CURVE_WITH_KNOTS ( 'NONE', 3,
 ( #12545, #4072, #8038, #10414, #12677, #8583, #27529, #1805, #8442, #14694, #23300, #23150, #1665, #14404, #21164, #10135, #21305, #12815 ),
 .UNSPECIFIED., .F., .F.,
 ( 4, 2, 2, 2, 2, 2, 2, 2, 4 ),
 ( 0.000000000000000000, 0.06250000000000001388, 0.1250000000000000000, 0.1875000000000000000, 0.2500000000000000000, 0.3125000000000000000, 0.3749999999999999445, 0.4375000000000000000, 0.5000000000000000000 ),
 .UNSPECIFIED. ) ;
#13952=CARTESIAN_POINT ( 'NONE',  ( -0.1141709026133623378, -0.3362336590883613363, 1.953740157480315043 ) ) ;
#13955=CARTESIAN_POINT ( 'NONE',  ( 0.5511811023268710086, 6.750021727151124356E-17, 1.747047244094488194 ) ) ;
#13958=AXIS2_PLACEMENT_3D ( 'NONE', #1834, #8199, #27834 ) ;
#13962=CARTESIAN_POINT ( 'NONE',  ( -0.1378076643338909391, 0.5144970376935737999, 1.747047244094488194 ) ) ;
#13967=CARTESIAN_POINT ( 'NONE',  ( -0.3535065162672771932, 0.2712027394948494652, -1.934055118110236338 ) ) ;
#13969=CARTESIAN_POINT ( 'NONE',  ( -0.3075341118175178856, -0.1775236553383595373, 1.953740157480314821 ) ) ;
#13975=EDGE_LOOP ( 'NONE', ( #9830, #18021 ) ) ;
#13976=CARTESIAN_POINT ( 'NONE',  ( -0.3707612262532960501, 0.3252100150720461658, -1.569881889763779625 ) ) ;
#13990=CARTESIAN_POINT ( 'NONE',  ( -0.3346456692913385988, -0.02190250779246036283, 1.953740157480315043 ) ) ;
#14005=CARTESIAN_POINT ( 'NONE',  ( 0.09586345222254320786, 0.1968503937007873850, -3.573990933995919939 ) ) ;
#14017=CARTESIAN_POINT ( 'NONE',  ( -0.04380447413658627998, 0.3324885138898243664, 1.973425196850393970 ) ) ;
#14018=CARTESIAN_POINT ( 'NONE',  ( -0.2564944395535840860, 0.4441657790094369895, -1.550196850393700920 ) ) ;
#14021=CARTESIAN_POINT ( 'NONE',  ( -0.3642352168757148623, 0.4152525734086685016, 0.9399606299212598381 ) ) ;
#14027=CARTESIAN_POINT ( 'NONE',  ( 0.2313841235333768398, -0.3010840436257779529, -3.100567304031764060 ) ) ;
#14028=CARTESIAN_POINT ( 'NONE',  ( 0.4599980997183205633, 0.2268967137093434727, -1.550196850393700920 ) ) ;
#14031=B_SPLINE_CURVE_WITH_KNOTS ( 'NONE', 3,
 ( #15997, #18512, #7374, #9475, #25023, #20651, #18226, #7663, #26864, #22768, #24884, #20790, #5690, #3539, #27016, #1304, #9911, #12036 ),
 .UNSPECIFIED., .F., .F.,
 ( 4, 2, 2, 2, 2, 2, 2, 2, 4 ),
 ( 0.000000000000000000, 0.06250000000000000000, 0.1250000000000000000, 0.1875000000000000000, 0.2500000000000000000, 0.3125000000000000000, 0.3750000000000000000, 0.4375000000000000000, 0.5000000000000000000 ),
 .UNSPECIFIED. ) ;
#14041=CARTESIAN_POINT ( 'NONE',  ( 0.04632170870412826574, 0.3520570504768268383, 1.953740157480315043 ) ) ;
#14043=CARTESIAN_POINT ( 'NONE',  ( 0.05926487674657893168, 0.4498374011143063678, -1.934055118110236338 ) ) ;
#14052=CARTESIAN_POINT ( 'NONE',  ( -0.1886891683788906593, -0.3267488823401751841, -3.100567304031762284 ) ) ;
#14056=CARTESIAN_POINT ( 'NONE',  ( -0.05819755867303792046, 0.4417361510194100505, -1.934055118110236338 ) ) ;
#14063=CARTESIAN_POINT ( 'NONE',  ( 0.4069448477556118493, -0.3121994997598555033, 1.747047244094488194 ) ) ;
#14067=CARTESIAN_POINT ( 'NONE',  ( 0.3384212623783066642, -0.1668516812751465739, -3.100567304031770277 ) ) ;
#14072=ORIENTED_EDGE ( 'NONE', *, *, #11791, .T. ) ;
#14088=ORIENTED_EDGE ( 'NONE', *, *, #7028, .F. ) ;
#14089=LINE ( 'NONE', #15926, #20915 ) ;
#14097=CARTESIAN_POINT ( 'NONE',  ( 0.4777261797697469614, 0.2355331214654221850, 1.747047244094488194 ) ) ;
#14099=CARTESIAN_POINT ( 'NONE',  ( 0.4069448477555425714, 0.3121994997598541155, 1.747047244094488194 ) ) ;
#14107=CARTESIAN_POINT ( 'NONE',  ( 0.3239425792934412240, 0.08676778863010829734, 1.973425196850393970 ) ) ;
#14110=B_SPLINE_CURVE_WITH_KNOTS ( 'NONE', 3,
 ( #16745, #4310, #12018, #25506, #14931, #6172, #2045, #12780, #113, #12917, #10804, #6297, #8548, #17166, #19281, #25783, #21125, #14656, #25357, #10378, #21407, #17301, #10517, #4450, #21543, #20981, #6432, #14798, #2187, #15067, #18998, #23259, #1627, #3889 ),
 .UNSPECIFIED., .F., .F.,
 ( 4, 2, 2, 2, 2, 2, 2, 2, 2, 2, 2, 2, 2, 2, 2, 2, 4 ),
 ( 0.000000000000000000, 0.03125000000000001388, 0.06250000000000001388, 0.09375000000000001388, 0.1250000000000000000, 0.1562500000000000000, 0.1875000000000000278, 0.2187500000000000278, 0.2500000000000000555, 0.2812500000000000555, 0.3125000000000000555, 0.3437500000000001110, 0.3750000000000001110, 0.4062500000000000555, 0.4375000000000000000, 0.4687500000000000555, 0.5000000000000000000 ),
 .UNSPECIFIED. ) ;
#14111=CARTESIAN_POINT ( 'NONE',  ( -0.3001918266902143251, 0.3912931228432222075, -1.569881889763779625 ) ) ;
#14113=ORIENTED_EDGE ( 'NONE', *, *, #22449, .T. ) ;
#14125=VERTEX_POINT ( 'NONE', #9006 ) ;
#14127=CARTESIAN_POINT ( 'NONE',  ( -0.08676778863011463949, -0.3239425792934414461, 1.953740157480315043 ) ) ;
#14151=CARTESIAN_POINT ( 'NONE',  ( 0.07874015748031480688, 0.1968503937007873850, -3.548228346456692162 ) ) ;
#14158=CARTESIAN_POINT ( 'NONE',  ( 0.09855118063547688156, 0.3667122560601321357, -3.100567304031763172 ) ) ;
#14160=ORIENTED_EDGE ( 'NONE', *, *, #13640, .F. ) ;
#14163=CARTESIAN_POINT ( 'NONE',  ( -0.3175540113612297932, -0.1078280746904006077, 1.973425196850393970 ) ) ;
#14164=CARTESIAN_POINT ( 'NONE',  ( -0.4441657790094409863, -0.2564944395535778687, -1.550196850393700920 ) ) ;
#14165=CARTESIAN_POINT ( 'NONE',  ( -2.685748425196850164E-17, 0.000000000000000000, -3.115157480314960647 ) ) ;
#14169=CARTESIAN_POINT ( 'NONE',  ( 0.4152525734086270348, -0.3642352168757560515, 0.9202755905511811330 ) ) ;
#14177=CARTESIAN_POINT ( 'NONE',  ( 0.06441834428467232976, 0.4889536969035311875, -1.569881889763779625 ) ) ;
#14187=CARTESIAN_POINT ( 'NONE',  ( 0.3520612535909328211, 0.04631512375351633237, 1.953740157480315487 ) ) ;
#14190=CARTESIAN_POINT ( 'NONE',  ( 0.02963280468032102044, 0.4527559054764770385, -1.934055118110236338 ) ) ;
#14193=CARTESIAN_POINT ( 'NONE',  ( 0.06046764050538371016, 0.3092437473714230722, -3.193908385656448523 ) ) ;
#14196=CARTESIAN_POINT ( 'NONE',  ( 0.07874015748031495954, 0.1968503937007874127, -3.548228346456692162 ) ) ;
#14205=CARTESIAN_POINT ( 'NONE',  ( -0.2228126397720058549, -0.3858397471888898589, -1.934055118110236338 ) ) ;
#14207=EDGE_CURVE ( 'NONE', #5007, #21690, #14089, .T. ) ;
#14215=CARTESIAN_POINT ( 'NONE',  ( 0.4856708409200665155, -0.1649135259616916482, 1.747047244094488194 ) ) ;
#14219=CARTESIAN_POINT ( 'NONE',  ( -0.3384212623783144913, -0.1668516812751341671, -3.100567304031760951 ) ) ;
#14223=CARTESIAN_POINT ( 'NONE',  ( 0.3346456692913385988, 0.000000000000000000, 1.953740157480315043 ) ) ;
#14229=CARTESIAN_POINT ( 'NONE',  ( 0.2228126397719881469, 0.3858397471888846408, -1.934055118110236338 ) ) ;
#14235=CARTESIAN_POINT ( 'NONE',  ( 0.09269288654273812045, -0.3460635936744816399, -3.115157480314960647 ) ) ;
#14239=DIRECTION ( 'NONE',  ( -0.000000000000000000, -0.000000000000000000, -1.000000000000000000 ) ) ;
#14241=PLANE ( 'NONE',  #6506 ) ;
#14246=VECTOR ( 'NONE', #17692, 39.37007874015748143 ) ;
#14252=CARTESIAN_POINT ( 'NONE',  ( -0.5043504886477523375, 0.1712563538833050680, 1.747047244094488194 ) ) ;
#14254=CARTESIAN_POINT ( 'NONE',  ( 0.4954415918530851726, -0.1327036767659643957, 1.766732283464566899 ) ) ;
#14256=CARTESIAN_POINT ( 'NONE',  ( -0.09269288654274109029, 0.3460635936744927421, -3.115157480314960647 ) ) ;
#14267=CARTESIAN_POINT ( 'NONE',  ( -0.4889536969035310210, -0.06441834428467370366, -1.569881889763779625 ) ) ;
#14281=EDGE_CURVE ( 'NONE', #285, #18101, #9705, .T. ) ;
#14291=CARTESIAN_POINT ( 'NONE',  ( 0.3726024258163779246, 0.000000000000000000, -3.115157480314960647 ) ) ;
#14309=B_SPLINE_SURFACE_WITH_KNOTS ( 'NONE', 2, 3, ( 
 ( #1311, #13593, #17825, #2843, #18233, #7379, #20521, #7237, #11480, #3400, #2981, #24458, #1037, #16149, #5408, #9778, #752, #1177, #14177, #26871, #9340, #18371, #9483, #15853, #7523, #17948, #7670, #18079, #24747, #16287, #5547, #12042, #20659, #27443, #16419, #25490, #3874, #16883, #12204, #16315, #18688, #16584, #5866, #12491, #8119, #23095, #1338, #3725, #20967, #1611, #10640, #21530, #13317, #21802, #2440, #24055, #26177, #2172, #17151, #17565, #21945, #19546, #8801, #14916, #4156, #8398 ),
 ( #25767, #25908, #17418, #21392, #23795, #26041, #2569, #19406, #15182, #11065, #99, #8665, #6417, #15049, #27755, #6557, #4439, #13044, #2297, #19263, #17016, #2028, #23664, #6694, #4295, #15334, #23930, #19690, #360, #15458, #15593, #3119, #24738, #17817, #11748, #24322, #4972, #7228, #20085, #2972, #9070, #5399, #11335, #11607, #18071, #3251, #605, #13585, #888, #477, #26435, #13871, #22069, #24595, #13445, #24195, #20367, #26715, #22206, #13726, #2834, #9474, #20228, #26862, #1025, #9620 ),
 ( #11471, #742, #22346, #7373, #15996, #7514, #19815, #5250, #16142, #9331, #17683, #14018, #17939, #26569, #22491, #6971, #22630, #15848, #2700, #26306, #19951, #4829, #24448, #5100, #14601, #1716, #10179, #21067, #1303, #25452, #27159, #25022, #22766, #8088, #23066, #22919, #8225, #6117, #9768, #18652, #3392, #5687, #18510, #5832, #18797, #27433, #3839, #23359, #16700, #14754, #1434, #11892, #23205, #7801, #9909, #14455, #27015, #25312, #16408, #14164, #20512, #12035, #24882, #5971, #3538, #12459 ) ),
 .UNSPECIFIED., .F., .T., .F.,
 ( 3, 3 ),
 ( 4, 2, 2, 2, 2, 2, 2, 2, 2, 2, 2, 2, 2, 2, 2, 2, 2, 2, 2, 2, 2, 2, 2, 2, 2, 2, 2, 2, 2, 2, 2, 2, 4 ),
 ( 0.000000000000000000, 1.000000000000000000 ),
 ( 0.000000000000000000, 0.1963495408493620697, 0.3926990816987241395, 0.5890486225480862092, 0.7853981633974482790, 0.9817477042468103487, 1.178097245096172418, 1.374446785945534488, 1.570796326794896558, 1.767145867644258628, 1.963495408493620697, 2.159844949342982545, 2.356194490192344837, 2.552544031041707129, 2.748893571891068976, 2.945243112740430824, 3.141592653589793116, 3.337942194439155408, 3.534291735288517255, 3.730641276137879103, 3.926990816987241395, 4.123340357836603687, 4.319689898685965090, 4.516039439535327382, 4.712388980384689674, 4.908738521234051966, 5.105088062083414258, 5.301437602932775661, 5.497787143782137953, 5.694136684631500245, 5.890486225480861648, 6.086835766330223940, 6.283185307179586232 ),
 .UNSPECIFIED. ) ;
#14342=CARTESIAN_POINT ( 'NONE',  ( 0.3349573549949907414, 0.2938049579018708890, -1.934055118110236338 ) ) ;
#14350=CARTESIAN_POINT ( 'NONE',  ( 0.07874015748031495954, 0.1968503937007873850, -3.272637795275590733 ) ) ;
#14352=CARTESIAN_POINT ( 'NONE',  ( -0.2663596103035606455, 0.4612490782034870396, 1.747047244094488194 ) ) ;
#14357=CARTESIAN_POINT ( 'NONE',  ( 0.3765118517642104257, 0.02464264302293800099, -3.100567304031763172 ) ) ;
#14358=CYLINDRICAL_SURFACE ( 'NONE', #27789, 0.5511811023622047445 ) ;
#14360=CARTESIAN_POINT ( 'NONE',  ( -0.1775730735577547292, 0.3074993854542629190, 1.953740157480315043 ) ) ;
#14363=EDGE_CURVE ( 'NONE', #5266, #19648, #17657, .T. ) ;
#14366=CARTESIAN_POINT ( 'NONE',  ( -0.03736310157557561074, 0.5708661417322835607, 0.9399606299212598381 ) ) ;
#14376=CARTESIAN_POINT ( 'NONE',  ( -0.3213305936751578717, -0.1584254766472200371, -3.115157480314960647 ) ) ;
#14377=CARTESIAN_POINT ( 'NONE',  ( -0.5511811023622046335, -0.07214943758244286853, 0.9202755905511811330 ) ) ;
#14383=B_SPLINE_CURVE_WITH_KNOTS ( 'NONE', 3,
 ( #18980, #18828, #3430, #5577, #10083, #11930, #1609, #12068, #18402, #24775, #27051, #20549, #5864, #9943, #10214, #14641, #14489, #16726, #18547, #21107, #27194, #27468, #7700, #7841, #8117, #16583, #16446, #23239, #5724, #1749, #5440, #3568, #12202, #25198 ),
 .UNSPECIFIED., .F., .F.,
 ( 4, 2, 2, 2, 2, 2, 2, 2, 2, 2, 2, 2, 2, 2, 2, 2, 4 ),
 ( 0.5000000000000000000, 0.5312500000000000000, 0.5625000000000000000, 0.5937500000000000000, 0.6250000000000000000, 0.6562500000000000000, 0.6875000000000000000, 0.7187500000000000000, 0.7500000000000000000, 0.7812500000000000000, 0.8125000000000001110, 0.8437500000000000000, 0.8750000000000000000, 0.9062500000000000000, 0.9375000000000000000, 0.9687500000000000000, 1.000000000000000000 ),
 .UNSPECIFIED. ) ;
#14396=CARTESIAN_POINT ( 'NONE',  ( -0.3855916753051397139, 0.3382184156732160329, 1.766732283464566899 ) ) ;
#14404=CARTESIAN_POINT ( 'NONE',  ( 0.3666644560843324574, -0.2817828961649161967, -1.928289503579156294 ) ) ;
#14409=CARTESIAN_POINT ( 'NONE',  ( -0.4423390553432706152, 0.2180862235769438773, -1.550196850393700920 ) ) ;
#14454=CARTESIAN_POINT ( 'NONE',  ( 0.3175540113612289050, 0.1078280746903826914, 1.953740157480315043 ) ) ;
#14455=CARTESIAN_POINT ( 'NONE',  ( -0.3121994997578409481, -0.4069448477569437284, -1.550196850393700920 ) ) ;
#14459=CARTESIAN_POINT ( 'NONE',  ( -0.5526079293737016229, 0.1480156394741962422, 0.9399606299212598381 ) ) ;
#14466=CARTESIAN_POINT ( 'NONE',  ( -0.4004902621171045896, 0.3511566718596346726, 1.747047244094488194 ) ) ;
#14489=CARTESIAN_POINT ( 'NONE',  ( 0.02345921195929052613, -0.3574961452116294791, -3.115157480314960647 ) ) ;
#14492=CARTESIAN_POINT ( 'NONE',  ( 0.3996230174612964148, -0.1970259548082136380, -1.934055118110236338 ) ) ;
#14503=CARTESIAN_POINT ( 'NONE',  ( 0.4004221243553300891, 0.3512268162760394108, 1.747047244094488194 ) ) ;
#14504=EDGE_CURVE ( 'NONE', #88, #7980, #16977, .T. ) ;
#14508=CARTESIAN_POINT ( 'NONE',  ( 0.3644697409450285974, -0.09762295995069371346, -3.100567304031760951 ) ) ;
#14510=CARTESIAN_POINT ( 'NONE',  ( -0.02325127328526653894, -0.3543321272855305404, 1.953740157480315043 ) ) ;
#14513=CARTESIAN_POINT ( 'NONE',  ( 0.2161381151963047975, 0.2817310484609297228, 1.953740157480315043 ) ) ;
#14516=CARTESIAN_POINT ( 'NONE',  ( -0.04928528614549732706, -0.3765118517642104257, -3.100567304031763616 ) ) ;
#14517=CARTESIAN_POINT ( 'NONE',  ( 0.3772436174784756235, 0.4300830224589536899, 0.9399606299212598381 ) ) ;
#14525=CARTESIAN_POINT ( 'NONE',  ( 0.3574975638436101444, -0.02339816079119092299, -3.115157480314960647 ) ) ;
#14526=CARTESIAN_POINT ( 'NONE',  ( 0.5511811023622046335, -0.07214943758244278527, 0.9202755905511811330 ) ) ;
#14541=CARTESIAN_POINT ( 'NONE',  ( -0.03478633594543645985, -0.5314960629921260393, 1.747047244094488194 ) ) ;
#14546=CARTESIAN_POINT ( 'NONE',  ( -0.4441657790107740866, 0.2564944395515753039, 1.766732283464566899 ) ) ;
#14550=CARTESIAN_POINT ( 'NONE',  ( -0.1584254766472275311, 0.3213305936751604253, -3.115157480314960647 ) ) ;
#14556=CARTESIAN_POINT ( 'NONE',  ( 0.2211428102655756955, 0.2521176338356569957, 1.973425196850393970 ) ) ;
#14560=CARTESIAN_POINT ( 'NONE',  ( -0.2466292688015021273, -0.4270824798167794922, -1.550196850393700920 ) ) ;
#14562=CARTESIAN_POINT ( 'NONE',  ( -0.5708661417322834497, 0.000000000000000000, 0.9399606299212598381 ) ) ;
#14568=PRODUCT ( 'Cam Shaft', 'Cam Shaft', '', ( #2483 ) ) ;
#14570=CIRCLE ( 'NONE', #2344, 0.3149606299212598381 ) ;
#14588=DIRECTION ( 'NONE',  ( 0.000000000000000000, 0.000000000000000000, 1.000000000000000000 ) ) ;
#14589=CARTESIAN_POINT ( 'NONE',  ( -0.2762247810519002922, 0.4783323773986519201, 0.9202755905511811330 ) ) ;
#14600=CARTESIAN_POINT ( 'NONE',  ( 0.5118110236220473341, 6.402768735150616610E-17, -1.550196850393700920 ) ) ;
#14601=CARTESIAN_POINT ( 'NONE',  ( 0.3382184156748877513, 0.3855916753034390188, -1.550196850393700920 ) ) ;
#14608=CARTESIAN_POINT ( 'NONE',  ( 0.4152525734085952824, 0.3642352168757231889, 0.9399606299212598381 ) ) ;
#14611=CARTESIAN_POINT ( 'NONE',  ( -0.3392608232658738676, 0.1151343661288097980, -3.115157480314960647 ) ) ;
#14617=B_SPLINE_CURVE_WITH_KNOTS ( 'NONE', 3,
 ( #11402, #13657, #9403, #22276, #22140, #15922, #674, #26646, #17878, #9264, #7167, #2908, #7587, #6043, #11967, #1785, #9840, #18440 ),
 .UNSPECIFIED., .F., .F.,
 ( 4, 2, 2, 2, 2, 2, 2, 2, 4 ),
 ( 0.000000000000000000, 0.1250000000000000000, 0.2500000000000000000, 0.3750000000000000000, 0.5000000000000000000, 0.6250000000000000000, 0.7500000000000000000, 0.8750000000000000000, 1.000000000000000000 ),
 .UNSPECIFIED. ) ;
#14619=CARTESIAN_POINT ( 'NONE',  ( -0.06699507805604322519, 0.5085118447796660446, -1.550196850393700920 ) ) ;
#14641=CARTESIAN_POINT ( 'NONE',  ( 0.04673614183192328908, -0.3552064049865930051, -3.115157480314960203 ) ) ;
#14642=CARTESIAN_POINT ( 'NONE',  ( -0.1173917140416368271, -0.4382752542996092293, -1.934055118110236338 ) ) ;
#14643=CARTESIAN_POINT ( 'NONE',  ( 0.4555658499975999698, -0.06001958459475366381, -1.928289503579165398 ) ) ;
#14649=CARTESIAN_POINT ( 'NONE',  ( -0.4612490782034870396, -0.2663596103035605345, 1.747047244094488194 ) ) ;
#14656=CARTESIAN_POINT ( 'NONE',  ( 0.02917857698688243462, 0.4446035140077004844, -1.934055118110236338 ) ) ;
#14657=CARTESIAN_POINT ( 'NONE',  ( 0.2341512108694336625, 0.2669480828848126985, 1.953740157480315043 ) ) ;
#14663=CARTESIAN_POINT ( 'NONE',  ( 0.4539000224941021067, -0.3482225189666773302, 0.9399606299212598381 ) ) ;
#14670=CARTESIAN_POINT ( 'NONE',  ( 0.3392387706403792169, -0.1151913129404410208, -3.115157480314960647 ) ) ;
#14671=CARTESIAN_POINT ( 'NONE',  ( 0.3387265385688508768, -0.4407612517155324316, 0.9202755905511812440 ) ) ;
#14679=CARTESIAN_POINT ( 'NONE',  ( -0.4954757973260912052, 0.2860025288262565413, 0.9399606299212600602 ) ) ;
#14686=CARTESIAN_POINT ( 'NONE',  ( 0.4225965726693019509, -0.3242071728275352505, 1.747047244094488194 ) ) ;
#14688=CARTESIAN_POINT ( 'NONE',  ( 0.5085118447801426633, -0.06699507805369582514, 1.766732283464566899 ) ) ;
#14692=CARTESIAN_POINT ( 'NONE',  ( -0.1584254766472190379, -0.3213305936751582048, -3.115157480314960647 ) ) ;
#14694=CARTESIAN_POINT ( 'NONE',  ( 0.06002032661671147240, -0.4585215200179057482, -1.928289503579156516 ) ) ;
#14697=CARTESIAN_POINT ( 'NONE',  ( -0.2521176338356572177, -0.2211428102655754180, 1.973425196850393970 ) ) ;
#14702=CARTESIAN_POINT ( 'NONE',  ( 0.2466292688015071233, 0.4270824798167958125, -1.550196850393700920 ) ) ;
#14728=LINE ( 'NONE', #16955, #654 ) ;
#14738=CARTESIAN_POINT ( 'NONE',  ( -0.07214854559198219386, 0.5476281405333177643, 0.9202755905511811330 ) ) ;
#14753=CARTESIAN_POINT ( 'NONE',  ( 0.3346456692913385988, 0.02190250779246873461, 1.953740157480315043 ) ) ;
#14754=CARTESIAN_POINT ( 'NONE',  ( -0.03349795313024241800, -0.5118110236220473341, -1.550196850393700920 ) ) ;
#14756=CARTESIAN_POINT ( 'NONE',  ( -0.1429116519061139623, 0.5335524835332415838, 0.9399606299212598381 ) ) ;
#14760=CARTESIAN_POINT ( 'NONE',  ( -0.3574975638436101999, 0.02346634615888416181, -3.115157480314961091 ) ) ;
#14766=CARTESIAN_POINT ( 'NONE',  ( -0.5708661417322834497, 0.000000000000000000, 0.9399606299212598381 ) ) ;
#14769=CARTESIAN_POINT ( 'NONE',  ( 0.5043865966252626398, -0.1711654737000346815, 1.747047244094488416 ) ) ;
#14784=CARTESIAN_POINT ( 'NONE',  ( 0.05926487674657893168, 0.4498374011143063678, -1.934055118110236338 ) ) ;
#14785=CARTESIAN_POINT ( 'NONE',  ( 0.4585215200179055817, 0.03001016326913595253, -1.928289503579156516 ) ) ;
#14798=CARTESIAN_POINT ( 'NONE',  ( 0.3858850602361924564, 0.2227473777836185831, -1.934055118110236116 ) ) ;
#14800=CARTESIAN_POINT ( 'NONE',  ( 0.09187177619658809524, -0.3429980251342298336, 1.953740157480315043 ) ) ;
#14810=CARTESIAN_POINT ( 'NONE',  ( 0.3349073414798194315, 0.1651192144506304638, -3.115157480314960647 ) ) ;
#14819=CARTESIAN_POINT ( 'NONE',  ( 0.2530774914995135849, 0.5130713940405263740, 0.9399606299212600602 ) ) ;
#14825=CARTESIAN_POINT ( 'NONE',  ( -0.1649135259617106886, 0.4856708409200803378, 1.747047244094488194 ) ) ;
#14829=CARTESIAN_POINT ( 'NONE',  ( 0.09269288654273812045, -0.3460635936744816399, -3.115157480314960647 ) ) ;
#14834=CARTESIAN_POINT ( 'NONE',  ( 0.02190250779246040100, 0.3346456692913385988, 1.973425196850393970 ) ) ;
#14837=AXIS2_PLACEMENT_3D ( 'NONE', #26439, #1031, #5404 ) ;
#14848=AXIS2_PLACEMENT_3D ( 'NONE', #5321, #11817, #9399 ) ;
#14860=CARTESIAN_POINT ( 'NONE',  ( -0.01030706208231672687, 0.1968503937007873850, -3.193897637795275912 ) ) ;
#14866=EDGE_CURVE ( 'NONE', #14958, #17898, #4162, .T. ) ;
#14874=CARTESIAN_POINT ( 'NONE',  ( 0.5335524835332355886, 0.1429116519061127411, 0.9202755905511811330 ) ) ;
#14883=CARTESIAN_POINT ( 'NONE',  ( -0.04956879678459434613, 0.2165354330708661457, -3.634230943941107572 ) ) ;
#14889=CARTESIAN_POINT ( 'NONE',  ( -0.5131133041953912510, 0.2529800193559492705, 0.9399606299212598381 ) ) ;
#14892=CARTESIAN_POINT ( 'NONE',  ( 0.3392634445559961631, 0.1151354519027797119, -3.115157480314959759 ) ) ;
#14898=CARTESIAN_POINT ( 'NONE',  ( 0.3855916753034099864, -0.3382184156749167836, -1.550196850393700920 ) ) ;
#14899=CARTESIAN_POINT ( 'NONE',  ( 0.5130713940404153517, -0.2530774915000200687, 0.9399606299212601712 ) ) ;
#14916=CARTESIAN_POINT ( 'NONE',  ( -0.4889536969035310210, -0.06441834428467370366, -1.569881889763779625 ) ) ;
#14918=CARTESIAN_POINT ( 'NONE',  ( -0.05926487674658171417, -0.4498374011143209117, -1.934055118110236338 ) ) ;
#14931=CARTESIAN_POINT ( 'NONE',  ( -0.4219236230595549419, 0.1431838228107190636, -1.934055118110236116 ) ) ;
#14934=CARTESIAN_POINT ( 'NONE',  ( 0.2669480828848183052, -0.2341512108694381034, 1.953740157480315043 ) ) ;
#14942=CARTESIAN_POINT ( 'NONE',  ( -0.1867299569291481776, 0.3233561589688985771, -3.115157480314960647 ) ) ;
#14949=CARTESIAN_POINT ( 'NONE',  ( -0.3642352168757148068, 0.4152525734086684461, 0.9202755905511811330 ) ) ;
#14956=CARTESIAN_POINT ( 'NONE',  ( -0.5118110236220472231, 0.03349795313264340019, 1.766732283464566899 ) ) ;
#14958=VERTEX_POINT ( 'NONE', #15440 ) ;
#14961=CARTESIAN_POINT ( 'NONE',  ( 0.1151913129404385921, 0.3392387706403768299, -3.115157480314960647 ) ) ;
#14966=CARTESIAN_POINT ( 'NONE',  ( 0.3346456692913385988, -0.02190250779246876237, 1.973425196850393970 ) ) ;
#14970=CARTESIAN_POINT ( 'NONE',  ( 0.4763861460130704994, -0.1275996891957771051, -1.550196850393700920 ) ) ;
#14989=CARTESIAN_POINT ( 'NONE',  ( -0.5314960629921260393, 6.402768735150616610E-17, 1.747047244094488194 ) ) ;
#14991=CYLINDRICAL_SURFACE ( 'NONE', #25219, 0.3346456692913385988 ) ;
#14993=CARTESIAN_POINT ( 'NONE',  ( 0.01288382760289561585, 0.2165354330708661457, -3.174212598425197207 ) ) ;
#15018=CARTESIAN_POINT ( 'NONE',  ( 0.5230301363771271417, 0.1775991818008589573, 0.9399606299212598381 ) ) ;
#15021=DIRECTION ( 'NONE',  ( 0.000000000000000000, 0.000000000000000000, 1.000000000000000000 ) ) ;
#15023=B_SPLINE_SURFACE_WITH_KNOTS ( 'NONE', 2, 3, ( 
 ( #26074, #13351, #21975, #22243, #15368, #15628, #784, #9371, #17976, #26612, #15887, #24490, #13766, #11644, #23959, #14056, #18550, #20687, #16588, #20822, #27330, #22812, #25061, #5728, #7846, #14342, #9666, #3159, #24630, #18263, #1341, #16317, #3433, #22956, #12070, #23098, #27053, #14492, #7981, #1070, #16450, #18110, #3572, #9946, #12350, #3727, #5579, #20970, #24920, #27196, #12207, #1473, #10085, #11786, #14205, #18693, #20405, #26902, #25201, #5868, #3294, #9510, #22668, #26759, #7409, #16032 ),
 ( #11934, #7552, #5288, #16179, #20552, #13913, #22531, #24779, #7704, #5443, #1207, #9807, #18407, #17153, #18831, #15052, #4158, #21531, #14784, #23389, #13047, #23525, #16727, #12631, #25340, #4440, #12768, #8668, #6283, #10503, #6559, #21393, #15183, #12495, #17287, #23797, #1613, #8532, #23666, #17020, #19408, #2032, #23244, #25769, #4299, #101, #6005, #25628, #21109, #27473, #14918, #14642, #25910, #10644, #10217, #8121, #8399, #6418, #1751, #3876, #10364, #27759, #19264, #18983, #21508, #12903 ),
 ( #2173, #1892, #19121, #27614, #16885, #8256, #10789, #25492, #6157, #4020, #21253, #5101, #15849, #13173, #9071, #6695, #4831, #6973, #24450, #13587, #15336, #17419, #4973, #26571, #19692, #22208, #26178, #8938, #17684, #21947, #13447, #10927, #7230, #21804, #22070, #19954, #21669, #2441, #17567, #2701, #2299, #11068, #15720, #23931, #26436, #4566, #26042, #2836, #606, #6831, #15596, #15461, #11336, #9200, #743, #11472, #20089, #24196, #17819, #7103, #24324, #9333, #361, #24057, #8804, #4692 ) ),
 .UNSPECIFIED., .F., .T., .F.,
 ( 3, 3 ),
 ( 4, 2, 2, 2, 2, 2, 2, 2, 2, 2, 2, 2, 2, 2, 2, 2, 2, 2, 2, 2, 2, 2, 2, 2, 2, 2, 2, 2, 2, 2, 2, 2, 4 ),
 ( 0.000000000000000000, 1.000000000000000000 ),
 ( 0.000000000000000000, 0.1963495408493620697, 0.3926990816987241395, 0.5890486225480862092, 0.7853981633974482790, 0.9817477042468103487, 1.178097245096172418, 1.374446785945534488, 1.570796326794896558, 1.767145867644258628, 1.963495408493620697, 2.159844949342982545, 2.356194490192344837, 2.552544031041707129, 2.748893571891068976, 2.945243112740430824, 3.141592653589793116, 3.337942194439155408, 3.534291735288517255, 3.730641276137879103, 3.926990816987241395, 4.123340357836603687, 4.319689898685965090, 4.516039439535327382, 4.712388980384689674, 4.908738521234051966, 5.105088062083414258, 5.301437602932775661, 5.497787143782137953, 5.694136684631500245, 5.890486225480861648, 6.086835766330223940, 6.283185307179586232 ),
 .UNSPECIFIED. ) ;
#15029=CARTESIAN_POINT ( 'NONE',  ( -0.4441657790094368230, 0.2564944395535841970, -1.550196850393700920 ) ) ;
#15030=CARTESIAN_POINT ( 'NONE',  ( -0.5672055940112499250, -0.07462095020172467008, 0.9399606299212600602 ) ) ;
#15033=CARTESIAN_POINT ( 'NONE',  ( -0.5280904602948607307, -0.06947618719658474329, 1.747047244094487972 ) ) ;
#15049=CARTESIAN_POINT ( 'NONE',  ( -0.1585706980422388890, 0.4669911931914605963, -1.550196850393700920 ) ) ;
#15052=CARTESIAN_POINT ( 'NONE',  ( -0.05926487674658593302, 0.4498374011143062567, -1.934055118110236338 ) ) ;
#15067=CARTESIAN_POINT ( 'NONE',  ( 0.4219262446671240840, 0.1431849087161535528, -1.934055118110236560 ) ) ;
#15069=VERTEX_POINT ( 'NONE', #1145 ) ;
#15076=CARTESIAN_POINT ( 'NONE',  ( 0.3726024258163779246, 0.02438677169350801990, -3.115157480314960647 ) ) ;
#15093=CARTESIAN_POINT ( 'NONE',  ( -0.1327036767659643679, -0.4954415918530851726, 1.766732283464566899 ) ) ;
#15098=CARTESIAN_POINT ( 'NONE',  ( -0.1151913129404409791, -0.3392387706403589553, -3.115157480314960647 ) ) ;
#15105=CARTESIAN_POINT ( 'NONE',  ( -0.02190250779245987017, -0.3346456692913387099, 1.973425196850393970 ) ) ;
#15117=CARTESIAN_POINT ( 'NONE',  ( -0.09334068553655658351, 0.3008231328410254091, -3.580124219708414657 ) ) ;
#15119=FACE_OUTER_BOUND ( 'NONE', #4896, .T. ) ;
#15129=AXIS2_PLACEMENT_3D ( 'NONE', #4770, #2371, #11004 ) ;
#15139=CARTESIAN_POINT ( 'NONE',  ( 0.2762247810519017355, -0.4783323773986510319, 0.9202755905511811330 ) ) ;
#15149=ADVANCED_FACE ( 'NONE', ( #20767, #10026 ), #16520, .T. ) ;
#15151=CARTESIAN_POINT ( 'NONE',  ( -0.09842519685039370636, 0.2165354330708661457, -3.272637795275590733 ) ) ;
#15154=CYLINDRICAL_SURFACE ( 'NONE', #17072, 0.3937007874015748254 ) ;
#15158=CARTESIAN_POINT ( 'NONE',  ( 0.4539000224941339701, 0.3482225189666781073, 0.9399606299212598381 ) ) ;
#15162=CIRCLE ( 'NONE', #2486, 0.3149606299212598381 ) ;
#15167=CARTESIAN_POINT ( 'NONE',  ( 0.4441657790094327707, -0.2564944395535760369, -1.550196850393700920 ) ) ;
#15182=CARTESIAN_POINT ( 'NONE',  ( -0.3707612262532960501, 0.3252100150720461658, -1.550196850393700920 ) ) ;
#15183=CARTESIAN_POINT ( 'NONE',  ( 0.4527559054764770385, 0.02963280468032115228, -1.934055118110236338 ) ) ;
#15189=CARTESIAN_POINT ( 'NONE',  ( 0.2355331214654088623, -0.4777261797697378021, 1.747047244094488194 ) ) ;
#15194=CARTESIAN_POINT ( 'NONE',  ( -0.3520598332081320558, -0.04632226222358686724, 1.953740157480314821 ) ) ;
#15201=CARTESIAN_POINT ( 'NONE',  ( -0.2761764805255799704, 0.3599896729929456529, -1.934055118110236338 ) ) ;
#15211=CARTESIAN_POINT ( 'NONE',  ( 0.1200583359873109851, -0.3535721684717733071, -3.115157480314960647 ) ) ;
#15225=CARTESIAN_POINT ( 'NONE',  ( -0.3855916753051397139, 0.3382184156732160329, 1.766732283464566899 ) ) ;
#15231=CARTESIAN_POINT ( 'NONE',  ( -0.2962590301041646557, 0.2272836761397697136, -3.115157480314960647 ) ) ;
#15232=ORIENTED_EDGE ( 'NONE', *, *, #11220, .F. ) ;
#15238=CARTESIAN_POINT ( 'NONE',  ( 0.2660793235464290474, -0.2041304421298306693, 1.953740157480315043 ) ) ;
#15260=CARTESIAN_POINT ( 'NONE',  ( -0.3666644560843326239, 0.2817828961649161412, -1.928289503579156960 ) ) ;
#15265=CARTESIAN_POINT ( 'NONE',  ( 0.09842519685039360922, 0.1968503937007873850, -3.272637795275590733 ) ) ;
#15269=DIRECTION ( 'NONE',  ( 0.000000000000000000, 0.000000000000000000, -1.000000000000000000 ) ) ;
#15274=DIRECTION ( 'NONE',  ( 0.7071067818211432821, 0.000000000000000000, 0.7071067805519516414 ) ) ;
#15278=CARTESIAN_POINT ( 'NONE',  ( -0.2762247810519398716, 0.4783323773986303262, 0.9399606299212598381 ) ) ;
#15301=CARTESIAN_POINT ( 'NONE',  ( -0.1480156394741835579, -0.5526079293737254927, 0.9399606299212598381 ) ) ;
#15302=VECTOR ( 'NONE', #22905, 39.37007874015748143 ) ;
#15308=ORIENTED_EDGE ( 'NONE', *, *, #21159, .T. ) ;
#15315=CARTESIAN_POINT ( 'NONE',  ( 0.4538399017589948015, -0.3483099419450786383, 0.9399606299212598381 ) ) ;
#15332=CARTESIAN_POINT ( 'NONE',  ( 0.03189995399141003218, 0.3133994105366679772, -3.641567849138989121 ) ) ;
#15334=CARTESIAN_POINT ( 'NONE',  ( 0.3707612262533330205, 0.3252100150720381722, -1.550196850393700920 ) ) ;
#15336=CARTESIAN_POINT ( 'NONE',  ( 0.1477428134820460426, 0.4351030398461616100, -1.928289503579165842 ) ) ;
#15343=CARTESIAN_POINT ( 'NONE',  ( -0.07874015748031502893, 0.1968503937007874127, -3.272637795275590733 ) ) ;
#15354=CARTESIAN_POINT ( 'NONE',  ( -0.2006393256663633884, 0.4069519308876736741, -1.934055118110236338 ) ) ;
#15360=CARTESIAN_POINT ( 'NONE',  ( -0.2712695779734264900, -0.3534635626045726786, -1.934055118110236116 ) ) ;
#15361=CARTESIAN_POINT ( 'NONE',  ( 0.3702005978258584573, 0.04877294052296160531, -3.115157480314960647 ) ) ;
#15368=CARTESIAN_POINT ( 'NONE',  ( -0.4218945342797432163, 0.1432577568504689591, -1.934055118110236338 ) ) ;
#15372=ADVANCED_FACE ( 'NONE', ( #17885 ), #5143, .T. ) ;
#15380=VERTEX_POINT ( 'NONE', #4912 ) ;
#15381=CARTESIAN_POINT ( 'NONE',  ( -0.2272836761397795113, -0.2962590301041581053, -3.115157480314960647 ) ) ;
#15386=CARTESIAN_POINT ( 'NONE',  ( -0.2904160862623610950, -0.1677079028045287690, 1.953740157480315043 ) ) ;
#15387=ORIENTED_EDGE ( 'NONE', *, *, #871, .T. ) ;
#15410=CARTESIAN_POINT ( 'NONE',  ( -0.09842519685039373412, 0.1968503937007873850, -3.272637795275590733 ) ) ;
#15414=CARTESIAN_POINT ( 'NONE',  ( 0.2669897767697305135, -0.2341075107470857453, 1.953740157480315043 ) ) ;
#15422=CARTESIAN_POINT ( 'NONE',  ( -0.2442565704126265502, 0.4954197419817717996, 0.9399606299212598381 ) ) ;
#15428=EDGE_CURVE ( 'NONE', #25987, #10805, #3363, .T. ) ;
#15436=CARTESIAN_POINT ( 'NONE',  ( -0.07472527936312116370, 0.5671862884094760471, 0.9399606299212598381 ) ) ;
#15440=CARTESIAN_POINT ( 'NONE',  ( -0.3574975638436101444, 0.000000000000000000, -3.115157480314960647 ) ) ;
#15458=CARTESIAN_POINT ( 'NONE',  ( 0.4669911931914377257, 0.1585706980422264545, -1.550196850393700920 ) ) ;
#15461=CARTESIAN_POINT ( 'NONE',  ( -0.1188866373884864824, -0.4438564651657386229, -1.928289503579162067 ) ) ;
#15486=CARTESIAN_POINT ( 'NONE',  ( -2.685748425196850164E-17, 0.000000000000000000, -3.745078740157480546 ) ) ;
#15487=CARTESIAN_POINT ( 'NONE',  ( 0.1213180142433833847, 0.3572819248074460829, -3.100567304031761395 ) ) ;
#15494=B_SPLINE_CURVE_WITH_KNOTS ( 'NONE', 2,
 ( #11300, #26004, #704 ),
 .UNSPECIFIED., .F., .F.,
 ( 3, 3 ),
 ( 0.000000000000000000, 1.000000000000000000 ),
 .UNSPECIFIED. ) ;
#15500=CARTESIAN_POINT ( 'NONE',  ( -0.06699590632655402778, 0.5118110236220472231, 1.766732283464566899 ) ) ;
#15502=CARTESIAN_POINT ( 'NONE',  ( 0.2268096725222696064, 0.4600326175561003650, 1.747047244094488194 ) ) ;
#15507=CARTESIAN_POINT ( 'NONE',  ( -0.1651192144506243575, -0.3349073414798197645, -3.115157480314960647 ) ) ;
#15513=CARTESIAN_POINT ( 'NONE',  ( 0.2211428102655656758, 0.2521176338356670432, 1.953740157480315043 ) ) ;
#15521=CARTESIAN_POINT ( 'NONE',  ( 0.07874015748031495954, 0.1968503937007874127, -3.548228346456692162 ) ) ;
#15535=CARTESIAN_POINT ( 'NONE',  ( -0.06699507805369007973, 0.5085118447801436625, 1.766732283464566899 ) ) ;
#15541=CARTESIAN_POINT ( 'NONE',  ( 0.1775236553383016391, -0.3075341118175515809, 1.953740157480314821 ) ) ;
#15548=VECTOR ( 'NONE', #25045, 39.37007874015748143 ) ;
#15550=CARTESIAN_POINT ( 'NONE',  ( 0.4152525734086270348, -0.3642352168757560515, 0.9202755905511811330 ) ) ;
#15554=ORIENTED_EDGE ( 'NONE', *, *, #7763, .F. ) ;
#15567=CARTESIAN_POINT ( 'NONE',  ( 0.03736310157557471562, -0.5708661417322835607, 0.9399606299212598381 ) ) ;
#15568=CARTESIAN_POINT ( 'NONE',  ( 0.5118110236220471121, -0.06699590632655400002, 1.766732283464566899 ) ) ;
#15584=CIRCLE ( 'NONE', #25518, 0.5511811023622047445 ) ;
#15593=CARTESIAN_POINT ( 'NONE',  ( 0.4763861460130703329, 0.1275996891957705826, -1.550196850393700920 ) ) ;
#15596=CARTESIAN_POINT ( 'NONE',  ( -0.06001958459474839719, -0.4555658499976154574, -1.928289503579151187 ) ) ;
#15597=CARTESIAN_POINT ( 'NONE',  ( 0.2564158049324918864, -0.4442166144912022552, -1.550196850393701142 ) ) ;
#15604=SURFACE_STYLE_USAGE ( .BOTH. , #9785 ) ;
#15606=EDGE_CURVE ( 'NONE', #19599, #22130, #26024, .T. ) ;
#15616=CARTESIAN_POINT ( 'NONE',  ( -0.3535065162672666461, -0.2712027394948650083, -1.934055118110236338 ) ) ;
#15622=CARTESIAN_POINT ( 'NONE',  ( 0.3740848232703748444, 0.04928467685643974500, -3.100567304031760507 ) ) ;
#15628=CARTESIAN_POINT ( 'NONE',  ( -0.3996230174612752095, 0.1970259548082017587, -1.934055118110236338 ) ) ;
#15632=CARTESIAN_POINT ( 'NONE',  ( -0.2577577458591218673, 0.4472135058506043759, 1.766732283464566899 ) ) ;
#15633=CARTESIAN_POINT ( 'NONE',  ( -0.2564944395516098874, 0.4441657790107518822, 1.747047244094488194 ) ) ;
#15638=CARTESIAN_POINT ( 'NONE',  ( 0.1651192144506298254, 0.3349073414798210413, -3.115157480314960647 ) ) ;
#15644=CARTESIAN_POINT ( 'NONE',  ( -0.2041304421298503480, 0.2660793235464394280, 1.953740157480315043 ) ) ;
#15649=CARTESIAN_POINT ( 'NONE',  ( 0.4446020952038907681, 5.549066237130534971E-17, -1.934055118110236338 ) ) ;
#15657=CARTESIAN_POINT ( 'NONE',  ( 0.000000000000000000, 0.000000000000000000, 1.953740157480315043 ) ) ;
#15658=CARTESIAN_POINT ( 'NONE',  ( 0.2817310484609195642, 0.2161381151962948888, 1.953740157480315043 ) ) ;
#15664=CARTESIAN_POINT ( 'NONE',  ( 0.3149606299212598381, 0.000000000000000000, -3.666338582670846780 ) ) ;
#15677=CARTESIAN_POINT ( 'NONE',  ( 0.5511811023622048555, 0.03607471876262481614, 0.9399606299212598381 ) ) ;
#15687=CARTESIAN_POINT ( 'NONE',  ( -0.3346456692913385988, 0.02190250779246044610, 1.953740157480315043 ) ) ;
#15691=EDGE_CURVE ( 'NONE', #7980, #27336, #13553, .T. ) ;
#15693=CARTESIAN_POINT ( 'NONE',  ( 0.07472527936311225416, 0.5671862884095085766, 0.9399606299212598381 ) ) ;
#15694=CARTESIAN_POINT ( 'NONE',  ( -0.06699590632655402778, -0.5118110236220471121, 1.766732283464566899 ) ) ;
#15711=AXIS2_PLACEMENT_3D ( 'NONE', #6830, #11333, #8936 ) ;
#15714=CARTESIAN_POINT ( 'NONE',  ( -0.07870736637777375755, 0.2165354330708661457, -3.608715228343988279 ) ) ;
#15720=CARTESIAN_POINT ( 'NONE',  ( 0.2796934465393767222, -0.3645739570812915331, -1.928289503579138753 ) ) ;
#15726=ADVANCED_BREP_SHAPE_REPRESENTATION ( 'Cam Shaft', ( #12711, #11588 ), #2999 ) ;
#15742=CARTESIAN_POINT ( 'NONE',  ( 0.3543307086614174151, 0.02327295973586337649, 1.953740157480314821 ) ) ;
#15745=CARTESIAN_POINT ( 'NONE',  ( 0.4498374011143674855, 0.05926487674658936083, -1.934055118110236338 ) ) ;
#15753=CARTESIAN_POINT ( 'NONE',  ( 0.2296683860596781812, -0.2993674444872274631, -3.100567304031764060 ) ) ;
#15767=CARTESIAN_POINT ( 'NONE',  ( 0.2564944395515434961, -0.4441657790107952364, 1.766732283464566899 ) ) ;
#15770=CARTESIAN_POINT ( 'NONE',  ( -0.3702005978258584573, -0.04877294052295926691, -3.115157480314960647 ) ) ;
#15775=CARTESIAN_POINT ( 'NONE',  ( 0.2521176338356516666, -0.2211428102655709216, 1.953740157480315043 ) ) ;
#15785=DIRECTION ( 'NONE',  ( 0.000000000000000000, 0.000000000000000000, -1.000000000000000000 ) ) ;
#15790=CARTESIAN_POINT ( 'NONE',  ( 0.2817310484609266696, -0.2161381151962942504, 1.953740157480315043 ) ) ;
#15795=CARTESIAN_POINT ( 'NONE',  ( -0.3765118517642104257, 2.305470170520414967E-17, -3.100567304031763172 ) ) ;
#15796=CARTESIAN_POINT ( 'NONE',  ( 0.5085118447801502128, -0.06699507805371243685, 1.747047244094488194 ) ) ;
#15802=ORIENTED_EDGE ( 'NONE', *, *, #9003, .F. ) ;
#15805=CARTESIAN_POINT ( 'NONE',  ( 0.03220957031753989008, 0.4921259842519685179, -1.569881889763779625 ) ) ;
#15808=CARTESIAN_POINT ( 'NONE',  ( 0.5526079293737398146, 0.1480156394741914405, 0.9399606299212598381 ) ) ;
#15833=CARTESIAN_POINT ( 'NONE',  ( -0.07669076177803985095, 0.1968503937007873850, -3.568838416488017362 ) ) ;
#15837=EDGE_CURVE ( 'NONE', #10141, #25275, #11233, .T. ) ;
#15841=CARTESIAN_POINT ( 'NONE',  ( -0.5118110236220473341, 0.000000000000000000, -1.550196850393700920 ) ) ;
#15847=CARTESIAN_POINT ( 'NONE',  ( 0.1677079028045456166, 0.2904160862623617056, 1.973425196850393970 ) ) ;
#15848=CARTESIAN_POINT ( 'NONE',  ( 0.03349795313024148125, 0.5118110236220473341, -1.550196850393700920 ) ) ;
#15849=CARTESIAN_POINT ( 'NONE',  ( -0.2031943647053863211, 0.4121342552748505916, -1.928289503579144748 ) ) ;
#15853=CARTESIAN_POINT ( 'NONE',  ( 0.3001918266902277588, 0.3912931228432131592, -1.569881889763779625 ) ) ;
#15858=( NAMED_UNIT ( * ) PLANE_ANGLE_UNIT ( ) SI_UNIT ( $, .RADIAN. ) ) ;
#15866=CARTESIAN_POINT ( 'NONE',  ( 0.3362580771780208644, 0.1141156591735774661, 1.953740157480315043 ) ) ;
#15869=CARTESIAN_POINT ( 'NONE',  ( -0.05926487674658171417, -0.4498374011143209117, -1.934055118110236338 ) ) ;
#15872=CARTESIAN_POINT ( 'NONE',  ( 0.09777739100673171757, 0.2994019835985785583, -3.259649345945281329 ) ) ;
#15875=ORIENTED_EDGE ( 'NONE', *, *, #8806, .T. ) ;
#15883=CARTESIAN_POINT ( 'NONE',  ( 0.1668516812751341394, -0.3384212623783144913, -3.100567304031760951 ) ) ;
#15887=CARTESIAN_POINT ( 'NONE',  ( -0.2712027394948746117, 0.3535065162672773043, -1.934055118110236338 ) ) ;
#15895=CARTESIAN_POINT ( 'NONE',  ( -0.4441657790107816917, 0.2564944395515652564, 1.747047244094488194 ) ) ;
#15899=CARTESIAN_POINT ( 'NONE',  ( -0.2993674444872340690, 0.2296683860596682170, -3.100567304031764060 ) ) ;
#15913=CARTESIAN_POINT ( 'NONE',  ( -0.02063524494269025969, 0.1968503937007874127, -3.624905640648360183 ) ) ;
#15916=CARTESIAN_POINT ( 'NONE',  ( 0.04840761057748826229, 0.1968503937007874127, -3.209693978926679847 ) ) ;
#15922=CARTESIAN_POINT ( 'NONE',  ( 0.06048688188729473697, 0.2165354330708661734, -3.193930428897816753 ) ) ;
#15923=CARTESIAN_POINT ( 'NONE',  ( -0.2924088307484721816, -0.1685339107540411718, 1.973425196850393526 ) ) ;
#15924=CARTESIAN_POINT ( 'NONE',  ( -0.09187177619658792871, 0.3429980251342187314, 1.953740157480315043 ) ) ;
#15926=CARTESIAN_POINT ( 'NONE',  ( -0.09842519685039370636, 0.2991866959364303247, -3.272637795275590733 ) ) ;
#15931=CARTESIAN_POINT ( 'NONE',  ( 0.2564944395515637576, -0.4441657790108029524, 1.747047244094488194 ) ) ;
#15933=CARTESIAN_POINT ( 'NONE',  ( 0.4441657790107835790, 0.2564944395515610931, 1.766732283464566899 ) ) ;
#15942=CARTESIAN_POINT ( 'NONE',  ( -0.4423390553432505201, 0.2180862235769355506, -1.569881889763779625 ) ) ;
#15945=CARTESIAN_POINT ( 'NONE',  ( 0.1775991818008549328, -0.5230301363771188150, 0.9399606299212598381 ) ) ;
#15962=CARTESIAN_POINT ( 'NONE',  ( 0.2211428102655795813, -0.2521176338356631019, 1.953740157480315043 ) ) ;
#15980=CARTESIAN_POINT ( 'NONE',  ( -0.07874015748031511219, 0.1968503937007873850, -3.548228346456693050 ) ) ;
#15988=CARTESIAN_POINT ( 'NONE',  ( -0.09855118063547704810, 0.3667122560601320247, -3.100567304031763172 ) ) ;
#15994=CARTESIAN_POINT ( 'NONE',  ( 0.1482986320106399469, 0.3007905576423889893, 1.973425196850393970 ) ) ;
#15996=CARTESIAN_POINT ( 'NONE',  ( -0.4856708409191340392, 0.1649135259639384898, -1.550196850393700920 ) ) ;
#15997=CARTESIAN_POINT ( 'NONE',  ( -0.5511811023622047445, 3.375010863791918375E-17, 0.9202755905511811330 ) ) ;
#15999=CARTESIAN_POINT ( 'NONE',  ( -0.4783323773986509764, -0.2762247810519017355, 0.9202755905511811330 ) ) ;
#16010=EDGE_LOOP ( 'NONE', ( #24861, #20462, #1138, #330 ) ) ;
#16016=CARTESIAN_POINT ( 'NONE',  ( 0.2669917830071264486, 0.2341095169845867630, 1.953740157480315487 ) ) ;
#16018=CARTESIAN_POINT ( 'NONE',  ( 0.3929158813954875540, -0.2268989272875726881, -1.934055118110236338 ) ) ;
#16021=CARTESIAN_POINT ( 'NONE',  ( 0.02573923578592207315, 0.3139710921709522595, -3.177418918035737949 ) ) ;
#16026=CARTESIAN_POINT ( 'NONE',  ( -0.4219262446670208888, -0.1431849087164892009, -1.934055118110236116 ) ) ;
#16027=CARTESIAN_POINT ( 'NONE',  ( 0.3384212623783066642, -0.1668516812751465739, -3.100567304031770277 ) ) ;
#16032=CARTESIAN_POINT ( 'NONE',  ( -0.4446020952038907681, 0.000000000000000000, -1.934055118110236338 ) ) ;
#16035=CARTESIAN_POINT ( 'NONE',  ( -0.3454440660767502114, -0.3030032861725112103, -1.928289503579147635 ) ) ;
#16042=CARTESIAN_POINT ( 'NONE',  ( -0.5085118447801415531, -0.06699507805368200286, 1.747047244094488194 ) ) ;
#16047=CARTESIAN_POINT ( 'NONE',  ( 0.1668516812751446310, 0.3384212623783090512, -3.100567304031764948 ) ) ;
#16058=CARTESIAN_POINT ( 'NONE',  ( 0.05819755867304853003, -0.4417361510194242613, -1.934055118110236338 ) ) ;
#16064=CARTESIAN_POINT ( 'NONE',  ( 0.02063524494269815615, 0.1968503937007874127, -3.195960501083794814 ) ) ;
#16066=CARTESIAN_POINT ( 'NONE',  ( -0.1685339107540412551, 0.2924088307484719595, 1.973425196850393970 ) ) ;
#16067=DIRECTION ( 'NONE',  ( 0.000000000000000000, 0.000000000000000000, 1.000000000000000000 ) ) ;
#16071=CARTESIAN_POINT ( 'NONE',  ( -0.2817310484609168997, -0.2161381151963037983, 1.953740157480315043 ) ) ;
#16078=CARTESIAN_POINT ( 'NONE',  ( 0.1649135259617203753, -0.4856708409200670151, 1.747047244094488194 ) ) ;
#16088=CARTESIAN_POINT ( 'NONE',  ( -0.2816963220976719806, -0.2161875334156889150, 1.953740157480315043 ) ) ;
#16092=CARTESIAN_POINT ( 'NONE',  ( -0.4669911931914806358, 0.1585706980422473544, -1.569881889763779625 ) ) ;
#16094=CARTESIAN_POINT ( 'NONE',  ( -0.2529800193559212929, 0.5131133041954029084, 0.9399606299212598381 ) ) ;
#16096=CARTESIAN_POINT ( 'NONE',  ( -0.3346456692913385988, 2.134256245050205639E-17, 1.973425196850393970 ) ) ;
#16097=CARTESIAN_POINT ( 'NONE',  ( -0.09842519685039370636, 0.2991866959364303802, -3.548228346456693050 ) ) ;
#16120=ORIENTED_EDGE ( 'NONE', *, *, #23921, .T. ) ;
#16126=CARTESIAN_POINT ( 'NONE',  ( -0.09842519684999369300, 0.1968503937007873850, -3.561114497143084368 ) ) ;
#16127=ORIENTED_EDGE ( 'NONE', *, *, #23073, .F. ) ;
#16135=CARTESIAN_POINT ( 'NONE',  ( -0.1896185148830509259, 0.3289909311256231650, -3.100567304031763172 ) ) ;
#16141=CARTESIAN_POINT ( 'NONE',  ( 0.3346456692913385988, 0.000000000000000000, 1.973425196850393970 ) ) ;
#16142=CARTESIAN_POINT ( 'NONE',  ( -0.3855916753034290823, 0.3382184156749268311, -1.550196850393700920 ) ) ;
#16149=CARTESIAN_POINT ( 'NONE',  ( -0.1585706980422471879, 0.4669911931914806913, -1.569881889763779625 ) ) ;
#16163=CARTESIAN_POINT ( 'NONE',  ( -0.2341095169845849588, 0.2669917830071098508, 1.953740157480314821 ) ) ;
#16176=CARTESIAN_POINT ( 'NONE',  ( -0.2488091035917020799, -0.2836590635674518524, -3.100567304031764948 ) ) ;
#16179=CARTESIAN_POINT ( 'NONE',  ( -0.4382752542996525835, 0.1173917140416343985, -1.934055118110236338 ) ) ;
#16186=CARTESIAN_POINT ( 'NONE',  ( 0.2268096725222282783, -0.4600326175560538466, 1.747047244094488194 ) ) ;
#16188=VERTEX_POINT ( 'NONE', #19535 ) ;
#16190=CARTESIAN_POINT ( 'NONE',  ( 0.3572819248074444731, 0.1213180142433879782, -3.100567304031760951 ) ) ;
#16195=CARTESIAN_POINT ( 'NONE',  ( -0.1648264847745520012, 0.4857053587578358256, -1.550196850393700920 ) ) ;
#16207=VECTOR ( 'NONE', #17278, 39.37007874015748143 ) ;
#16211=CARTESIAN_POINT ( 'NONE',  ( -0.3184841198566448206, 0.1570220809524502381, 1.953740157480315043 ) ) ;
#16217=VECTOR ( 'NONE', #8017, 39.37007874015748143 ) ;
#16220=AXIS2_PLACEMENT_3D ( 'NONE', #12106, #3912, #10404 ) ;
#16222=CARTESIAN_POINT ( 'NONE',  ( -0.1712563538833084820, -0.5043504886477717664, 1.747047244094488194 ) ) ;
#16223=CARTESIAN_POINT ( 'NONE',  ( 0.2268096725222696064, 0.4600326175561003650, 1.747047244094488194 ) ) ;
#16235=CARTESIAN_POINT ( 'NONE',  ( -0.4763861460130343062, -0.1275996891957688339, -1.569881889763779625 ) ) ;
#16250=CARTESIAN_POINT ( 'NONE',  ( 0.3346456692913385988, -0.02190250779246876237, 1.953740157480315043 ) ) ;
#16277=CARTESIAN_POINT ( 'NONE',  ( 0.3239425792934412240, 0.08676778863010829734, 1.973425196850393970 ) ) ;
#16282=CARTESIAN_POINT ( 'NONE',  ( 0.5476281405333177643, 0.07214854559198216610, 0.9202755905511811330 ) ) ;
#16287=CARTESIAN_POINT ( 'NONE',  ( 0.4669911931914765835, 0.1585706980422571244, -1.569881889763779625 ) ) ;
#16290=CARTESIAN_POINT ( 'NONE',  ( 0.5043892184459985994, 0.1711665596932881450, 1.747047244094488194 ) ) ;
#16296=FACE_OUTER_BOUND ( 'NONE', #25895, .T. ) ;
#16309=EDGE_LOOP ( 'NONE', ( #16851, #8525, #3703, #1766 ) ) ;
#16311=CARTESIAN_POINT ( 'NONE',  ( 0.4585215200179055817, -2.840735999735804609E-17, -1.928289503579156516 ) ) ;
#16315=CARTESIAN_POINT ( 'NONE',  ( 0.3912931228432222075, -0.3001918266902142696, -1.569881889763779625 ) ) ;
#16317=CARTESIAN_POINT ( 'NONE',  ( 0.4417361510194462992, 0.05819755867304002989, -1.934055118110236338 ) ) ;
#16325=CARTESIAN_POINT ( 'NONE',  ( 0.3855916753051596424, -0.3382184156732262470, 1.747047244094488194 ) ) ;
#16328=CARTESIAN_POINT ( 'NONE',  ( -0.2296683860596777926, -0.2993674444872276297, -3.100567304031764060 ) ) ;
#16341=EDGE_CURVE ( 'NONE', #4928, #22130, #18268, .T. ) ;
#16345=CARTESIAN_POINT ( 'NONE',  ( 0.3392387706403788838, 0.1151913129404419922, -3.115157480314960647 ) ) ;
#16347=CARTESIAN_POINT ( 'NONE',  ( 0.2056553984168021654, 0.2676050456844303316, 1.973425196850393526 ) ) ;
#16359=CARTESIAN_POINT ( 'NONE',  ( -0.3242071728275120468, 0.4225965726692976765, 1.747047244094488194 ) ) ;
#16360=CARTESIAN_POINT ( 'NONE',  ( 0.4856708409200641841, -0.1649135259617057481, 1.766732283464566899 ) ) ;
#16364=CARTESIAN_POINT ( 'NONE',  ( -0.1151913129404333325, 0.3392387706403566239, -3.115157480314960647 ) ) ;
#16371=CARTESIAN_POINT ( 'NONE',  ( 0.4889536969035315761, -0.06441834428467053952, -1.569881889763779625 ) ) ;
#16386=CARTESIAN_POINT ( 'NONE',  ( -0.2478439864030017592, 0.4300129863948120579, -1.569881889763779625 ) ) ;
#16392=AXIS2_PLACEMENT_3D ( 'NONE', #27666, #18751, #16932 ) ;
#16399=CARTESIAN_POINT ( 'NONE',  ( 0.07669076177803835215, 0.1968503937007873850, -3.568838416488088860 ) ) ;
#16400=ORIENTED_EDGE ( 'NONE', *, *, #19037, .T. ) ;
#16401=DIRECTION ( 'NONE',  ( 1.000000000000000000, 0.000000000000000000, 0.000000000000000000 ) ) ;
#16408=CARTESIAN_POINT ( 'NONE',  ( -0.4069448477569433953, -0.3121994997578269593, -1.550196850393700920 ) ) ;
#16412=CARTESIAN_POINT ( 'NONE',  ( -0.07214854559198564943, -0.5476281405333169872, 0.9202755905511811330 ) ) ;
#16419=CARTESIAN_POINT ( 'NONE',  ( 0.4889536969035315761, -0.06441834428467053952, -1.569881889763779625 ) ) ;
#16428=LINE ( 'NONE', #12327, #15548 ) ;
#16442=EDGE_CURVE ( 'NONE', #804, #15069, #16706, .T. ) ;
#16446=CARTESIAN_POINT ( 'NONE',  ( -0.2842139414039350775, -0.2181198385717931787, -3.115157480314961091 ) ) ;
#16450=CARTESIAN_POINT ( 'NONE',  ( 0.3349573549949902418, -0.2938049579018460755, -1.934055118110236338 ) ) ;
#16458=CARTESIAN_POINT ( 'NONE',  ( 0.3121994997598398491, -0.4069448477555819843, 1.747047244094488194 ) ) ;
#16462=CARTESIAN_POINT ( 'NONE',  ( -0.2296683860596825943, 0.2993674444872254092, -3.100567304031761395 ) ) ;
#16463=CARTESIAN_POINT ( 'NONE',  ( -0.09842519685039370636, 0.2165354330708661457, -3.272637795275590733 ) ) ;
#16475=EDGE_CURVE ( 'NONE', #285, #16188, #20306, .T. ) ;
#16476=CARTESIAN_POINT ( 'NONE',  ( -0.1151913129404409791, -0.3392387706403589553, -3.115157480314960647 ) ) ;
#16479=CARTESIAN_POINT ( 'NONE',  ( -0.2676050456844304981, 0.2056553984168023042, 1.973425196850394858 ) ) ;
#16490=CARTESIAN_POINT ( 'NONE',  ( 0.09586345242798374744, 0.2165354330708660902, -3.573990933499927802 ) ) ;
#16494=DIRECTION ( 'NONE',  ( -1.000000000000000000, 0.000000000000000000, 0.000000000000000000 ) ) ;
#16502=CARTESIAN_POINT ( 'NONE',  ( 0.4921259842519685179, 0.03220957031754003580, -1.550196850393700920 ) ) ;
#16520=PLANE ( 'NONE',  #2452 ) ;
#16547=CARTESIAN_POINT ( 'NONE',  ( -0.5230301363771188150, -0.1775991818008711975, 0.9399606299212598381 ) ) ;
#16557=CARTESIAN_POINT ( 'NONE',  ( 0.4004922687719589258, 0.3511586785140410893, 1.747047244094488416 ) ) ;
#16563=CARTESIAN_POINT ( 'NONE',  ( 0.000000000000000000, 0.000000000000000000, 2.504921259842519898 ) ) ;
#16583=CARTESIAN_POINT ( 'NONE',  ( -0.2693781226335786316, -0.2362017869179856566, -3.115157480314961980 ) ) ;
#16584=CARTESIAN_POINT ( 'NONE',  ( 0.3252100150720381722, -0.3707612262533039327, -1.569881889763779625 ) ) ;
#16585=EDGE_CURVE ( 'NONE', #21933, #18631, #19401, .T. ) ;
#16588=CARTESIAN_POINT ( 'NONE',  ( 0.05819755867303724045, 0.4417361510194101615, -1.934055118110236338 ) ) ;
#16596=CARTESIAN_POINT ( 'NONE',  ( 0.4777261797697469614, 0.2355331214654221850, 1.747047244094488194 ) ) ;
#16603=CARTESIAN_POINT ( 'NONE',  ( 0.04638120790932896698, -0.3520466617656974884, 1.953740157480315043 ) ) ;
#16607=CARTESIAN_POINT ( 'NONE',  ( -0.1896185148830506761, -0.3289909311256231095, -3.100567304031762728 ) ) ;
#16608=CARTESIAN_POINT ( 'NONE',  ( 0.5476281405333121022, -0.07214854559198019546, 0.9399606299212598381 ) ) ;
#16616=CARTESIAN_POINT ( 'NONE',  ( -0.2693339498142315880, 0.2362439534887433579, -3.115157480314960647 ) ) ;
#16634=CARTESIAN_POINT ( 'NONE',  ( 0.06048688188729493126, 0.2165354330708660902, -3.626935712834465697 ) ) ;
#16637=CARTESIAN_POINT ( 'NONE',  ( 0.2564944395515434961, -0.4441657790107952364, 1.766732283464566899 ) ) ;
#16643=CARTESIAN_POINT ( 'NONE',  ( -0.2693339498142315880, 0.2362439534887433579, -3.115157480314960647 ) ) ;
#16649=CARTESIAN_POINT ( 'NONE',  ( 0.3346456692913385988, 0.02190250779246873461, 1.953740157480315043 ) ) ;
#16652=CARTESIAN_POINT ( 'NONE',  ( -0.1585706980422225409, -0.4669911931914833558, -1.550196850393700920 ) ) ;
#16662=DIRECTION ( 'NONE',  ( 1.000000000000000000, 0.000000000000000000, 0.000000000000000000 ) ) ;
#16676=CARTESIAN_POINT ( 'NONE',  ( 0.5905511811023621549, 0.000000000000000000, 0.9399606299212598381 ) ) ;
#16687=CARTESIAN_POINT ( 'NONE',  ( -0.5476281405333199848, 0.07214854559197045325, 0.9202755905511811330 ) ) ;
#16690=VERTEX_POINT ( 'NONE', #16096 ) ;
#16699=CARTESIAN_POINT ( 'NONE',  ( 0.04380447413658629385, 0.3324885138898144854, 1.953740157480315043 ) ) ;
#16700=CARTESIAN_POINT ( 'NONE',  ( 0.03349795313024073878, -0.5118110236220473341, -1.550196850393700920 ) ) ;
#16703=CARTESIAN_POINT ( 'NONE',  ( -0.5335524835331961757, -0.1429116519061072454, 0.9399606299212598381 ) ) ;
#16706=CIRCLE ( 'NONE', #18955, 0.3135473077061334268 ) ;
#16709=CARTESIAN_POINT ( 'NONE',  ( -0.1649135259639237794, 0.4856708409191340947, -1.550196850393700920 ) ) ;
#16718=CARTESIAN_POINT ( 'NONE',  ( -2.685748425196850164E-17, 0.000000000000000000, -3.666338582670846780 ) ) ;
#16726=CARTESIAN_POINT ( 'NONE',  ( -0.02345921195929173697, -0.3574989824755908652, -3.115157480314960647 ) ) ;
#16727=CARTESIAN_POINT ( 'NONE',  ( 0.2268989272875726881, 0.3929158813954875540, -1.934055118110236338 ) ) ;
#16728=CARTESIAN_POINT ( 'NONE',  ( -0.4555658499976060760, 0.06001958459474820984, -1.928289503579160513 ) ) ;
#16729=ADVANCED_FACE ( 'NONE', ( #9431, #22444 ), #13830, .T. ) ;
#16732=EDGE_LOOP ( 'NONE', ( #11823, #6047, #21027, #19544 ) ) ;
#16736=CARTESIAN_POINT ( 'NONE',  ( -0.5144970376935739109, -0.1378076643338908835, 1.747047244094488194 ) ) ;
#16745=CARTESIAN_POINT ( 'NONE',  ( -0.4446020952038907681, 0.000000000000000000, -1.934055118110236338 ) ) ;
#16747=CARTESIAN_POINT ( 'NONE',  ( 0.3074993854542625304, -0.1775730735577552566, 1.953740157480315043 ) ) ;
#16752=CARTESIAN_POINT ( 'NONE',  ( -0.5335524835331961757, -0.1429116519061072454, 0.9399606299212598381 ) ) ;
#16760=CARTESIAN_POINT ( 'NONE',  ( 0.3102476824511484210, 0.1791601451668926315, -3.115157480314960647 ) ) ;
#16775=CARTESIAN_POINT ( 'NONE',  ( 0.1712563538833069832, -0.5043504886477723215, 1.747047244094488194 ) ) ;
#16778=CARTESIAN_POINT ( 'NONE',  ( 0.4441657790108421988, 0.2564944395515498798, 1.747047244094488194 ) ) ;
#16782=CARTESIAN_POINT ( 'NONE',  ( 0.04679574315772144777, 0.3551931031211610912, -3.115157480314960647 ) ) ;
#16788=CARTESIAN_POINT ( 'NONE',  ( -0.08676778863011327947, 0.3239425792934402248, 1.973425196850393970 ) ) ;
#16792=CARTESIAN_POINT ( 'NONE',  ( 0.3001918266902036669, -0.3912931228432058872, -1.550196850393700920 ) ) ;
#16817=PLANE ( 'NONE',  #13958 ) ;
#16829=DIRECTION ( 'NONE',  ( -0.000000000000000000, -0.000000000000000000, 1.000000000000000000 ) ) ;
#16838=ADVANCED_FACE ( 'NONE', ( #18719 ), #21661, .T. ) ;
#16839=DIRECTION ( 'NONE',  ( -1.000000000000000000, 0.000000000000000000, -0.000000000000000000 ) ) ;
#16843=CARTESIAN_POINT ( 'NONE',  ( 0.3324885138898234782, -0.04380447413659139394, 1.973425196850393970 ) ) ;
#16847=CARTESIAN_POINT ( 'NONE',  ( -0.07214854559199535000, -0.5476281405333250918, 0.9399606299212598381 ) ) ;
#16851=ORIENTED_EDGE ( 'NONE', *, *, #871, .F. ) ;
#16859=CARTESIAN_POINT ( 'NONE',  ( 0.4069448477569526101, -0.3121994997578271813, -1.550196850393700920 ) ) ;
#16860=CARTESIAN_POINT ( 'NONE',  ( -0.5708661417322835607, -0.03747632742162953362, 0.9399606299212600602 ) ) ;
#16863=CARTESIAN_POINT ( 'NONE',  ( 0.06947618719649770180, -0.5280904602948609528, 1.747047244094488416 ) ) ;
#16883=CARTESIAN_POINT ( 'NONE',  ( 0.4423390553432409722, -0.2180862235769587265, -1.569881889763779625 ) ) ;
#16885=CARTESIAN_POINT ( 'NONE',  ( -0.4351030398461734339, 0.1477428134820354677, -1.928289503579158959 ) ) ;
#16898=CARTESIAN_POINT ( 'NONE',  ( 0.02319089060378217229, -0.3543307086614173596, 1.953740157480315043 ) ) ;
#16902=CARTESIAN_POINT ( 'NONE',  ( -0.5526079293736928522, -0.1480156394741928838, 0.9399606299212598381 ) ) ;
#16906=CARTESIAN_POINT ( 'NONE',  ( -0.2842490391651530390, -0.2180698645301770988, -3.115157480314960647 ) ) ;
#16930=CARTESIAN_POINT ( 'NONE',  ( 0.2693339498142349187, -0.2362439534887297299, -3.115157480314960647 ) ) ;
#16932=DIRECTION ( 'NONE',  ( 1.000000000000000000, 0.000000000000000000, -0.000000000000000000 ) ) ;
#16935=CARTESIAN_POINT ( 'NONE',  ( -0.3239425792934405024, 0.08676778863011171128, 1.973425196850393970 ) ) ;
#16939=CARTESIAN_POINT ( 'NONE',  ( 0.4669911931914963454, -0.1585706980422251222, -1.550196850393700920 ) ) ;
#16944=DIRECTION ( 'NONE',  ( 1.000000000000000000, 0.000000000000000000, 0.000000000000000000 ) ) ;
#16953=CARTESIAN_POINT ( 'NONE',  ( -0.1200170377978882624, 0.4465874321618641951, -1.928289503579156960 ) ) ;
#16955=CARTESIAN_POINT ( 'NONE',  ( 0.3346456692913385988, 4.098227477461614641E-17, 2.504921259842519898 ) ) ;
#16957=CARTESIAN_POINT ( 'NONE',  ( 0.02061007003135907623, 0.1968503937007873850, -3.195947033497543721 ) ) ;
#16963=ORIENTED_EDGE ( 'NONE', *, *, #24423, .F. ) ;
#16967=CARTESIAN_POINT ( 'NONE',  ( 0.4783323773986568606, 0.2762247810518930202, 0.9202755905511811330 ) ) ;
#16977=B_SPLINE_CURVE_WITH_KNOTS ( 'NONE', 2,
 ( #17824, #12805, #2069 ),
 .UNSPECIFIED., .F., .F.,
 ( 3, 3 ),
 ( 0.000000000000000000, 1.000000000000000000 ),
 .UNSPECIFIED. ) ;
#16981=CARTESIAN_POINT ( 'NONE',  ( -0.09842519685039366473, 0.1968503937007873850, -3.364501312335960836 ) ) ;
#16986=CARTESIAN_POINT ( 'NONE',  ( 0.2442565704126269388, 0.4954197419817067960, 0.9399606299212598381 ) ) ;
#16989=CARTESIAN_POINT ( 'NONE',  ( 0.3213059197595201644, 0.1584813376848823729, -3.115157480314960647 ) ) ;
#16995=CARTESIAN_POINT ( 'NONE',  ( 0.1649135259639267770, -0.4856708409191258236, -1.550196850393700920 ) ) ;
#17002=ORIENTED_EDGE ( 'NONE', *, *, #18180, .T. ) ;
#17016=CARTESIAN_POINT ( 'NONE',  ( 0.1585706980422246781, 0.4669911931914895176, -1.550196850393700920 ) ) ;
#17020=CARTESIAN_POINT ( 'NONE',  ( 0.3599896729929412120, -0.2761764805255614297, -1.934055118110236338 ) ) ;
#17032=B_SPLINE_SURFACE_WITH_KNOTS ( 'NONE', 2, 3, ( 
 ( #25672, #271, #17059, #19166, #23964, #2339, #8, #17332, #17193, #4478, #6600, #2484, #4598, #19726, #8710, #10969, #19594, #21712, #8843, #23569, #396, #19308, #1937, #8974, #2209, #15225, #17466, #23838, #27803, #21298, #13088, #23432, #14956, #26080, #4065, #10545, #8438, #6326, #4202, #138, #12808, #21436, #2077, #10690, #25809, #6458, #15093, #23703, #4339, #12942, #21573, #3016, #11236, #13776, #15767, #1075, #3163, #7414, #13922, #9673, #9522, #18118, #11796, #9109, #11516, #22394 ),
 ( #26480, #19861, #18271, #17984, #22537, #20132, #24369, #20413, #7276, #26913, #20273, #792, #15502, #24100, #11654, #933, #2882, #5297, #26619, #17728, #4735, #26765, #15633, #5011, #9378, #7012, #13357, #15895, #517, #21982, #24498, #2615, #26350, #22251, #16042, #19996, #13630, #5149, #24638, #24236, #4875, #13489, #22116, #7144, #2745, #11377, #649, #9239, #17857, #24785, #18991, #22675, #7560, #16186, #7991, #16458, #12357, #16325, #14063, #12502, #22822, #14215, #1481, #5876, #20559, #25071 ),
 ( #10093, #20976, #18702, #11942, #5450, #16596, #3883, #27060, #14503, #3302, #1620, #27339, #10370, #21117, #3584, #1212, #22965, #25209, #23106, #3735, #10224, #18416, #14352, #7712, #27200, #23251, #18840, #5585, #27481, #7849, #1757, #3440, #8127, #6012, #12077, #16736, #25349, #20696, #14649, #18556, #5735, #12217, #13182, #10798, #6567, #2448, #17429, #25501, #4028, #27764, #6166, #6291, #25776, #15189, #21263, #19556, #21679, #4167, #2307, #12774, #26045, #10507, #21400, #2040, #10653, #19273 ) ),
 .UNSPECIFIED., .F., .T., .F.,
 ( 3, 3 ),
 ( 4, 2, 2, 2, 2, 2, 2, 2, 2, 2, 2, 2, 2, 2, 2, 2, 2, 2, 2, 2, 2, 2, 2, 2, 2, 2, 2, 2, 2, 2, 2, 2, 4 ),
 ( 0.000000000000000000, 1.000000000000000000 ),
 ( 0.000000000000000000, 0.1963495408493620697, 0.3926990816987241395, 0.5890486225480862092, 0.7853981633974482790, 0.9817477042468103487, 1.178097245096172418, 1.374446785945534488, 1.570796326794896558, 1.767145867644258628, 1.963495408493620697, 2.159844949342982545, 2.356194490192344837, 2.552544031041707129, 2.748893571891068976, 2.945243112740430824, 3.141592653589793116, 3.337942194439155408, 3.534291735288517255, 3.730641276137879103, 3.926990816987241395, 4.123340357836603687, 4.319689898685965090, 4.516039439535327382, 4.712388980384689674, 4.908738521234051966, 5.105088062083414258, 5.301437602932775661, 5.497787143782137953, 5.694136684631500245, 5.890486225480861648, 6.086835766330223940, 6.283185307179586232 ),
 .UNSPECIFIED. ) ;
#17035=CARTESIAN_POINT ( 'NONE',  ( -0.02319089060378155473, 0.3543307086614173596, 1.953740157480315043 ) ) ;
#17039=CARTESIAN_POINT ( 'NONE',  ( 0.2860899518037616773, -0.4954156765914850546, 0.9399606299212598381 ) ) ;
#17043=CARTESIAN_POINT ( 'NONE',  ( -0.09660931395005634137, -0.3606853515406420185, -3.115157480314960647 ) ) ;
#17059=CARTESIAN_POINT ( 'NONE',  ( 0.5085118447801419972, 0.06699507805369840641, 1.766732283464566899 ) ) ;
#17063=CARTESIAN_POINT ( 'NONE',  ( -0.04679574315772200288, 0.3551931031211610357, -3.115157480314960647 ) ) ;
#17067=CARTESIAN_POINT ( 'NONE',  ( 0.2041304421298449356, -0.2660793235464211093, 1.973425196850393970 ) ) ;
#17071=CARTESIAN_POINT ( 'NONE',  ( 0.3001918266902269261, 0.3912931228431901776, -1.550196850393700920 ) ) ;
#17072=AXIS2_PLACEMENT_3D ( 'NONE', #23763, #1861, #8369 ) ;
#17092=CARTESIAN_POINT ( 'NONE',  ( -0.08600259748439828544, 0.1968503937007873850, -3.223068998490981496 ) ) ;
#17093=VERTEX_POINT ( 'NONE', #1742 ) ;
#17102=CARTESIAN_POINT ( 'NONE',  ( 0.5335524835332358107, -0.1429116519061119361, 0.9202755905511811330 ) ) ;
#17107=VECTOR ( 'NONE', #11146, 39.37007874015748143 ) ;
#17122=CARTESIAN_POINT ( 'NONE',  ( 0.4382482975805209735, 0.3362148458989007715, 0.9399606299212598381 ) ) ;
#17123=FACE_OUTER_BOUND ( 'NONE', #20679, .T. ) ;
#17128=ORIENTED_EDGE ( 'NONE', *, *, #25154, .F. ) ;
#17130=CARTESIAN_POINT ( 'NONE',  ( 0.1327036767636163017, -0.4954415918535808872, -1.550196850393700920 ) ) ;
#17134=CARTESIAN_POINT ( 'NONE',  ( 0.1711665596932999966, -0.5043892184459949357, 1.747047244094488194 ) ) ;
#17151=CARTESIAN_POINT ( 'NONE',  ( -0.3912931228432153796, -0.3001918266902245391, -1.569881889763779625 ) ) ;
#17153=CARTESIAN_POINT ( 'NONE',  ( -0.1458850421962410715, 0.4296318976989903504, -1.934055118110236338 ) ) ;
#17164=CARTESIAN_POINT ( 'NONE',  ( -0.3429848536917952662, -0.09193072188233032682, 1.953740157480315043 ) ) ;
#17166=CARTESIAN_POINT ( 'NONE',  ( -0.1431849087158744982, 0.4219262446672297773, -1.934055118110236116 ) ) ;
#17169=CARTESIAN_POINT ( 'NONE',  ( -0.04638120790932924453, 0.3520466617657084796, 1.953740157480315043 ) ) ;
#17171=CARTESIAN_POINT ( 'NONE',  ( -0.4218945342797526532, -0.1432577568504610210, -1.934055118110236338 ) ) ;
#17175=CARTESIAN_POINT ( 'NONE',  ( -0.4954156765914849991, -0.2860899518037616773, 0.9399606299212598381 ) ) ;
#17177=DIRECTION ( 'NONE',  ( 0.000000000000000000, 0.000000000000000000, 1.000000000000000000 ) ) ;
#17178=CARTESIAN_POINT ( 'NONE',  ( 0.3535721684717935132, 0.1200583359873110406, -3.115157480314960647 ) ) ;
#17193=CARTESIAN_POINT ( 'NONE',  ( 0.3855916753051394363, 0.3382184156732163660, 1.766732283464566899 ) ) ;
#17194=CARTESIAN_POINT ( 'NONE',  ( -0.4954415918530866159, 0.1327036767659691974, 1.747047244094488194 ) ) ;
#17198=CARTESIAN_POINT ( 'NONE',  ( 0.1791601451668926592, -0.3102476824511484210, -3.115157480314960647 ) ) ;
#17204=CARTESIAN_POINT ( 'NONE',  ( -0.1078280746904044657, 0.3175540113612282389, 1.973425196850393970 ) ) ;
#17224=CARTESIAN_POINT ( 'NONE',  ( -0.4351030398461813720, -0.1477428134820238381, -1.928289503579156294 ) ) ;
#17227=CARTESIAN_POINT ( 'NONE',  ( 0.4300129863948118913, 0.2478439864030018147, -1.569881889763779403 ) ) ;
#17230=B_SPLINE_CURVE_WITH_KNOTS ( 'NONE', 3,
 ( #738, #20223, #22625, #5535, #17935, #26707, #5243, #14158, #7224, #26855, #15988, #16135, #22155, #11014, #13125, #691, #24274, #21893 ),
 .UNSPECIFIED., .F., .F.,
 ( 4, 2, 2, 2, 2, 2, 2, 2, 4 ),
 ( 0.5000000000000000000, 0.5625000000000000000, 0.6250000000000001110, 0.6875000000000001110, 0.7500000000000001110, 0.8125000000000001110, 0.8750000000000000000, 0.9375000000000000000, 1.000000000000000000 ),
 .UNSPECIFIED. ) ;
#17236=( CONVERSION_BASED_UNIT ( 'INCH', #1839 ) LENGTH_UNIT ( ) NAMED_UNIT ( #25859 ) ) ;
#17241=CARTESIAN_POINT ( 'NONE',  ( 0.2442565704126255510, -0.4954197419817655823, 0.9202755905511811330 ) ) ;
#17249=ORIENTED_EDGE ( 'NONE', *, *, #23921, .F. ) ;
#17261=CARTESIAN_POINT ( 'NONE',  ( 0.4954156765914486393, 0.2860899518037346989, 0.9399606299212598381 ) ) ;
#17271=CARTESIAN_POINT ( 'NONE',  ( -0.07462150385364368921, -0.5672083774005965973, 0.9399606299212601712 ) ) ;
#17272=DIRECTION ( 'NONE',  ( 0.2588190448135640476, 3.169619147893065576E-17, -0.9659258263664939337 ) ) ;
#17278=DIRECTION ( 'NONE',  ( -0.000000000000000000, -0.000000000000000000, 1.000000000000000000 ) ) ;
#17287=CARTESIAN_POINT ( 'NONE',  ( 0.4498374011142918794, -0.05926487674658236643, -1.934055118110236338 ) ) ;
#17301=CARTESIAN_POINT ( 'NONE',  ( 0.1970998888482821121, 0.3995939286813822711, -1.934055118110236560 ) ) ;
#17305=CARTESIAN_POINT ( 'NONE',  ( -0.3411003281196917092, 0.2991932138496784521, -1.934055118110236338 ) ) ;
#17308=CARTESIAN_POINT ( 'NONE',  ( 0.5708661417322835607, 0.03736310157557569400, 0.9399606299212598381 ) ) ;
#17314=CARTESIAN_POINT ( 'NONE',  ( 0.2227473777839351354, -0.3858850602360253679, -1.934055118110236560 ) ) ;
#17329=B_SPLINE_CURVE_WITH_KNOTS ( 'NONE', 3,
 ( #10440, #22112, #13484, #8340, #25703, #23329, #21470, #10728, #10294, #2239, #16953, #6088, #21608, #15260, #25569, #10860, #4095, #12701 ),
 .UNSPECIFIED., .F., .F.,
 ( 4, 2, 2, 2, 2, 2, 2, 2, 4 ),
 ( 0.5000000000000000000, 0.5625000000000000000, 0.6250000000000000000, 0.6875000000000000000, 0.7500000000000000000, 0.8125000000000000000, 0.8750000000000000000, 0.9375000000000000000, 1.000000000000000000 ),
 .UNSPECIFIED. ) ;
#17332=CARTESIAN_POINT ( 'NONE',  ( 0.4069448477556011912, 0.3121994997598430133, 1.766732283464566899 ) ) ;
#17338=CARTESIAN_POINT ( 'NONE',  ( -0.3213305936751578717, -0.1584254766472200371, -3.115157480314960647 ) ) ;
#17344=CARTESIAN_POINT ( 'NONE',  ( -0.1482986320106521871, -0.3007905576423956506, 1.953740157480315043 ) ) ;
#17350=EDGE_LOOP ( 'NONE', ( #25036, #2822, #12550, #21495 ) ) ;
#17359=DIRECTION ( 'NONE',  ( -0.000000000000000000, -0.000000000000000000, 1.000000000000000000 ) ) ;
#17369=CARTESIAN_POINT ( 'NONE',  ( 0.06296589279854367116, 0.1968503937007873850, -3.224248289462122941 ) ) ;
#17372=CARTESIAN_POINT ( 'NONE',  ( 0.3937007874015748254, 0.000000000000000000, -3.115157480314960647 ) ) ;
#17374=CARTESIAN_POINT ( 'NONE',  ( 0.09842519685039370636, 0.2991866959364303802, -3.272637795275590733 ) ) ;
#17379=CARTESIAN_POINT ( 'NONE',  ( -0.4152525734086447429, -0.3642352168757386210, 0.9202755905511811330 ) ) ;
#17395=CARTESIAN_POINT ( 'NONE',  ( 0.5708661417322835607, -0.03736310157557555522, 0.9399606299212598381 ) ) ;
#17418=CARTESIAN_POINT ( 'NONE',  ( -0.4889536969035060410, 0.06441834428466772233, -1.550196850393700920 ) ) ;
#17419=CARTESIAN_POINT ( 'NONE',  ( 0.2031943647053748025, 0.4121342552748526455, -1.928289503579147190 ) ) ;
#17424=CARTESIAN_POINT ( 'NONE',  ( 0.3149606299212598381, 0.000000000000000000, -3.745078740157480546 ) ) ;
#17429=CARTESIAN_POINT ( 'NONE',  ( -0.1378076643338853602, -0.5144970376935932288, 1.747047244094488194 ) ) ;
#17430=FACE_BOUND ( 'NONE', #2428, .T. ) ;
#17438=ORIENTED_EDGE ( 'NONE', *, *, #5227, .T. ) ;
#17440=CARTESIAN_POINT ( 'NONE',  ( -0.3599896729929454864, 0.2761764805255169652, -1.934055118110236338 ) ) ;
#17445=CARTESIAN_POINT ( 'NONE',  ( 0.5131133041954354379, -0.2529800193559368360, 0.9399606299212598381 ) ) ;
#17451=CIRCLE ( 'NONE', #5260, 0.4921259842519685179 ) ;
#17452=DIRECTION ( 'NONE',  ( 0.000000000000000000, 0.000000000000000000, -1.000000000000000000 ) ) ;
#17453=CARTESIAN_POINT ( 'NONE',  ( -0.2962590301041646557, 0.2272836761397697136, -3.115157480314960647 ) ) ;
#17466=CARTESIAN_POINT ( 'NONE',  ( -0.4069448477556103505, 0.3121994997598293020, 1.766732283464566899 ) ) ;
#17467=CARTESIAN_POINT ( 'NONE',  ( -0.4069448477556027455, 0.3121994997598392940, 1.747047244094488194 ) ) ;
#17472=CARTESIAN_POINT ( 'NONE',  ( 0.2962590301041578278, 0.2272836761397798999, -3.115157480314960647 ) ) ;
#17498=CIRCLE ( 'NONE', #9896, 0.5905511811023621549 ) ;
#17499=CARTESIAN_POINT ( 'NONE',  ( -0.04956879678462303151, 0.2165354330708661457, -3.186635197791187757 ) ) ;
#17504=CARTESIAN_POINT ( 'NONE',  ( 0.2816986811832786208, -0.2161891097065020695, 1.953740157480315043 ) ) ;
#17506=DIRECTION ( 'NONE',  ( 0.000000000000000000, 0.000000000000000000, 1.000000000000000000 ) ) ;
#17514=CARTESIAN_POINT ( 'NONE',  ( 0.4954197419817713000, 0.2442565704126274662, 0.9399606299212598381 ) ) ;
#17527=ORIENTED_EDGE ( 'NONE', *, *, #16341, .T. ) ;
#17534=CARTESIAN_POINT ( 'NONE',  ( 0.1839420097223146422, 0.5417097841049177687, 0.9399606299212598381 ) ) ;
#17545=CARTESIAN_POINT ( 'NONE',  ( 0.3135473077061334268, 3.839847067635865072E-17, 2.504921259842519898 ) ) ;
#17565=CARTESIAN_POINT ( 'NONE',  ( -0.4270824798167697223, -0.2466292688015108703, -1.569881889763779625 ) ) ;
#17566=AXIS2_PLACEMENT_3D ( 'NONE', #26665, #20881, #975 ) ;
#17567=CARTESIAN_POINT ( 'NONE',  ( 0.3979194638820598984, -0.2297883689023126064, -1.928289503579157183 ) ) ;
#17568=CARTESIAN_POINT ( 'NONE',  ( 0.3454440660767517657, -0.3030032861724969440, -1.928289503579156516 ) ) ;
#17570=CARTESIAN_POINT ( 'NONE',  ( -0.2762247810519002922, 0.4783323773986519201, 0.9202755905511811330 ) ) ;
#17572=CARTESIAN_POINT ( 'NONE',  ( 0.09842519685039370636, 0.2991866959364303247, -3.548228346456693050 ) ) ;
#17582=CARTESIAN_POINT ( 'NONE',  ( 0.5118110236220472231, 3.133938659235352953E-17, 1.766732283464566899 ) ) ;
#17587=CARTESIAN_POINT ( 'NONE',  ( 0.02438677169350789847, 0.3726024258163779246, -3.115157480314960647 ) ) ;
#17591=CARTESIAN_POINT ( 'NONE',  ( 0.1288129352161812846, -0.4793172621399190425, -1.569881889763779403 ) ) ;
#17606=CARTESIAN_POINT ( 'NONE',  ( 0.04877294052295595012, 0.3702005978258479102, -3.115157480314960647 ) ) ;
#17612=CARTESIAN_POINT ( 'NONE',  ( 0.08676778863011140597, -0.3239425792934415571, 1.953740157480315043 ) ) ;
#17616=FACE_OUTER_BOUND ( 'NONE', #5904, .T. ) ;
#17622=CARTESIAN_POINT ( 'NONE',  ( 0.3765118517642104257, -2.263258471485603576E-17, -3.100567304031763172 ) ) ;
#17640=AXIS2_PLACEMENT_3D ( 'NONE', #24284, #22034, #4930 ) ;
#17642=CARTESIAN_POINT ( 'NONE',  ( 0.09842519685039370636, 0.5905905511811023745, -3.548228346456693050 ) ) ;
#17645=CARTESIAN_POINT ( 'NONE',  ( 0.3362148458988353239, 0.4382482975805538361, 0.9399606299212598381 ) ) ;
#17655=CARTESIAN_POINT ( 'NONE',  ( -0.5314960629921260393, 6.402768735150616610E-17, 1.747047244094488194 ) ) ;
#17657=B_SPLINE_CURVE_WITH_KNOTS ( 'NONE', 3,
 ( #12105, #27517, #27229, #1932, #1651, #19158, #10540, #21007, #21148, #18737, #25243, #4059, #14819, #19021, #10257, #25100, #22852, #8025, #25382, #5905, #12665, #27796, #20728, #25668, #1373, #9987, #18585, #14679, #23136, #27655, #22997, #7879, #8432, #1512 ),
 .UNSPECIFIED., .F., .F.,
 ( 4, 2, 2, 2, 2, 2, 2, 2, 2, 2, 2, 2, 2, 2, 2, 2, 4 ),
 ( 0.5000000000000000000, 0.5312500000000000000, 0.5625000000000000000, 0.5937500000000000000, 0.6250000000000000000, 0.6562500000000000000, 0.6875000000000000000, 0.7187500000000000000, 0.7500000000000000000, 0.7812500000000000000, 0.8125000000000000000, 0.8437500000000000000, 0.8750000000000000000, 0.9062500000000000000, 0.9375000000000000000, 0.9687500000000000000, 1.000000000000000000 ),
 .UNSPECIFIED. ) ;
#17658=CARTESIAN_POINT ( 'NONE',  ( -0.5671862884095228985, -0.07472527936312044206, 0.9399606299212598381 ) ) ;
#17659=CARTESIAN_POINT ( 'NONE',  ( 0.4092783051644229841, -0.3145317858139328737, 1.766732283464567121 ) ) ;
#17660=ORIENTED_EDGE ( 'NONE', *, *, #9364, .F. ) ;
#17661=DIRECTION ( 'NONE',  ( 0.000000000000000000, 0.000000000000000000, 1.000000000000000000 ) ) ;
#17678=ORIENTED_EDGE ( 'NONE', *, *, #10852, .T. ) ;
#17683=CARTESIAN_POINT ( 'NONE',  ( -0.3121994997578197428, 0.4069448477569481692, -1.550196850393700920 ) ) ;
#17684=CARTESIAN_POINT ( 'NONE',  ( 0.4121342552748534227, 0.2031943647053804092, -1.928289503579144304 ) ) ;
#17687=CARTESIAN_POINT ( 'NONE',  ( -0.4954197419817560344, 0.2442565704126489212, 0.9202755905511811330 ) ) ;
#17692=DIRECTION ( 'NONE',  ( 0.000000000000000000, 0.000000000000000000, 1.000000000000000000 ) ) ;
#17713=CARTESIAN_POINT ( 'NONE',  ( 0.4446035140077002623, -0.02917857698668054056, -1.934055118110235894 ) ) ;
#17714=CARTESIAN_POINT ( 'NONE',  ( -0.3644697409450256553, 0.09762295995070000010, -3.100567304031767168 ) ) ;
#17728=CARTESIAN_POINT ( 'NONE',  ( -0.1327036767659760530, 0.4954415918530867269, 1.747047244094488194 ) ) ;
#17732=CARTESIAN_POINT ( 'NONE',  ( 0.02438677169350789847, 0.3726024258163779246, -3.115157480314960647 ) ) ;
#17736=CARTESIAN_POINT ( 'NONE',  ( -0.1078280746903979848, 0.3175540113612246862, 1.953740157480315043 ) ) ;
#17737=EDGE_LOOP ( 'NONE', ( #3790, #1856, #13746, #22001 ) ) ;
#17745=CARTESIAN_POINT ( 'NONE',  ( -0.07874015748031511219, 0.1968503937007874127, -3.558551041376953883 ) ) ;
#17754=CYLINDRICAL_SURFACE ( 'NONE', #9179, 0.5118110236220472231 ) ;
#17758=CARTESIAN_POINT ( 'NONE',  ( -0.3543307086614173596, 0.02319089060378165187, 1.953740157480315043 ) ) ;
#17777=CARTESIAN_POINT ( 'NONE',  ( 0.07214854559195596484, 0.5476281405333121022, 0.9399606299212598381 ) ) ;
#17789=CARTESIAN_POINT ( 'NONE',  ( 0.1677079028045289355, -0.2904160862623609840, 1.953740157480315043 ) ) ;
#17817=CARTESIAN_POINT ( 'NONE',  ( 0.4921259842519685179, -0.03220957031753991784, -1.550196850393700920 ) ) ;
#17819=CARTESIAN_POINT ( 'NONE',  ( -0.3645739570812778219, -0.2796934465393718927, -1.928289503579152742 ) ) ;
#17820=CARTESIAN_POINT ( 'NONE',  ( -0.5118110236220472231, 0.000000000000000000, 1.914370078775489148 ) ) ;
#17824=CARTESIAN_POINT ( 'NONE',  ( 0.4921259842519685179, 2.987958743070287587E-17, -1.569881889763779625 ) ) ;
#17825=CARTESIAN_POINT ( 'NONE',  ( -0.4889536969035324643, 0.06441834428466573781, -1.569881889763779625 ) ) ;
#17840=CARTESIAN_POINT ( 'NONE',  ( 0.4069519308877018182, 0.2006393256663585589, -1.934055118110236338 ) ) ;
#17845=CARTESIAN_POINT ( 'NONE',  ( -0.3858850602361762472, -0.2227473777835706492, -1.934055118110236116 ) ) ;
#17846=CARTESIAN_POINT ( 'NONE',  ( -0.2993674444872340690, 0.2296683860596682170, -3.100567304031764060 ) ) ;
#17857=CARTESIAN_POINT ( 'NONE',  ( -0.03349795313264251895, -0.5118110236220472231, 1.747047244094488194 ) ) ;
#17859=CARTESIAN_POINT ( 'NONE',  ( -0.02438677169350859236, -0.3726024258163779246, -3.115157480314960647 ) ) ;
#17861=EDGE_LOOP ( 'NONE', ( #12402, #6756, #17923, #12072 ) ) ;
#17865=CARTESIAN_POINT ( 'NONE',  ( 0.04380447413658629385, 0.3324885138898144854, 1.953740157480315043 ) ) ;
#17868=VECTOR ( 'NONE', #15274, 39.37007874015748854 ) ;
#17875=CARTESIAN_POINT ( 'NONE',  ( -0.3551931031211768008, 0.04679574315772456333, -3.115157480314960647 ) ) ;
#17878=CARTESIAN_POINT ( 'NONE',  ( 0.01288382813972187464, 0.2165354330708661457, -3.174212598425197207 ) ) ;
#17879=CARTESIAN_POINT ( 'NONE',  ( 0.04638120790932724613, 0.3520466617656882735, 1.953740157480315043 ) ) ;
#17885=FACE_OUTER_BOUND ( 'NONE', #2212, .T. ) ;
#17894=CARTESIAN_POINT ( 'NONE',  ( 0.3937007874015748254, 0.000000000000000000, -1.934055118110236338 ) ) ;
#17898=VERTEX_POINT ( 'NONE', #1267 ) ;
#17899=CARTESIAN_POINT ( 'NONE',  ( 0.5671862884094760471, 0.07472527936312113594, 0.9399606299212598381 ) ) ;
#17913=CIRCLE ( 'NONE', #12555, 0.3937007874015748254 ) ;
#17923=ORIENTED_EDGE ( 'NONE', *, *, #8806, .F. ) ;
#17927=CARTESIAN_POINT ( 'NONE',  ( 0.09586345222253873921, 0.2165354330708661457, -3.573990933995916830 ) ) ;
#17935=CARTESIAN_POINT ( 'NONE',  ( 0.3010840436257780639, 0.2313841235333765900, -3.100567304031763616 ) ) ;
#17938=CARTESIAN_POINT ( 'NONE',  ( 0.09776461103677401565, 0.2994061874507674692, -3.561313241017925790 ) ) ;
#17939=CARTESIAN_POINT ( 'NONE',  ( -0.2268096725200260955, 0.4600326175569864340, -1.550196850393700920 ) ) ;
#17941=CARTESIAN_POINT ( 'NONE',  ( 0.5230301363771282519, -0.1775991818008710588, 0.9202755905511811330 ) ) ;
#17945=CARTESIAN_POINT ( 'NONE',  ( -0.1477428134820341077, 0.4351030398461640525, -1.928289503579168285 ) ) ;
#17948=CARTESIAN_POINT ( 'NONE',  ( 0.3707612262533184766, 0.3252100150720236282, -1.569881889763779625 ) ) ;
#17949=AXIS2_PLACEMENT_3D ( 'NONE', #9268, #11545, #7447 ) ;
#17953=EDGE_CURVE ( 'NONE', #16188, #724, #35, .T. ) ;
#17960=ORIENTED_EDGE ( 'NONE', *, *, #4364, .T. ) ;
#17961=CARTESIAN_POINT ( 'NONE',  ( 0.1173917140416251143, -0.4382752542995838052, -1.934055118110236338 ) ) ;
#17964=CYLINDRICAL_SURFACE ( 'NONE', #12362, 0.09842519685039378963 ) ;
#17971=CARTESIAN_POINT ( 'NONE',  ( -0.3535721684717733071, -0.1200583359873110406, -3.115157480314960647 ) ) ;
#17976=CARTESIAN_POINT ( 'NONE',  ( -0.3349573549949658169, 0.2938049579018958690, -1.934055118110236338 ) ) ;
#17978=EDGE_CURVE ( 'NONE', #21690, #7673, #6480, .T. ) ;
#17984=CARTESIAN_POINT ( 'NONE',  ( 0.4954415918531143714, 0.1327036767659736105, 1.747047244094488194 ) ) ;
#17989=CARTESIAN_POINT ( 'NONE',  ( -0.3606853515406215904, -0.09660931395005714628, -3.115157480314960647 ) ) ;
#17991=CARTESIAN_POINT ( 'NONE',  ( -2.685748425196850164E-17, 0.000000000000000000, -1.894685039405410665 ) ) ;
#18010=CARTESIAN_POINT ( 'NONE',  ( 0.3074993854542699689, 0.1775730735577541186, 1.953740157480315043 ) ) ;
#18015=FACE_OUTER_BOUND ( 'NONE', #5704, .T. ) ;
#18016=CARTESIAN_POINT ( 'NONE',  ( -0.2355331214654133032, 0.4777261797697266998, 1.747047244094488194 ) ) ;
#18021=ORIENTED_EDGE ( 'NONE', *, *, #3062, .T. ) ;
#18027=CARTESIAN_POINT ( 'NONE',  ( 0.4270824798167768277, 0.2466292688015001844, -1.569881889763779625 ) ) ;
#18030=CARTESIAN_POINT ( 'NONE',  ( -0.1839420097223304074, 0.5417097841048854612, 0.9399606299212598381 ) ) ;
#18033=DIRECTION ( 'NONE',  ( -1.000000000000000000, 0.000000000000000000, 0.000000000000000000 ) ) ;
#18042=CARTESIAN_POINT ( 'NONE',  ( -0.2660793235464189999, 0.2041304421298406335, 1.953740157480315043 ) ) ;
#18048=CARTESIAN_POINT ( 'NONE',  ( -0.5118110236220472231, 3.201384367575308305E-17, 1.766732283464566899 ) ) ;
#18049=B_SPLINE_CURVE_WITH_KNOTS ( 'NONE', 3,
 ( #21538, #12506, #6016, #2185 ),
 .UNSPECIFIED., .F., .F.,
 ( 4, 4 ),
 ( 0.000000000000000000, 1.000000000000000000 ),
 .UNSPECIFIED. ) ;
#18056=CARTESIAN_POINT ( 'NONE',  ( -0.09842519685039383126, 0.1968503937007873850, -3.548228346456693050 ) ) ;
#18071=CARTESIAN_POINT ( 'NONE',  ( 0.2180862235769456536, -0.4423390553432768879, -1.550196850393700920 ) ) ;
#18074=CARTESIAN_POINT ( 'NONE',  ( 0.5511811023622047445, -0.03607471876262466348, 0.9202755905511811330 ) ) ;
#18079=CARTESIAN_POINT ( 'NONE',  ( 0.4270824798167768277, 0.2466292688015001844, -1.569881889763779625 ) ) ;
#18087=MECHANICAL_DESIGN_GEOMETRIC_PRESENTATION_REPRESENTATION('',(#27153),#18552);
#18091=CARTESIAN_POINT ( 'NONE',  ( 0.09193127540178998303, 0.3429876364231002062, 1.953740157480315043 ) ) ;
#18093=CARTESIAN_POINT ( 'NONE',  ( 0.4382752542996382616, -0.1173917140416361471, -1.934055118110236338 ) ) ;
#18095=EDGE_CURVE ( 'NONE', #24094, #27336, #6142, .T. ) ;
#18101=VERTEX_POINT ( 'NONE', #18295 ) ;
#18102=VECTOR ( 'NONE', #1489, 39.37007874015748143 ) ;
#18106=CARTESIAN_POINT ( 'NONE',  ( 0.1668516812751446310, 0.3384212623783090512, -3.100567304031764948 ) ) ;
#18110=CARTESIAN_POINT ( 'NONE',  ( 0.2938049579018456314, -0.3349573549949907414, -1.934055118110236338 ) ) ;
#18113=ADVANCED_FACE ( 'NONE', ( #7031 ), #24727, .T. ) ;
#18118=CARTESIAN_POINT ( 'NONE',  ( 0.4856708409200641841, -0.1649135259617057481, 1.766732283464566899 ) ) ;
#18119=CARTESIAN_POINT ( 'NONE',  ( -0.1649135259616916205, -0.4856708409200665155, 1.747047244094488194 ) ) ;
#18125=CARTESIAN_POINT ( 'NONE',  ( 0.1668516812751341394, -0.3384212623783144913, -3.100567304031760951 ) ) ;
#18132=CARTESIAN_POINT ( 'NONE',  ( 0.03359157810797400862, 0.5118096047255845660, -1.550196850393700920 ) ) ;
#18137=CARTESIAN_POINT ( 'NONE',  ( 0.4303822302054278182, -0.1152775731717046309, -1.934055118110236338 ) ) ;
#18140=CARTESIAN_POINT ( 'NONE',  ( -0.06881018027188809394, 0.1968503937007874127, -3.587856484193131745 ) ) ;
#18143=CARTESIAN_POINT ( 'NONE',  ( 0.03962986251637121149, 0.1968503937007874127, -3.203822249701830494 ) ) ;
#18144=CARTESIAN_POINT ( 'NONE',  ( 0.07874015748031489015, 0.1968503937007874127, -3.272637795275590733 ) ) ;
#18145=CARTESIAN_POINT ( 'NONE',  ( 0.2924088307484721261, 0.1685339107540412829, 1.973425196850394192 ) ) ;
#18151=DIRECTION ( 'NONE',  ( -1.000000000000000000, 0.000000000000000000, 0.000000000000000000 ) ) ;
#18153=CARTESIAN_POINT ( 'NONE',  ( -0.2341512108694372152, -0.2669480828848191933, 1.953740157480315043 ) ) ;
#18162=CARTESIAN_POINT ( 'NONE',  ( -0.3512268162760389667, -0.4004221243553605092, 1.747047244094488194 ) ) ;
#18174=CARTESIAN_POINT ( 'NONE',  ( 0.4423390553432409722, -0.2180862235769587265, -1.569881889763779625 ) ) ;
#18175=ORIENTED_EDGE ( 'NONE', *, *, #7763, .T. ) ;
#18176=CARTESIAN_POINT ( 'NONE',  ( -0.3772436174784328244, 0.4300830224589641260, 0.9399606299212598381 ) ) ;
#18180=EDGE_CURVE ( 'NONE', #22130, #4351, #11463, .T. ) ;
#18209=CARTESIAN_POINT ( 'NONE',  ( 0.04956879678466356159, 0.1968503937007203553, -3.634230943941128888 ) ) ;
#18211=CARTESIAN_POINT ( 'NONE',  ( -0.5118110236220473341, 0.000000000000000000, -1.550196850393700920 ) ) ;
#18213=CARTESIAN_POINT ( 'NONE',  ( -0.07874015748031495954, 0.1968503937007874127, -3.456364829396325611 ) ) ;
#18225=CARTESIAN_POINT ( 'NONE',  ( 0.3346456692913385988, 0.02190250779246873461, 1.973425196850393970 ) ) ;
#18226=CARTESIAN_POINT ( 'NONE',  ( -0.2775852647713619725, 0.4816145447621894005, 0.9202755905511812440 ) ) ;
#18227=CARTESIAN_POINT ( 'NONE',  ( -0.3362148458988027944, 0.4382482975805537806, 0.9399606299212598381 ) ) ;
#18233=CARTESIAN_POINT ( 'NONE',  ( -0.4669911931914806358, 0.1585706980422473544, -1.569881889763779625 ) ) ;
#18243=PRODUCT_DEFINITION ( 'UNKNOWN', '', #9291, #23524 ) ;
#18259=ORIENTED_EDGE ( 'NONE', *, *, #15606, .F. ) ;
#18260=CARTESIAN_POINT ( 'NONE',  ( -0.02464264302293797324, 0.3765118517642104257, -3.100567304031763172 ) ) ;
#18263=CARTESIAN_POINT ( 'NONE',  ( 0.4218945342797220666, 0.1432577568504696530, -1.934055118110236338 ) ) ;
#18268=B_SPLINE_CURVE_WITH_KNOTS ( 'NONE', 3,
 ( #4959, #18213, #24725, #1156 ),
 .UNSPECIFIED., .F., .F.,
 ( 4, 4 ),
 ( 0.000000000000000000, 1.000000000000000000 ),
 .UNSPECIFIED. ) ;
#18271=CARTESIAN_POINT ( 'NONE',  ( 0.5085118447801136865, 0.06699507805368522251, 1.747047244094488194 ) ) ;
#18277=EDGE_CURVE ( 'NONE', #25, #10350, #5049, .T. ) ;
#18278=CARTESIAN_POINT ( 'NONE',  ( 0.3740848232703729015, -0.04928467685644277729, -3.100567304031765392 ) ) ;
#18295=CARTESIAN_POINT ( 'NONE',  ( 0.5905511811023621549, 0.000000000000000000, 1.707677165389662743 ) ) ;
#18299=CARTESIAN_POINT ( 'NONE',  ( -0.2056553984168023042, -0.2676050456844303871, 1.973425196850394636 ) ) ;
#18300=CARTESIAN_POINT ( 'NONE',  ( 0.3074993854542625304, -0.1775730735577552566, 1.953740157480315043 ) ) ;
#18309=CARTESIAN_POINT ( 'NONE',  ( 0.1378076643338917162, 0.5144970376936037759, 1.747047244094488194 ) ) ;
#18310=CARTESIAN_POINT ( 'NONE',  ( -0.4856708409200606313, -0.1649135259617140470, 1.766732283464566899 ) ) ;
#18314=CARTESIAN_POINT ( 'NONE',  ( -0.2842490391651705806, 0.2180698645301660521, -3.115157480314960647 ) ) ;
#18317=CARTESIAN_POINT ( 'NONE',  ( -0.4218945342797432163, 0.1432577568504689591, -1.934055118110236338 ) ) ;
#18323=CARTESIAN_POINT ( 'NONE',  ( 0.3252100150720381722, -0.3707612262533039327, -1.569881889763779625 ) ) ;
#18336=EDGE_LOOP ( 'NONE', ( #59, #21864, #8408, #23427 ) ) ;
#18348=EDGE_CURVE ( 'NONE', #5829, #5072, #8471, .T. ) ;
#18354=CARTESIAN_POINT ( 'NONE',  ( 0.06880207798751825088, 0.1968503937007873850, -3.587883383884366229 ) ) ;
#18363=CARTESIAN_POINT ( 'NONE',  ( -0.2660793235464223860, 0.2041304421298429095, 1.973425196850393970 ) ) ;
#18364=DIRECTION ( 'NONE',  ( 0.000000000000000000, 0.000000000000000000, 1.000000000000000000 ) ) ;
#18366=CARTESIAN_POINT ( 'NONE',  ( 0.5335524835332358107, -0.1429116519061119361, 0.9202755905511811330 ) ) ;
#18371=CARTESIAN_POINT ( 'NONE',  ( 0.2180862235769582824, 0.4423390553432410832, -1.569881889763779625 ) ) ;
#18376=CARTESIAN_POINT ( 'NONE',  ( -0.03488411621188159534, 0.5314946440730492494, 1.747047244094488638 ) ) ;
#18384=CARTESIAN_POINT ( 'NONE',  ( -0.2938622683360632148, 3.598774863079403804E-17, -3.745078740157480546 ) ) ;
#18391=CARTESIAN_POINT ( 'NONE',  ( -0.02963280468032113146, 0.4527559054764770385, -1.934055118110236338 ) ) ;
#18402=CARTESIAN_POINT ( 'NONE',  ( 0.2693761163850450502, -0.2361997806693590662, -3.115157480314961091 ) ) ;
#18407=CARTESIAN_POINT ( 'NONE',  ( -0.2006393256663633884, 0.4069519308876736741, -1.934055118110236338 ) ) ;
#18416=CARTESIAN_POINT ( 'NONE',  ( -0.2355331214654133032, 0.4777261797697266998, 1.747047244094488194 ) ) ;
#18420=CARTESIAN_POINT ( 'NONE',  ( -0.04928467685643870416, 0.3740848232703742893, -3.100567304031763172 ) ) ;
#18428=ORIENTED_EDGE ( 'NONE', *, *, #12146, .T. ) ;
#18429=CARTESIAN_POINT ( 'NONE',  ( 0.4417361510194462992, 0.05819755867304002989, -1.934055118110236338 ) ) ;
#18432=CARTESIAN_POINT ( 'NONE',  ( 0.1791601451668921319, 0.3102476824511487541, -3.115157480314960647 ) ) ;
#18433=CARTESIAN_POINT ( 'NONE',  ( -0.2775852647713620280, -0.4816145447621894560, 0.9202755905511813550 ) ) ;
#18437=CYLINDRICAL_SURFACE ( 'NONE', #4483, 0.3149606299212598381 ) ;
#18440=CARTESIAN_POINT ( 'NONE',  ( -0.09842519685039370636, 0.2165354330708661457, -3.272637795275590733 ) ) ;
#18451=CARTESIAN_POINT ( 'NONE',  ( -0.03478633594543723007, 0.5314960629921260393, 1.747047244094488194 ) ) ;
#18453=CARTESIAN_POINT ( 'NONE',  ( -0.3855916753051542023, -0.3382184156732014890, 1.766732283464566899 ) ) ;
#18461=ORIENTED_EDGE ( 'NONE', *, *, #556, .F. ) ;
#18463=CARTESIAN_POINT ( 'NONE',  ( 0.06441834428467232976, 0.4889536969035311875, -1.569881889763779625 ) ) ;
#18468=ORIENTED_EDGE ( 'NONE', *, *, #22982, .T. ) ;
#18491=VERTEX_POINT ( 'NONE', #9193 ) ;
#18506=EDGE_CURVE ( 'NONE', #7118, #1047, #17230, .T. ) ;
#18508=CARTESIAN_POINT ( 'NONE',  ( 0.02190250779246040100, 0.3346456692913385988, 1.973425196850393970 ) ) ;
#18510=CARTESIAN_POINT ( 'NONE',  ( 0.3121994997578124154, -0.4069448477569433953, -1.550196850393700920 ) ) ;
#18512=CARTESIAN_POINT ( 'NONE',  ( -0.5511811023622046335, 0.07214943758244282690, 0.9202755905511811330 ) ) ;
#18514=CARTESIAN_POINT ( 'NONE',  ( -0.4152525734086447429, -0.3642352168757386210, 0.9202755905511811330 ) ) ;
#18520=CARTESIAN_POINT ( 'NONE',  ( 0.3765118517642103146, -0.04928528614549727849, -3.100567304031763172 ) ) ;
#18547=CARTESIAN_POINT ( 'NONE',  ( -0.04673558830912487999, -0.3552036222398666232, -3.115157480314960647 ) ) ;
#18550=CARTESIAN_POINT ( 'NONE',  ( -0.02909913904662018644, 0.4446020952038907681, -1.934055118110236338 ) ) ;
#18552=( GEOMETRIC_REPRESENTATION_CONTEXT ( 3 ) GLOBAL_UNCERTAINTY_ASSIGNED_CONTEXT ( ( #5368 ) ) GLOBAL_UNIT_ASSIGNED_CONTEXT ( ( #4839, #15858, #22362 ) ) REPRESENTATION_CONTEXT ( 'NONE', 'WORKASPACE' ) ) ;
#18556=CARTESIAN_POINT ( 'NONE',  ( -0.4225965726692976765, -0.3242071728275119913, 1.747047244094488194 ) ) ;
#18557=ORIENTED_EDGE ( 'NONE', *, *, #20021, .T. ) ;
#18567=CARTESIAN_POINT ( 'NONE',  ( -0.05819755867304135522, -0.4417361510194244278, -1.934055118110236338 ) ) ;
#18574=CARTESIAN_POINT ( 'NONE',  ( 0.1791601451668926592, -0.3102476824511484210, -3.115157480314960647 ) ) ;
#18576=CARTESIAN_POINT ( 'NONE',  ( -0.2924088307484721261, 0.1685339107540411718, 1.973425196850393526 ) ) ;
#18577=CARTESIAN_POINT ( 'NONE',  ( 0.000000000000000000, 0.000000000000000000, 2.426181102355854158 ) ) ;
#18585=CARTESIAN_POINT ( 'NONE',  ( -0.4538399017594920148, 0.3483099419441555988, 0.9399606299212600602 ) ) ;
#18586=CARTESIAN_POINT ( 'NONE',  ( 0.5118110236220472231, 0.000000000000000000, 1.747047244094488194 ) ) ;
#18589=VERTEX_POINT ( 'NONE', #17374 ) ;
#18592=CARTESIAN_POINT ( 'NONE',  ( 0.03349795313264414959, -0.5118110236220472231, 1.747047244094488194 ) ) ;
#18594=CARTESIAN_POINT ( 'NONE',  ( 0.1649135259616801574, 0.4856708409200201637, 1.747047244094488194 ) ) ;
#18603=EDGE_CURVE ( 'NONE', #18589, #10030, #25990, .T. ) ;
#18605=CARTESIAN_POINT ( 'NONE',  ( 0.3346456692913385988, 0.02190250779246873461, 1.973425196850393970 ) ) ;
#18609=CARTESIAN_POINT ( 'NONE',  ( -0.1585706980422471879, 0.4669911931914806913, -1.569881889763779625 ) ) ;
#18615=EDGE_CURVE ( 'NONE', #2791, #5588, #9432, .T. ) ;
#18616=CARTESIAN_POINT ( 'NONE',  ( -0.3726024258163779246, 4.563063681305663643E-17, -3.115157480314960647 ) ) ;
#18631=VERTEX_POINT ( 'NONE', #24004 ) ;
#18651=CARTESIAN_POINT ( 'NONE',  ( 0.3175540113612324578, -0.1078280746903944320, 1.973425196850393970 ) ) ;
#18652=CARTESIAN_POINT ( 'NONE',  ( 0.4069448477569526101, -0.3121994997578271813, -1.550196850393700920 ) ) ;
#18656=CARTESIAN_POINT ( 'NONE',  ( 0.2442565704126313797, -0.4954197419817796266, 0.9399606299212598381 ) ) ;
#18662=CARTESIAN_POINT ( 'NONE',  ( 0.03965503742771028101, 0.1968503937007873850, -3.203835717288081142 ) ) ;
#18688=CARTESIAN_POINT ( 'NONE',  ( 0.3707612262533033776, -0.3252100150720387273, -1.569881889763779625 ) ) ;
#18690=ADVANCED_FACE ( 'NONE', ( #12260 ), #19380, .T. ) ;
#18693=CARTESIAN_POINT ( 'NONE',  ( -0.2712027394948519632, -0.3535065162672669792, -1.934055118110236338 ) ) ;
#18694=CARTESIAN_POINT ( 'NONE',  ( -0.3979194638820524044, 0.2297883689023302312, -1.928289503579153630 ) ) ;
#18702=CARTESIAN_POINT ( 'NONE',  ( 0.5280699926562892887, 0.06957181182498746452, 1.747047244094488194 ) ) ;
#18708=CARTESIAN_POINT ( 'NONE',  ( 0.3740848232703748444, 0.04928467685643974500, -3.100567304031760507 ) ) ;
#18709=DIRECTION ( 'NONE',  ( 1.000000000000000000, 0.000000000000000000, 0.000000000000000000 ) ) ;
#18713=CARTESIAN_POINT ( 'NONE',  ( -0.2161381151963043257, -0.2817310484609166221, 1.953740157480315043 ) ) ;
#18717=CARTESIAN_POINT ( 'NONE',  ( -0.3765118517642103702, -0.04928528614549713277, -3.100567304031763172 ) ) ;
#18718=CARTESIAN_POINT ( 'NONE',  ( 0.1480156394741987402, 0.5526079293737075071, 0.9399606299212598381 ) ) ;
#18719=FACE_OUTER_BOUND ( 'NONE', #17861, .T. ) ;
#18725=CARTESIAN_POINT ( 'NONE',  ( -0.1791601451668828893, 0.3102476824511414266, -3.115157480314960647 ) ) ;
#18734=CARTESIAN_POINT ( 'NONE',  ( 0.3543307086614173596, 0.000000000000000000, 1.953740157480315043 ) ) ;
#18737=CARTESIAN_POINT ( 'NONE',  ( 0.3771696032822623446, 0.4301590433674484792, 0.9399606299212601712 ) ) ;
#18742=CARTESIAN_POINT ( 'NONE',  ( 0.4004221243553557907, -0.3512268162760437407, 1.747047244094488194 ) ) ;
#18744=CARTESIAN_POINT ( 'NONE',  ( -0.4954415918530857832, 0.1327036767659614813, 1.766732283464566899 ) ) ;
#18751=DIRECTION ( 'NONE',  ( 0.000000000000000000, 0.000000000000000000, 1.000000000000000000 ) ) ;
#18753=CARTESIAN_POINT ( 'NONE',  ( -0.04380447413658894451, -0.3324885138898239778, 1.973425196850393970 ) ) ;
#18775=DIRECTION ( 'NONE',  ( -0.000000000000000000, 0.000000000000000000, -1.000000000000000000 ) ) ;
#18777=ADVANCED_FACE ( 'NONE', ( #22437 ), #5743, .T. ) ;
#18778=CARTESIAN_POINT ( 'NONE',  ( 0.4442166144915702941, 0.2564158049319635868, -1.550196850393700476 ) ) ;
#18785=CARTESIAN_POINT ( 'NONE',  ( -0.5511811023622047445, 0.03607471876259063515, 0.9202755905511811330 ) ) ;
#18789=CARTESIAN_POINT ( 'NONE',  ( 0.000000000000000000, 0.000000000000000000, 2.426181102355854158 ) ) ;
#18791=CARTESIAN_POINT ( 'NONE',  ( -0.09842519685039385902, 0.2165354330708661457, -3.561114497143080815 ) ) ;
#18794=CARTESIAN_POINT ( 'NONE',  ( 0.4857079805366297243, -0.1648275707506031140, -1.550196850393700254 ) ) ;
#18796=CARTESIAN_POINT ( 'NONE',  ( 0.2041304421298423266, 0.2660793235464414264, 1.953740157480315043 ) ) ;
#18797=CARTESIAN_POINT ( 'NONE',  ( 0.2268096725200246799, -0.4600326175569940945, -1.550196850393700920 ) ) ;
#18801=CARTESIAN_POINT ( 'NONE',  ( -0.1775991818008371415, -0.5230301363771194811, 0.9399606299212598381 ) ) ;
#18811=CARTESIAN_POINT ( 'NONE',  ( -0.4270824798167792147, -0.2466292688015026546, -1.550196850393700920 ) ) ;
#18816=CARTESIAN_POINT ( 'NONE',  ( -0.06947563356185801342, -0.5280876769849813801, 1.747047244094488194 ) ) ;
#18825=AXIS2_PLACEMENT_3D ( 'NONE', #24337, #757, #11907 ) ;
#18828=CARTESIAN_POINT ( 'NONE',  ( 0.3574989824755537837, -0.02345921195965521011, -3.115157480314960647 ) ) ;
#18831=CARTESIAN_POINT ( 'NONE',  ( -0.1173917140416340377, 0.4382752542996236622, -1.934055118110236338 ) ) ;
#18832=EDGE_CURVE ( 'NONE', #5287, #17093, #21938, .T. ) ;
#18840=CARTESIAN_POINT ( 'NONE',  ( -0.4225965726692971769, 0.3242071728275127129, 1.747047244094488194 ) ) ;
#18847=CARTESIAN_POINT ( 'NONE',  ( 0.3184841198566381593, 0.1570220809524529026, 1.953740157480315043 ) ) ;
#18854=CARTESIAN_POINT ( 'NONE',  ( 0.07214854559198032036, -0.5476281405333571772, 0.9399606299212598381 ) ) ;
#18861=B_SPLINE_CURVE_WITH_KNOTS ( 'NONE', 2,
 ( #8027, #18586, #21150 ),
 .UNSPECIFIED., .F., .F.,
 ( 3, 3 ),
 ( 0.000000000000000000, 1.000000000000000000 ),
 .UNSPECIFIED. ) ;
#18863=CARTESIAN_POINT ( 'NONE',  ( 0.04679574315772527804, -0.3551931031211721379, -3.115157480314960647 ) ) ;
#18874=FACE_OUTER_BOUND ( 'NONE', #11770, .T. ) ;
#18879=CARTESIAN_POINT ( 'NONE',  ( 0.5118110236220472231, 0.03349795313260757468, 1.747047244094488194 ) ) ;
#18884=DIRECTION ( 'NONE',  ( 0.000000000000000000, 0.000000000000000000, 1.000000000000000000 ) ) ;
#18886=VECTOR ( 'NONE', #26837, 39.37007874015748143 ) ;
#18889=CARTESIAN_POINT ( 'NONE',  ( -0.2041304421298332783, 0.2660793235464289364, 1.973425196850393970 ) ) ;
#18892=CARTESIAN_POINT ( 'NONE',  ( -0.1275996891957763835, -0.4763861460130486281, -1.550196850393700920 ) ) ;
#18899=CARTESIAN_POINT ( 'NONE',  ( -0.3726024258163779246, 0.000000000000000000, -3.115157480314960647 ) ) ;
#18926=( NAMED_UNIT ( * ) PLANE_ANGLE_UNIT ( ) SI_UNIT ( $, .RADIAN. ) ) ;
#18933=CARTESIAN_POINT ( 'NONE',  ( -0.4783323773986817851, 0.2762247810518556612, 0.9202755905511811330 ) ) ;
#18945=CARTESIAN_POINT ( 'NONE',  ( 0.1677079028045344034, -0.2904160862623691997, 1.973425196850393970 ) ) ;
#18951=CARTESIAN_POINT ( 'NONE',  ( -0.5511811023622048555, 0.000000000000000000, 0.9399606299212598381 ) ) ;
#18955=AXIS2_PLACEMENT_3D ( 'NONE', #12585, #25441, #3376 ) ;
#18958=CARTESIAN_POINT ( 'NONE',  ( -0.5118110236220473341, 0.000000000000000000, -1.550196850393700920 ) ) ;
#18980=CARTESIAN_POINT ( 'NONE',  ( 0.3574975638436101444, 4.268512490100411279E-17, -3.115157480314960647 ) ) ;
#18983=CARTESIAN_POINT ( 'NONE',  ( -0.4498374011143459472, -0.05926487674658267174, -1.934055118110236338 ) ) ;
#18991=CARTESIAN_POINT ( 'NONE',  ( 0.06699507805368110080, -0.5085118447801203478, 1.747047244094488194 ) ) ;
#18998=CARTESIAN_POINT ( 'NONE',  ( 0.4303653410901771004, 0.1153552079391450824, -1.934055118110237004 ) ) ;
#19000=CARTESIAN_POINT ( 'NONE',  ( -0.3520466617656974884, -0.04638120790932648285, 1.953740157480315043 ) ) ;
#19011=CARTESIAN_POINT ( 'NONE',  ( 0.2842490391651533721, -0.2180698645301867300, -3.115157480314960647 ) ) ;
#19014=CARTESIAN_POINT ( 'NONE',  ( 0.5314960629921260393, 0.000000000000000000, 1.747047244094488194 ) ) ;
#19019=EDGE_CURVE ( 'NONE', #27336, #7980, #6086, .T. ) ;
#19021=CARTESIAN_POINT ( 'NONE',  ( 0.1838445375787389757, 0.5417516942597615515, 0.9399606299212601712 ) ) ;
#19024=CARTESIAN_POINT ( 'NONE',  ( 0.01288382813972203597, 0.2165354330708660902, -3.646653543307087020 ) ) ;
#19030=CARTESIAN_POINT ( 'NONE',  ( -0.2362439534887390002, -0.2693339498142257038, -3.115157480314960647 ) ) ;
#19031=FACE_BOUND ( 'NONE', #25995, .T. ) ;
#19034=CARTESIAN_POINT ( 'NONE',  ( 0.1482986320106470801, -0.3007905576423859917, 1.973425196850393970 ) ) ;
#19037=EDGE_CURVE ( 'NONE', #22996, #12810, #17451, .T. ) ;
#19039=CARTESIAN_POINT ( 'NONE',  ( -0.1275996891957738577, 0.4763861460130593972, -1.550196850393700920 ) ) ;
#19068=EDGE_CURVE ( 'NONE', #26373, #12810, #6648, .T. ) ;
#19072=CARTESIAN_POINT ( 'NONE',  ( 0.4382482975805264136, 0.3362148458988503674, 0.9202755905511811330 ) ) ;
#19088=CARTESIAN_POINT ( 'NONE',  ( 0.3362148458988509225, -0.4382482975804891101, 0.9399606299212598381 ) ) ;
#19093=CARTESIAN_POINT ( 'NONE',  ( 0.3102827802122046230, 0.1791101711255022044, -3.115157480314962424 ) ) ;
#19099=VERTEX_POINT ( 'NONE', #2251 ) ;
#19100=CARTESIAN_POINT ( 'NONE',  ( 0.2268096725200246799, -0.4600326175569940945, -1.550196850393700920 ) ) ;
#19102=CARTESIAN_POINT ( 'NONE',  ( 0.1481199686343411814, -0.5525886237723267591, 0.9399606299212601712 ) ) ;
#19105=CARTESIAN_POINT ( 'NONE',  ( -0.03488411621167891719, -0.5314974819112028293, 1.747047244094488194 ) ) ;
#19121=CARTESIAN_POINT ( 'NONE',  ( -0.4555658499976060760, 0.06001958459474820984, -1.928289503579160513 ) ) ;
#19122=CARTESIAN_POINT ( 'NONE',  ( 0.4438564651657541105, -0.1188866373884811950, -1.928289503579147857 ) ) ;
#19137=CARTESIAN_POINT ( 'NONE',  ( -0.5708661417322834497, 0.000000000000000000, 0.9399606299212598381 ) ) ;
#19140=CARTESIAN_POINT ( 'NONE',  ( 0.1141709026133613525, -0.3362336590883617249, 1.953740157480315043 ) ) ;
#19148=AXIS2_PLACEMENT_3D ( 'NONE', #1002, #9590, #26413 ) ;
#19149=CARTESIAN_POINT ( 'NONE',  ( -0.1200583359873150374, -0.3535721684717939017, -3.115157480314960647 ) ) ;
#19158=CARTESIAN_POINT ( 'NONE',  ( 0.5130740159365840825, 0.2530785775239950963, 0.9399606299212597271 ) ) ;
#19165=CARTESIAN_POINT ( 'NONE',  ( 0.5280699926562971713, -0.06957181182499251604, 1.747047244094488194 ) ) ;
#19166=CARTESIAN_POINT ( 'NONE',  ( 0.4954415918530860607, 0.1327036767659604266, 1.766732283464566899 ) ) ;
#19171=CARTESIAN_POINT ( 'NONE',  ( -0.3574975638436101444, -0.02339816079122979120, -3.115157480314960647 ) ) ;
#19179=CARTESIAN_POINT ( 'NONE',  ( -0.1482986320106401412, 0.3007905576423888783, 1.973425196850393970 ) ) ;
#19183=CARTESIAN_POINT ( 'NONE',  ( 0.4270824798167662806, 0.2466292688014931900, -1.550196850393700920 ) ) ;
#19192=VERTEX_POINT ( 'NONE', #17894 ) ;
#19207=CARTESIAN_POINT ( 'NONE',  ( 0.09842519685039363697, 0.2165354330708661457, -3.259751644589254482 ) ) ;
#19215=CARTESIAN_POINT ( 'NONE',  ( 0.5511811023622047445, -0.03607471876262466348, 0.9202755905511811330 ) ) ;
#19229=CARTESIAN_POINT ( 'NONE',  ( 0.3346456692913385988, -0.02190250779246876237, 1.973425196850393970 ) ) ;
#19233=ADVANCED_FACE ( 'NONE', ( #4644 ), #10016, .T. ) ;
#19234=CARTESIAN_POINT ( 'NONE',  ( 0.5230301363770953893, -0.1775991818008574585, 0.9399606299212598381 ) ) ;
#19236=CYLINDRICAL_SURFACE ( 'NONE', #21394, 0.09842519685039378963 ) ;
#19238=CARTESIAN_POINT ( 'NONE',  ( 0.1584824234590462289, 0.3213085410495249983, -3.115157480314959759 ) ) ;
#19246=CARTESIAN_POINT ( 'NONE',  ( -0.4423390553432768879, -0.2180862235769457091, -1.550196850393700920 ) ) ;
#19247=CARTESIAN_POINT ( 'NONE',  ( 0.5525858403826197085, -0.1481194149833565954, 0.9399606299212598381 ) ) ;
#19263=CARTESIAN_POINT ( 'NONE',  ( 0.1275996891957731083, 0.4763861460130595082, -1.550196850393700920 ) ) ;
#19264=CARTESIAN_POINT ( 'NONE',  ( -0.4382752542995838052, -0.1173917140416377847, -1.934055118110236338 ) ) ;
#19273=CARTESIAN_POINT ( 'NONE',  ( 0.5314960629921260393, 0.000000000000000000, 1.747047244094488194 ) ) ;
#19281=CARTESIAN_POINT ( 'NONE',  ( -0.1153552079393971586, 0.4303653410901769893, -1.934055118110237004 ) ) ;
#19283=CARTESIAN_POINT ( 'NONE',  ( 0.2817310484609266696, -0.2161381151962942504, 1.953740157480315043 ) ) ;
#19287=CARTESIAN_POINT ( 'NONE',  ( -0.3772436174784659646, -0.4300830224589956563, 0.9399606299212598381 ) ) ;
#19291=CARTESIAN_POINT ( 'NONE',  ( -0.1867299569291685502, -0.3233561589689051829, -3.115157480314960647 ) ) ;
#19292=CARTESIAN_POINT ( 'NONE',  ( -0.08600259727896251982, 0.2165354330708660902, -3.597797143737292203 ) ) ;
#19308=CARTESIAN_POINT ( 'NONE',  ( -0.2268096725222462362, 0.4600326175560554565, 1.766732283464566899 ) ) ;
#19309=CARTESIAN_POINT ( 'NONE',  ( -0.2268096725222397969, 0.4600326175560398023, 1.747047244094488194 ) ) ;
#19312=CARTESIAN_POINT ( 'NONE',  ( 0.3102476824511487541, -0.1791601451668820011, -3.115157480314960647 ) ) ;
#19318=CARTESIAN_POINT ( 'NONE',  ( 0.1078280746904042159, 0.3175540113612283499, 1.973425196850393970 ) ) ;
#19319=EDGE_LOOP ( 'NONE', ( #1043, #24239 ) ) ;
#19326=ORIENTED_EDGE ( 'NONE', *, *, #3202, .T. ) ;
#19346=CARTESIAN_POINT ( 'NONE',  ( 0.06048688226688470060, 0.1968503937007873850, -3.193930429277340277 ) ) ;
#19357=CARTESIAN_POINT ( 'NONE',  ( -0.4783323773986509764, -0.2762247810519017355, 0.9202755905511811330 ) ) ;
#19376=EDGE_CURVE ( 'NONE', #20990, #25275, #18861, .T. ) ;
#19379=CARTESIAN_POINT ( 'NONE',  ( 0.02345921195965492909, 0.3574989824755535617, -3.115157480314959759 ) ) ;
#19380=CONICAL_SURFACE ( 'NONE', #17566, 0.4527559054764771496, 0.7853981642949022790 ) ;
#19386=CARTESIAN_POINT ( 'NONE',  ( -0.3121994997578197428, 0.4069448477569481692, -1.550196850393700920 ) ) ;
#19393=ORIENTED_EDGE ( 'NONE', *, *, #20021, .F. ) ;
#19401=CIRCLE ( 'NONE', #2246, 0.5905511811023621549 ) ;
#19406=CARTESIAN_POINT ( 'NONE',  ( -0.3912931228432124930, 0.3001918266902225407, -1.550196850393700920 ) ) ;
#19408=CARTESIAN_POINT ( 'NONE',  ( 0.3411003281197156900, -0.2991932138496291582, -1.934055118110236338 ) ) ;
#19413=ORIENTED_EDGE ( 'NONE', *, *, #23798, .T. ) ;
#19419=B_SPLINE_CURVE_WITH_KNOTS ( 'NONE', 2,
 ( #8254, #11674, #18144 ),
 .UNSPECIFIED., .F., .F.,
 ( 3, 3 ),
 ( 0.000000000000000000, 1.000000000000000000 ),
 .UNSPECIFIED. ) ;
#19425=ADVANCED_FACE ( 'NONE', ( #21020 ), #6431, .T. ) ;
#19426=CARTESIAN_POINT ( 'NONE',  ( -0.3858397471888894703, -0.2228126397719936702, -1.934055118110236338 ) ) ;
#19433=CARTESIAN_POINT ( 'NONE',  ( 0.3349073414797994475, -0.1651192144506243853, -3.115157480314960647 ) ) ;
#19447=CARTESIAN_POINT ( 'NONE',  ( -0.2564944395515793563, -0.4441657790107725323, 1.747047244094488194 ) ) ;
#19450=ORIENTED_EDGE ( 'NONE', *, *, #25880, .F. ) ;
#19452=CARTESIAN_POINT ( 'NONE',  ( -0.3726024258163779246, 0.000000000000000000, -3.115157480314960647 ) ) ;
#19457=CARTESIAN_POINT ( 'NONE',  ( -0.2660793235464189999, 0.2041304421298406335, 1.953740157480315043 ) ) ;
#19471=CARTESIAN_POINT ( 'NONE',  ( -0.4613022222206683010, 0.2662775206743746015, 1.747047244094488416 ) ) ;
#19480=CARTESIAN_POINT ( 'NONE',  ( -0.06048688226689052927, 0.2165354330708661457, -3.193930429277413108 ) ) ;
#19491=EDGE_LOOP ( 'NONE', ( #15875, #15387, #412, #1115 ) ) ;
#19492=CARTESIAN_POINT ( 'NONE',  ( -0.4954197419817713000, -0.2442565704126117565, 0.9202755905511811330 ) ) ;
#19516=CARTESIAN_POINT ( 'NONE',  ( 0.5526079293737398146, 0.1480156394741914405, 0.9399606299212598381 ) ) ;
#19528=ORIENTED_EDGE ( 'NONE', *, *, #18506, .F. ) ;
#19530=CARTESIAN_POINT ( 'NONE',  ( 0.4301590433675085978, -0.3771696032822019484, 0.9399606299212598381 ) ) ;
#19535=CARTESIAN_POINT ( 'NONE',  ( -0.5511811023268710086, 0.000000000000000000, 1.747047244094488194 ) ) ;
#19544=ORIENTED_EDGE ( 'NONE', *, *, #7789, .F. ) ;
#19546=CARTESIAN_POINT ( 'NONE',  ( -0.4669911931914798586, -0.1585706980422492696, -1.569881889763779625 ) ) ;
#19548=CARTESIAN_POINT ( 'NONE',  ( 0.4555658499976260600, 0.06001958459474954211, -1.928289503579140529 ) ) ;
#19552=ADVANCED_FACE ( 'NONE', ( #27345 ), #14358, .T. ) ;
#19556=CARTESIAN_POINT ( 'NONE',  ( 0.3242071728275346953, -0.4225965726692721969, 1.747047244094488194 ) ) ;
#19579=CARTESIAN_POINT ( 'NONE',  ( -0.02917857698710797643, -0.4446035140077002623, -1.934055118110236338 ) ) ;
#19580=CARTESIAN_POINT ( 'NONE',  ( -0.2962590301041579388, -0.2272836761397900585, -3.115157480314960647 ) ) ;
#19594=CARTESIAN_POINT ( 'NONE',  ( 0.03349795313264332386, 0.5118110236220472231, 1.766732283464566899 ) ) ;
#19599=VERTEX_POINT ( 'NONE', #16463 ) ;
#19601=CARTESIAN_POINT ( 'NONE',  ( 0.3551931031211721379, 0.04679574315772513232, -3.115157480314960647 ) ) ;
#19602=ORIENTED_EDGE ( 'NONE', *, *, #26134, .T. ) ;
#19603=EDGE_LOOP ( 'NONE', ( #1907, #977, #25288, #3398 ) ) ;
#19608=CARTESIAN_POINT ( 'NONE',  ( -0.2211428102655905170, 0.2521176338356723168, 1.953740157480315043 ) ) ;
#19625=CARTESIAN_POINT ( 'NONE',  ( -0.5144793533647340489, 0.1379038425975085413, 1.747047244094487972 ) ) ;
#19644=CARTESIAN_POINT ( 'NONE',  ( 0.3642352168757886366, 0.4152525734086595088, 0.9399606299212598381 ) ) ;
#19648=VERTEX_POINT ( 'NONE', #19137 ) ;
#19649=CARTESIAN_POINT ( 'NONE',  ( 0.000000000000000000, 0.000000000000000000, 1.953740157480315043 ) ) ;
#19657=CARTESIAN_POINT ( 'NONE',  ( -0.09842519685039366473, 0.1968503937007873850, -3.456364829396323390 ) ) ;
#19663=CARTESIAN_POINT ( 'NONE',  ( -0.1839420097223304074, 0.5417097841048854612, 0.9399606299212598381 ) ) ;
#19675=CARTESIAN_POINT ( 'NONE',  ( -0.3122781343789607367, 0.4068940122751343869, -1.550196850393701142 ) ) ;
#19690=CARTESIAN_POINT ( 'NONE',  ( 0.4270824798167662806, 0.2466292688014931900, -1.550196850393700920 ) ) ;
#19692=CARTESIAN_POINT ( 'NONE',  ( 0.3030032861725032167, 0.3454440660767328364, -1.928289503579165620 ) ) ;
#19695=AXIS2_PLACEMENT_3D ( 'NONE', #22904, #14588, #22614 ) ;
#19714=CARTESIAN_POINT ( 'NONE',  ( -0.1431838228103958222, -0.4219236230597716575, -1.934055118110236560 ) ) ;
#19715=CARTESIAN_POINT ( 'NONE',  ( -0.1651192144506347381, 0.3349073414798414139, -3.115157480314960647 ) ) ;
#19726=CARTESIAN_POINT ( 'NONE',  ( 0.1649135259617122706, 0.4856708409200614640, 1.766732283464566899 ) ) ;
#19732=CARTESIAN_POINT ( 'NONE',  ( 0.2807137536170459802, 0.2462256503456008716, -3.115157480314960647 ) ) ;
#19736=CARTESIAN_POINT ( 'NONE',  ( -0.3175540113612215221, -0.1078280746903921422, 1.953740157480315043 ) ) ;
#19737=ORIENTED_EDGE ( 'NONE', *, *, #27111, .T. ) ;
#19756=DIRECTION ( 'NONE',  ( 0.000000000000000000, 0.000000000000000000, -1.000000000000000000 ) ) ;
#19759=CIRCLE ( 'NONE', #16220, 0.3135473077061334268 ) ;
#19764=CARTESIAN_POINT ( 'NONE',  ( 0.3075317527319106903, -0.1775220790475473265, 1.953740157480315043 ) ) ;
#19772=CARTESIAN_POINT ( 'NONE',  ( -0.2762247810519161129, -0.4783323773986413729, 0.9202755905511811330 ) ) ;
#19775=FACE_OUTER_BOUND ( 'NONE', #26493, .T. ) ;
#19790=CARTESIAN_POINT ( 'NONE',  ( 0.3772436174784425389, -0.4300830224589218265, 0.9399606299212598381 ) ) ;
#19815=CARTESIAN_POINT ( 'NONE',  ( -0.4441657790094368230, 0.2564944395535841970, -1.550196850393700920 ) ) ;
#19822=CARTESIAN_POINT ( 'NONE',  ( -0.1188866373884876204, 0.4438564651657459503, -1.928289503579154740 ) ) ;
#19835=ADVANCED_FACE ( 'NONE', ( #16296 ), #13887, .T. ) ;
#19840=CARTESIAN_POINT ( 'NONE',  ( -0.4498374011142775575, 0.05926487674658489219, -1.934055118110236338 ) ) ;
#19844=EDGE_CURVE ( 'NONE', #25987, #14125, #13605, .T. ) ;
#19860=CARTESIAN_POINT ( 'NONE',  ( -0.5118110236220473341, 0.06699590632655400002, 1.766732283464566899 ) ) ;
#19861=CARTESIAN_POINT ( 'NONE',  ( 0.5118110236220472231, 0.03349795313260757468, 1.747047244094488194 ) ) ;
#19867=CARTESIAN_POINT ( 'NONE',  ( -0.3267488823401686893, 0.1886891683789005680, -3.100567304031762284 ) ) ;
#19873=CARTESIAN_POINT ( 'NONE',  ( 0.2041304421298423266, 0.2660793235464414264, 1.953740157480315043 ) ) ;
#19892=CARTESIAN_POINT ( 'NONE',  ( 0.2669480828848183052, -0.2341512108694381034, 1.953740157480315043 ) ) ;
#19910=CARTESIAN_POINT ( 'NONE',  ( 0.2442565704126269388, 0.4954197419817067960, 0.9399606299212598381 ) ) ;
#19926=CARTESIAN_POINT ( 'NONE',  ( -0.5526079293736928522, -0.1480156394741928838, 0.9399606299212598381 ) ) ;
#19939=ORIENTED_EDGE ( 'NONE', *, *, #20548, .T. ) ;
#19940=CARTESIAN_POINT ( 'NONE',  ( -0.4068916527368352520, 0.3122765577853303109, -1.550196850393700920 ) ) ;
#19949=CARTESIAN_POINT ( 'NONE',  ( 0.01298928997750990744, 0.3147564789080253278, -3.646005713789110203 ) ) ;
#19951=CARTESIAN_POINT ( 'NONE',  ( 0.1649135259639241124, 0.4856708409191630715, -1.550196850393700920 ) ) ;
#19954=CARTESIAN_POINT ( 'NONE',  ( 0.4438564651657541105, -0.1188866373884811950, -1.928289503579147857 ) ) ;
#19955=CARTESIAN_POINT ( 'NONE',  ( 0.1775991818008376133, 0.5230301363771421297, 0.9202755905511811330 ) ) ;
#19980=CARTESIAN_POINT ( 'NONE',  ( -0.1970998888482735634, -0.3995939286812472124, -1.934055118110236338 ) ) ;
#19981=CARTESIAN_POINT ( 'NONE',  ( 0.3765118517642104257, -0.02464264302293790732, -3.100567304031763172 ) ) ;
#19982=DIRECTION ( 'NONE',  ( 0.000000000000000000, 0.000000000000000000, -1.000000000000000000 ) ) ;
#19987=CARTESIAN_POINT ( 'NONE',  ( -0.4793172621399190425, -0.1288129352161815622, -1.569881889763780070 ) ) ;
#19996=CARTESIAN_POINT ( 'NONE',  ( -0.4954415918530867824, -0.1327036767659759697, 1.747047244094488194 ) ) ;
#20000=CARTESIAN_POINT ( 'NONE',  ( 0.3702005978258584573, 0.04877294052296160531, -3.115157480314960647 ) ) ;
#20005=CARTESIAN_POINT ( 'NONE',  ( -0.3324885138898231451, -0.04380447413659061678, 1.953740157480315043 ) ) ;
#20006=ORIENTED_EDGE ( 'NONE', *, *, #26211, .F. ) ;
#20009=EDGE_LOOP ( 'NONE', ( #1985, #23887, #19326, #11457 ) ) ;
#20016=CARTESIAN_POINT ( 'NONE',  ( -0.02063739440585312876, 0.1968503937007874127, -3.195955311827340051 ) ) ;
#20021=EDGE_CURVE ( 'NONE', #18631, #18101, #3410, .T. ) ;
#20023=CARTESIAN_POINT ( 'NONE',  ( -0.1570220809524473238, 0.3184841198566425446, 1.953740157480315043 ) ) ;
#20036=CARTESIAN_POINT ( 'NONE',  ( 0.1141156591737397391, -0.3362580771779613009, 1.953740157480315043 ) ) ;
#20045=CARTESIAN_POINT ( 'NONE',  ( 0.2860899518037664513, 0.4954156765914491944, 0.9399606299212598381 ) ) ;
#20047=DIRECTION ( 'NONE',  ( 1.000000000000000000, 0.000000000000000000, -0.000000000000000000 ) ) ;
#20058=CARTESIAN_POINT ( 'NONE',  ( 0.02190250779246093876, -0.3346456692913385988, 1.953740157480315043 ) ) ;
#20064=CARTESIAN_POINT ( 'NONE',  ( 0.2577577458591218673, -0.4472135058506043759, 1.766732283464566899 ) ) ;
#20065=AXIS2_PLACEMENT_3D ( 'NONE', #3758, #23422, #5899 ) ;
#20072=CARTESIAN_POINT ( 'NONE',  ( -0.3135473077061334268, 0.000000000000000000, 2.504921259842519898 ) ) ;
#20084=FACE_OUTER_BOUND ( 'NONE', #4107, .T. ) ;
#20085=CARTESIAN_POINT ( 'NONE',  ( 0.4270824798167666692, -0.2466292688015215839, -1.550196850393700920 ) ) ;
#20089=CARTESIAN_POINT ( 'NONE',  ( -0.3030032861724965554, -0.3454440660767394422, -1.928289503579165620 ) ) ;
#20109=CARTESIAN_POINT ( 'NONE',  ( 0.2761764805255614297, 0.3599896729929412120, -1.934055118110236338 ) ) ;
#20116=DIRECTION ( 'NONE',  ( -1.000000000000000000, 0.000000000000000000, 0.000000000000000000 ) ) ;
#20118=CARTESIAN_POINT ( 'NONE',  ( -0.04928467685644277035, -0.3740848232703729015, -3.100567304031765392 ) ) ;
#20132=CARTESIAN_POINT ( 'NONE',  ( 0.4600326175560603970, 0.2268096725222477072, 1.747047244094488194 ) ) ;
#20134=ORIENTED_EDGE ( 'NONE', *, *, #12525, .F. ) ;
#20135=ORIENTED_EDGE ( 'NONE', *, *, #21724, .T. ) ;
#20136=CARTESIAN_POINT ( 'NONE',  ( 0.3349073414797994475, -0.1651192144506243853, -3.115157480314960647 ) ) ;
#20157=CARTESIAN_POINT ( 'NONE',  ( -0.1685339107540412829, -0.2924088307484720706, 1.973425196850394192 ) ) ;
#20163=CARTESIAN_POINT ( 'NONE',  ( -0.5314960629921260393, 0.03478633594543736884, 1.747047244094488194 ) ) ;
#20164=ORIENTED_EDGE ( 'NONE', *, *, #19068, .F. ) ;
#20167=ORIENTED_EDGE ( 'NONE', *, *, #12888, .T. ) ;
#20174=CARTESIAN_POINT ( 'NONE',  ( 0.4423390553432540173, 0.2180862235769270852, -1.569881889763779625 ) ) ;
#20179=CARTESIAN_POINT ( 'NONE',  ( -0.1775991818008371415, -0.5230301363771194811, 0.9399606299212598381 ) ) ;
#20182=DIRECTION ( 'NONE',  ( 0.000000000000000000, 0.000000000000000000, 1.000000000000000000 ) ) ;
#20190=DIRECTION ( 'NONE',  ( 0.000000000000000000, 0.000000000000000000, -1.000000000000000000 ) ) ;
#20193=CARTESIAN_POINT ( 'NONE',  ( -0.1078280746903930304, -0.3175540113612211890, 1.953740157480315043 ) ) ;
#20210=CARTESIAN_POINT ( 'NONE',  ( -0.08600259748439401108, 0.1968503937007873850, -3.597797143241373785 ) ) ;
#20212=EDGE_CURVE ( 'NONE', #804, #12664, #12746, .T. ) ;
#20223=CARTESIAN_POINT ( 'NONE',  ( 0.3765118517642103146, 0.04928528614549709808, -3.100567304031763172 ) ) ;
#20227=CARTESIAN_POINT ( 'NONE',  ( -0.3175540113612294602, 0.1078280746904015375, 1.973425196850393970 ) ) ;
#20228=CARTESIAN_POINT ( 'NONE',  ( -0.4763861460130774939, -0.1275996891957774104, -1.550196850393700920 ) ) ;
#20231=CARTESIAN_POINT ( 'NONE',  ( 0.4382482975805169212, -0.3362148458988646338, 0.9202755905511811330 ) ) ;
#20235=CARTESIAN_POINT ( 'NONE',  ( 0.3765118517642104257, -2.263258471485603576E-17, -3.100567304031763172 ) ) ;
#20246=ORIENTED_EDGE ( 'NONE', *, *, #10729, .T. ) ;
#20247=CARTESIAN_POINT ( 'NONE',  ( 0.3429834333089943899, 0.09193786035240139598, 1.953740157480315043 ) ) ;
#20249=CARTESIAN_POINT ( 'NONE',  ( 0.2006393256663695779, -0.4069519308876702324, -1.934055118110236338 ) ) ;
#20252=CARTESIAN_POINT ( 'NONE',  ( 0.09334108100632415583, 0.3008230085310484858, -3.240743125436765126 ) ) ;
#20259=CIRCLE ( 'NONE', #8096, 0.3346456692913385988 ) ;
#20261=CARTESIAN_POINT ( 'NONE',  ( 0.02464264302293787262, 0.3765118517642104257, -3.100567304031763172 ) ) ;
#20273=CARTESIAN_POINT ( 'NONE',  ( 0.3121994997598087074, 0.4069448477555728250, 1.747047244094488194 ) ) ;
#20279=CARTESIAN_POINT ( 'NONE',  ( -0.09660931395005439848, 0.3606853515406323596, -3.115157480314960647 ) ) ;
#20280=ORIENTED_EDGE ( 'NONE', *, *, #9385, .T. ) ;
#20292=CARTESIAN_POINT ( 'NONE',  ( -0.3460635936744770880, 0.09269288654273796779, -3.115157480314960647 ) ) ;
#20296=DIRECTION ( 'NONE',  ( 1.000000000000000000, 0.000000000000000000, 0.000000000000000000 ) ) ;
#20300=DIRECTION ( 'NONE',  ( -1.000000000000000000, 0.000000000000000000, 0.000000000000000000 ) ) ;
#20304=CARTESIAN_POINT ( 'NONE',  ( -0.3520466617656973218, 0.04638120790932954290, 1.953740157480315043 ) ) ;
#20306=CIRCLE ( 'NONE', #23932, 0.5511811023268710086 ) ;
#20309=CARTESIAN_POINT ( 'NONE',  ( -0.4612490782034865955, 0.2663596103035612561, 1.747047244094488194 ) ) ;
#20310=CARTESIAN_POINT ( 'NONE',  ( -0.2268096725222462362, 0.4600326175560554565, 1.766732283464566899 ) ) ;
#20316=CARTESIAN_POINT ( 'NONE',  ( -0.2669917830071097953, -0.2341095169845849866, 1.953740157480314821 ) ) ;
#20322=CARTESIAN_POINT ( 'NONE',  ( 0.2180862235769582824, 0.4423390553432410832, -1.569881889763779625 ) ) ;
#20324=CARTESIAN_POINT ( 'NONE',  ( -0.2762247810519084523, -0.4783323773986298266, 0.9399606299212598381 ) ) ;
#20338=CARTESIAN_POINT ( 'NONE',  ( 0.3324885138898230341, -0.04380447413659129680, 1.953740157480315043 ) ) ;
#20340=B_SPLINE_CURVE_WITH_KNOTS ( 'NONE', 2,
 ( #26935, #24384, #1359 ),
 .UNSPECIFIED., .F., .F.,
 ( 3, 3 ),
 ( 0.000000000000000000, 1.000000000000000000 ),
 .UNSPECIFIED. ) ;
#20343=EDGE_CURVE ( 'NONE', #15069, #22294, #2960, .T. ) ;
#20344=CARTESIAN_POINT ( 'NONE',  ( -0.1477428134820414352, -0.4351030398461918081, -1.928289503579139641 ) ) ;
#20347=DIRECTION ( 'NONE',  ( -1.000000000000000000, 0.000000000000000000, 0.000000000000000000 ) ) ;
#20348=PLANE ( 'NONE',  #19148 ) ;
#20366=CARTESIAN_POINT ( 'NONE',  ( -0.08676778863011193332, -0.3239425792934405024, 1.973425196850393970 ) ) ;
#20367=CARTESIAN_POINT ( 'NONE',  ( -0.3252100150720236837, -0.3707612262533185321, -1.550196850393700920 ) ) ;
#20371=CARTESIAN_POINT ( 'NONE',  ( -0.5476281405333500718, 0.07214854559197644845, 0.9399606299212598381 ) ) ;
#20390=CARTESIAN_POINT ( 'NONE',  ( -0.2816986811832633553, 0.2161891097064990996, 1.953740157480315043 ) ) ;
#20394=CARTESIAN_POINT ( 'NONE',  ( -1.452994488188976472E-16, 0.5905905511811023745, -3.548228346456693050 ) ) ;
#20401=ORIENTED_EDGE ( 'NONE', *, *, #18180, .F. ) ;
#20405=CARTESIAN_POINT ( 'NONE',  ( -0.2938049579018679469, -0.3349573549949684259, -1.934055118110236338 ) ) ;
#20413=CARTESIAN_POINT ( 'NONE',  ( 0.4069448477555425714, 0.3121994997598541155, 1.747047244094488194 ) ) ;
#20419=CARTESIAN_POINT ( 'NONE',  ( 0.3267488823401797360, -0.1886891683788832486, -3.100567304031763172 ) ) ;
#20420=VERTEX_POINT ( 'NONE', #9317 ) ;
#20421=CARTESIAN_POINT ( 'NONE',  ( -0.4555658499976152354, -0.06001958459474936169, -1.928289503579151187 ) ) ;
#20426=CARTESIAN_POINT ( 'NONE',  ( -0.09842519685039370636, 0.5905905511811023745, -3.272637795275590733 ) ) ;
#20428=CARTESIAN_POINT ( 'NONE',  ( 0.2938049579018456314, -0.3349573549949907414, -1.934055118110236338 ) ) ;
#20430=ORIENTED_EDGE ( 'NONE', *, *, #25154, .T. ) ;
#20442=CARTESIAN_POINT ( 'NONE',  ( 0.1775730735577447927, -0.3074993854542728555, 1.953740157480315043 ) ) ;
#20451=CARTESIAN_POINT ( 'NONE',  ( -0.2663596103035690277, -0.4612490782034817105, 1.747047244094488194 ) ) ;
#20453=CARTESIAN_POINT ( 'NONE',  ( -0.3382184156732009339, -0.3855916753051547574, 1.766732283464566899 ) ) ;
#20459=CARTESIAN_POINT ( 'NONE',  ( -0.2712027394948746117, 0.3535065162672773043, -1.934055118110236338 ) ) ;
#20461=CARTESIAN_POINT ( 'NONE',  ( 0.3324885138898233672, 0.04380447413659172701, 1.973425196850393970 ) ) ;
#20462=ORIENTED_EDGE ( 'NONE', *, *, #17978, .F. ) ;
#20465=CARTESIAN_POINT ( 'NONE',  ( 0.4763861460130341396, -0.1275996891957698887, -1.569881889763779625 ) ) ;
#20477=CARTESIAN_POINT ( 'NONE',  ( -0.2211428102655801364, -0.2521176338356625468, 1.953740157480315043 ) ) ;
#20484=DIRECTION ( 'NONE',  ( 0.000000000000000000, 0.000000000000000000, 1.000000000000000000 ) ) ;
#20495=CARTESIAN_POINT ( 'NONE',  ( -0.03965503742771055162, 0.1968503937007873850, -3.617030424444270587 ) ) ;
#20511=CARTESIAN_POINT ( 'NONE',  ( 0.09333873788075952582, 0.3008237467743239413, -3.580130230456529894 ) ) ;
#20512=CARTESIAN_POINT ( 'NONE',  ( -0.4600326175569940945, -0.2268096725200247077, -1.550196850393700920 ) ) ;
#20514=CARTESIAN_POINT ( 'NONE',  ( 0.4382482975805264136, 0.3362148458988503674, 0.9202755905511811330 ) ) ;
#20521=CARTESIAN_POINT ( 'NONE',  ( -0.4270824798167633385, 0.2466292688015202517, -1.569881889763779625 ) ) ;
#20524=CARTESIAN_POINT ( 'NONE',  ( -0.1711665596939558887, 0.5043892184458266259, 1.747047244094488194 ) ) ;
#20525=PRESENTATION_STYLE_ASSIGNMENT (( #15604 ) ) ;
#20537=CARTESIAN_POINT ( 'NONE',  ( -0.2006393256663304703, -0.4069519308876202168, -1.934055118110236338 ) ) ;
#20547=CARTESIAN_POINT ( 'NONE',  ( -0.2836590635674511307, -0.2488091035917043836, -3.100567304031761395 ) ) ;
#20548=EDGE_CURVE ( 'NONE', #15380, #10350, #12444, .T. ) ;
#20549=CARTESIAN_POINT ( 'NONE',  ( 0.1791101711252919282, -0.3102827802123563905, -3.115157480314960203 ) ) ;
#20551=ORIENTED_EDGE ( 'NONE', *, *, #18603, .T. ) ;
#20552=CARTESIAN_POINT ( 'NONE',  ( -0.4296318976990082805, 0.1458850421962457622, -1.934055118110236338 ) ) ;
#20554=CARTESIAN_POINT ( 'NONE',  ( -0.4498374011143459472, -0.05926487674658267174, -1.934055118110236338 ) ) ;
#20559=CARTESIAN_POINT ( 'NONE',  ( 0.5118110236220472231, -0.03349795313260760937, 1.747047244094488194 ) ) ;
#20566=CARTESIAN_POINT ( 'NONE',  ( -0.09762295995069376897, -0.3644697409450285974, -3.100567304031760951 ) ) ;
#20581=CARTESIAN_POINT ( 'NONE',  ( 0.1151913129404385921, 0.3392387706403768299, -3.115157480314960647 ) ) ;
#20587=EDGE_CURVE ( 'NONE', #7118, #22055, #5812, .T. ) ;
#20595=CARTESIAN_POINT ( 'NONE',  ( 0.5118110236220472231, -0.03349795313260760937, 1.747047244094488194 ) ) ;
#20596=CARTESIAN_POINT ( 'NONE',  ( -0.2268096725222457366, -0.4600326175560556230, 1.766732283464566899 ) ) ;
#20599=CARTESIAN_POINT ( 'NONE',  ( -0.3460635936744770880, 0.09269288654273796779, -3.115157480314960647 ) ) ;
#20607=CARTESIAN_POINT ( 'NONE',  ( 0.3001918266902277588, 0.3912931228432131592, -1.569881889763779625 ) ) ;
#20637=CARTESIAN_POINT ( 'NONE',  ( 0.04956879678462433603, 0.2165354330708661457, -3.634230943941095138 ) ) ;
#20647=ORIENTED_EDGE ( 'NONE', *, *, #21256, .F. ) ;
#20651=CARTESIAN_POINT ( 'NONE',  ( -0.3387265385688507657, 0.4407612517155324872, 0.9202755905511812440 ) ) ;
#20653=CARTESIAN_POINT ( 'NONE',  ( 0.2762247810519017355, -0.4783323773986510319, 0.9202755905511811330 ) ) ;
#20659=CARTESIAN_POINT ( 'NONE',  ( 0.4921259842519685179, 0.03220957031754003580, -1.569881889763779625 ) ) ;
#20666=CARTESIAN_POINT ( 'NONE',  ( 0.5905511811023621549, 0.000000000000000000, 0.9399606299212598381 ) ) ;
#20672=CARTESIAN_POINT ( 'NONE',  ( -0.3520570504767979725, 0.04632170870437362503, 1.953740157480315043 ) ) ;
#20676=CARTESIAN_POINT ( 'NONE',  ( -0.02563572372337621225, 0.3139795790815559373, -3.177391021203589183 ) ) ;
#20679=EDGE_LOOP ( 'NONE', ( #20551, #16120, #6197, #16963 ) ) ;
#20687=CARTESIAN_POINT ( 'NONE',  ( 0.02909913904662007542, 0.4446020952038907681, -1.934055118110236338 ) ) ;
#20696=CARTESIAN_POINT ( 'NONE',  ( -0.4777261797697572310, -0.2355331214654124150, 1.747047244094488194 ) ) ;
#20702=CARTESIAN_POINT ( 'NONE',  ( -0.3765118517642104257, 0.000000000000000000, -3.100567304031763172 ) ) ;
#20709=DIRECTION ( 'NONE',  ( 0.000000000000000000, -0.000000000000000000, -1.000000000000000000 ) ) ;
#20712=CARTESIAN_POINT ( 'NONE',  ( 0.1970259548082107792, -0.3996230174612653285, -1.934055118110236338 ) ) ;
#20716=CARTESIAN_POINT ( 'NONE',  ( 0.1584254766472199816, -0.3213305936751578717, -3.115157480314960647 ) ) ;
#20718=CARTESIAN_POINT ( 'NONE',  ( 0.1685339107540412273, 0.2924088307484721816, 1.973425196850394192 ) ) ;
#20725=CARTESIAN_POINT ( 'NONE',  ( 0.3520466617656973218, -0.04638120790932973719, 1.953740157480315043 ) ) ;
#20728=CARTESIAN_POINT ( 'NONE',  ( -0.2860009521618332440, 0.4954734376824599384, 0.9399606299212600602 ) ) ;
#20731=DIRECTION ( 'NONE',  ( 0.000000000000000000, 0.000000000000000000, 1.000000000000000000 ) ) ;
#20736=CARTESIAN_POINT ( 'NONE',  ( 0.5314960629921260393, 0.000000000000000000, 1.747047244094488194 ) ) ;
#20739=CARTESIAN_POINT ( 'NONE',  ( 0.1327036767659575123, -0.4954415918530866714, 1.766732283464566899 ) ) ;
#20749=CARTESIAN_POINT ( 'NONE',  ( -0.4921259842519685179, 0.000000000000000000, -1.569881889763779625 ) ) ;
#20750=ORIENTED_EDGE ( 'NONE', *, *, #21159, .F. ) ;
#20766=CARTESIAN_POINT ( 'NONE',  ( -0.06441914069860964209, 0.4921259842519686845, -1.569881889763779625 ) ) ;
#20767=FACE_BOUND ( 'NONE', #25715, .T. ) ;
#20774=ADVANCED_FACE ( 'NONE', ( #11807 ), #26929, .F. ) ;
#20781=ORIENTED_EDGE ( 'NONE', *, *, #8518, .F. ) ;
#20783=DIRECTION ( 'NONE',  ( 0.000000000000000000, 0.000000000000000000, -1.000000000000000000 ) ) ;
#20790=CARTESIAN_POINT ( 'NONE',  ( 0.2775852647713619725, 0.4816145447621894005, 0.9202755905511812440 ) ) ;
#20793=CARTESIAN_POINT ( 'NONE',  ( 0.5511811023622047445, 0.03607471876262480226, 0.9202755905511811330 ) ) ;
#20800=CARTESIAN_POINT ( 'NONE',  ( -0.02576258753921337533, 0.2165354330708661457, -3.176774343053047733 ) ) ;
#20812=CARTESIAN_POINT ( 'NONE',  ( -0.09842519685039377575, 0.2991866959364320455, -3.266083869132035744 ) ) ;
#20822=CARTESIAN_POINT ( 'NONE',  ( 0.1152775731717068236, 0.4303822302054135518, -1.934055118110236338 ) ) ;
#20835=CARTESIAN_POINT ( 'NONE',  ( -0.1886891683788859964, 0.3267488823401775155, -3.100567304031764948 ) ) ;
#20840=CARTESIAN_POINT ( 'NONE',  ( -0.04638120790932972332, -0.3520466617656973218, 1.953740157480315043 ) ) ;
#20845=CARTESIAN_POINT ( 'NONE',  ( -0.4954156765914823346, 0.2860899518036844058, 0.9399606299212598381 ) ) ;
#20847=EDGE_LOOP ( 'NONE', ( #24612, #25532 ) ) ;
#20854=CARTESIAN_POINT ( 'NONE',  ( -0.3460635936744816399, -0.09269288654274071559, -3.115157480314960647 ) ) ;
#20866=CIRCLE ( 'NONE', #6904, 0.3937007874015748254 ) ;
#20869=CARTESIAN_POINT ( 'NONE',  ( 0.5314960629921260393, -0.03478633594540021801, 1.747047244094488194 ) ) ;
#20871=CARTESIAN_POINT ( 'NONE',  ( -0.09842519685039366473, 0.1968503937007873850, -3.272637795275590733 ) ) ;
#20872=CARTESIAN_POINT ( 'NONE',  ( 0.5118110236220472231, 0.000000000000000000, 1.747047244094488194 ) ) ;
#20877=CARTESIAN_POINT ( 'NONE',  ( -0.3574975638436101444, 0.000000000000000000, -3.115157480314960647 ) ) ;
#20881=DIRECTION ( 'NONE',  ( 0.000000000000000000, 0.000000000000000000, 1.000000000000000000 ) ) ;
#20885=CARTESIAN_POINT ( 'NONE',  ( 0.3707612262533330205, 0.3252100150720381722, -1.550196850393700920 ) ) ;
#20915=VECTOR ( 'NONE', #24531, 39.37007874015748143 ) ;
#20933=CARTESIAN_POINT ( 'NONE',  ( 0.2521176338356670432, 0.2211428102655656758, 1.953740157480315043 ) ) ;
#20936=CARTESIAN_POINT ( 'NONE',  ( -0.4382482975804890546, -0.3362148458988509225, 0.9399606299212598381 ) ) ;
#20951=AXIS2_PLACEMENT_3D ( 'NONE', #26251, #8746, #11279 ) ;
#20967=CARTESIAN_POINT ( 'NONE',  ( 0.03220957031753916844, -0.4921259842519686289, -1.569881889763779625 ) ) ;
#20970=CARTESIAN_POINT ( 'NONE',  ( 0.05819755867304853003, -0.4417361510194242613, -1.934055118110236338 ) ) ;
#20976=CARTESIAN_POINT ( 'NONE',  ( 0.5314960629921260393, 0.03478633594540018331, 1.747047244094488194 ) ) ;
#20981=CARTESIAN_POINT ( 'NONE',  ( 0.3350145293470547236, 0.2937497900413817975, -1.934055118110236338 ) ) ;
#20983=CARTESIAN_POINT ( 'NONE',  ( 0.1775730735577439323, 0.3074993854542599769, 1.953740157480315043 ) ) ;
#20988=CARTESIAN_POINT ( 'NONE',  ( 0.4954156765914486393, 0.2860899518037346989, 0.9399606299212598381 ) ) ;
#20990=VERTEX_POINT ( 'NONE', #17582 ) ;
#20996=CARTESIAN_POINT ( 'NONE',  ( 0.3551931031211519874, -0.04679574315772458415, -3.115157480314960647 ) ) ;
#20998=CARTESIAN_POINT ( 'NONE',  ( 0.4816145447621895115, -0.2775852647713619170, 0.9202755905511811330 ) ) ;
#21007=CARTESIAN_POINT ( 'NONE',  ( 0.4538422614035440561, 0.3483115186079798753, 0.9399606299212601712 ) ) ;
#21011=CARTESIAN_POINT ( 'NONE',  ( -0.4600326175560542907, 0.2268096725222489285, 1.766732283464566899 ) ) ;
#21016=ORIENTED_EDGE ( 'NONE', *, *, #4364, .F. ) ;
#21020=FACE_OUTER_BOUND ( 'NONE', #22154, .T. ) ;
#21022=CARTESIAN_POINT ( 'NONE',  ( -0.3175540113612294602, 0.1078280746904015375, 1.973425196850393970 ) ) ;
#21024=CARTESIAN_POINT ( 'NONE',  ( -0.4889536969035060410, 0.06441834428466772233, -1.550196850393700920 ) ) ;
#21027=ORIENTED_EDGE ( 'NONE', *, *, #20587, .T. ) ;
#21030=LINE ( 'NONE', #18616, #3590 ) ;
#21045=LINE ( 'NONE', #10446, #22196 ) ;
#21057=CARTESIAN_POINT ( 'NONE',  ( 0.1429116519061275903, 0.5335524835332325910, 0.9202755905511811330 ) ) ;
#21065=ORIENTED_EDGE ( 'NONE', *, *, #25880, .T. ) ;
#21066=CARTESIAN_POINT ( 'NONE',  ( -0.1482986320106466638, 0.3007905576423924310, 1.953740157480315043 ) ) ;
#21067=CARTESIAN_POINT ( 'NONE',  ( 0.4441657790094322711, 0.2564944395535476707, -1.550196850393700920 ) ) ;
#21070=CARTESIAN_POINT ( 'NONE',  ( 0.07214854559198032036, -0.5476281405333571772, 0.9399606299212598381 ) ) ;
#21079=CARTESIAN_POINT ( 'NONE',  ( -0.3242876858378660465, 0.4225410690761917665, 1.747047244094487972 ) ) ;
#21083=CARTESIAN_POINT ( 'NONE',  ( 0.3855916753034687172, 0.3382184156749162285, -1.550196850393700920 ) ) ;
#21089=EDGE_LOOP ( 'NONE', ( #24772, #5619, #7285, #25943 ) ) ;
#21098=AXIS2_PLACEMENT_3D ( 'NONE', #7406, #19982, #13476 ) ;
#21107=CARTESIAN_POINT ( 'NONE',  ( -0.09275304139133716541, -0.3460530745557874321, -3.115157480314960647 ) ) ;
#21109=CARTESIAN_POINT ( 'NONE',  ( 0.02963280468032034737, -0.4527559054764770385, -1.934055118110236338 ) ) ;
#21111=CARTESIAN_POINT ( 'NONE',  ( -0.3645739570812708275, 0.2796934465393700053, -1.928289503579159625 ) ) ;
#21117=CARTESIAN_POINT ( 'NONE',  ( 0.1712563538833041243, 0.5043504886477225835, 1.747047244094488194 ) ) ;
#21125=CARTESIAN_POINT ( 'NONE',  ( -0.02917857698688259421, 0.4446006764000811629, -1.934055118110236338 ) ) ;
#21127=CARTESIAN_POINT ( 'NONE',  ( 0.3074993854542699689, 0.1775730735577541186, 1.953740157480315043 ) ) ;
#21137=CARTESIAN_POINT ( 'NONE',  ( -0.2362439534887390002, -0.2693339498142257038, -3.115157480314960647 ) ) ;
#21138=CARTESIAN_POINT ( 'NONE',  ( -0.4816145447621893450, -0.2775852647713621946, 0.9202755905511812440 ) ) ;
#21141=DIRECTION ( 'NONE',  ( -0.000000000000000000, -0.000000000000000000, 1.000000000000000000 ) ) ;
#21148=CARTESIAN_POINT ( 'NONE',  ( 0.4301570366551352165, 0.3771675965699478050, 0.9399606299212600602 ) ) ;
#21150=CARTESIAN_POINT ( 'NONE',  ( 0.5314960629921260393, 0.000000000000000000, 1.747047244094488194 ) ) ;
#21153=CARTESIAN_POINT ( 'NONE',  ( 0.2355331214654088623, -0.4777261797697378021, 1.747047244094488194 ) ) ;
#21159=EDGE_CURVE ( 'NONE', #1064, #14125, #22990, .T. ) ;
#21162=CARTESIAN_POINT ( 'NONE',  ( 0.3392387706403792169, -0.1151913129404410208, -3.115157480314960647 ) ) ;
#21164=CARTESIAN_POINT ( 'NONE',  ( 0.4006498629591503380, -0.2309201403895325411, -1.928289503579156294 ) ) ;
#21166=CARTESIAN_POINT ( 'NONE',  ( 0.08676778863010879694, -0.3239425792934411685, 1.973425196850393970 ) ) ;
#21169=CARTESIAN_POINT ( 'NONE',  ( -0.4669911931914605407, 0.1585706980422390278, -1.550196850393700920 ) ) ;
#21181=AXIS2_PLACEMENT_3D ( 'NONE', #4521, #17506, #26126 ) ;
#21191=CARTESIAN_POINT ( 'NONE',  ( 0.4793172621399192090, 0.1288129352161812569, -1.569881889763779625 ) ) ;
#21201=AXIS2_PLACEMENT_3D ( 'NONE', #27777, #27356, #2054 ) ;
#21205=CARTESIAN_POINT ( 'NONE',  ( 0.3642352168757561071, 0.4152525734086270348, 0.9202755905511811330 ) ) ;
#21212=CARTESIAN_POINT ( 'NONE',  ( -0.5085287184740916455, -0.06690297524250585215, -1.550196850393700920 ) ) ;
#21216=ORIENTED_EDGE ( 'NONE', *, *, #9385, .F. ) ;
#21218=CARTESIAN_POINT ( 'NONE',  ( 0.3239425792934409465, -0.08676778863010950471, 1.973425196850393970 ) ) ;
#21223=CARTESIAN_POINT ( 'NONE',  ( 0.2762247810519068980, 0.4783323773986306038, 0.9399606299212598381 ) ) ;
#21226=FACE_OUTER_BOUND ( 'NONE', #8249, .T. ) ;
#21233=CARTESIAN_POINT ( 'NONE',  ( -0.2564944395535840860, 0.4441657790094369895, -1.550196850393700920 ) ) ;
#21234=CARTESIAN_POINT ( 'NONE',  ( -0.4954734376818675790, -0.2860009521627228657, 0.9399606299212597271 ) ) ;
#21237=CARTESIAN_POINT ( 'NONE',  ( -0.4004922687717342167, -0.3511586785142652989, 1.747047244094487972 ) ) ;
#21243=CARTESIAN_POINT ( 'NONE',  ( -0.08582064676143620618, 0.3030881253039517387, -3.222721154529648135 ) ) ;
#21253=CARTESIAN_POINT ( 'NONE',  ( -0.2796934465393912106, 0.3645739570812651653, -1.928289503579152742 ) ) ;
#21254=CARTESIAN_POINT ( 'NONE',  ( 0.4585215200179055817, -0.03001016326913584151, -1.928289503579156516 ) ) ;
#21256=EDGE_CURVE ( 'NONE', #10004, #25, #349, .T. ) ;
#21263=CARTESIAN_POINT ( 'NONE',  ( 0.2663596103035382745, -0.4612490782035122416, 1.747047244094488194 ) ) ;
#21274=CARTESIAN_POINT ( 'NONE',  ( -0.3184841198566448206, 0.1570220809524502381, 1.953740157480315043 ) ) ;
#21275=VERTEX_POINT ( 'NONE', #21658 ) ;
#21284=CARTESIAN_POINT ( 'NONE',  ( 0.1867299569291587802, -0.3233561589689049609, -3.115157480314960647 ) ) ;
#21291=CARTESIAN_POINT ( 'NONE',  ( 0.4921259842519685179, -0.06441914069860961434, -1.569881889763779848 ) ) ;
#21297=CARTESIAN_POINT ( 'NONE',  ( 0.09842519685039355370, 0.2165354330708661457, -3.548228346456693050 ) ) ;
#21298=CARTESIAN_POINT ( 'NONE',  ( -0.4856708409200654608, 0.1649135259617025839, 1.766732283464566899 ) ) ;
#21303=CARTESIAN_POINT ( 'NONE',  ( -0.2842490391651530390, -0.2180698645301770988, -3.115157480314960647 ) ) ;
#21305=CARTESIAN_POINT ( 'NONE',  ( 0.4585215200179056372, -0.06002032661671170138, -1.928289503579156516 ) ) ;
#21308=CARTESIAN_POINT ( 'NONE',  ( -0.3346456692913385988, 0.02190250779246044610, 1.973425196850393970 ) ) ;
#21312=CARTESIAN_POINT ( 'NONE',  ( 0.2180862235769585322, 0.4423390553432415273, -1.550196850393700920 ) ) ;
#21320=CARTESIAN_POINT ( 'NONE',  ( -0.04992658653707177097, 0.3112137629952766438, -3.634044155725667302 ) ) ;
#21328=DIRECTION ( 'NONE',  ( 0.000000000000000000, 0.000000000000000000, 1.000000000000000000 ) ) ;
#21338=CARTESIAN_POINT ( 'NONE',  ( -0.03965503742771017692, 0.1968503937007873850, -3.203835717288081142 ) ) ;
#21345=CARTESIAN_POINT ( 'NONE',  ( 0.03607471876262465654, 0.5511811023622047445, 0.9202755905511811330 ) ) ;
#21357=VERTEX_POINT ( 'NONE', #22621 ) ;
#21363=CARTESIAN_POINT ( 'NONE',  ( 0.4783323773986625782, 0.2762247810518427271, 0.9399606299212598381 ) ) ;
#21366=CARTESIAN_POINT ( 'NONE',  ( -0.04673614183172691838, 0.3552064049866300866, -3.115157480314961091 ) ) ;
#21371=APPLICATION_CONTEXT ( 'automotive_design' ) ;
#21373=CARTESIAN_POINT ( 'NONE',  ( -0.3382184156749268311, 0.3855916753034290823, -1.550196850393700920 ) ) ;
#21377=CARTESIAN_POINT ( 'NONE',  ( -0.1327957795767781002, 0.4954247181592900118, -1.550196850393701364 ) ) ;
#21392=CARTESIAN_POINT ( 'NONE',  ( -0.4763861460130593972, 0.1275996891957734969, -1.550196850393700920 ) ) ;
#21393=CARTESIAN_POINT ( 'NONE',  ( 0.4498374011143674855, 0.05926487674658936083, -1.934055118110236338 ) ) ;
#21394=AXIS2_PLACEMENT_3D ( 'NONE', #2002, #25881, #21644 ) ;
#21399=CARTESIAN_POINT ( 'NONE',  ( 0.3346456692913385988, 4.098227477461614641E-17, 2.426181102355854158 ) ) ;
#21400=CARTESIAN_POINT ( 'NONE',  ( 0.5144970376935932288, -0.1378076643338853879, 1.747047244094488194 ) ) ;
#21405=AXIS2_PLACEMENT_3D ( 'NONE', #2767, #15785, #26372 ) ;
#21407=CARTESIAN_POINT ( 'NONE',  ( 0.1431838228103888555, 0.4219236230596360993, -1.934055118110237004 ) ) ;
#21410=CARTESIAN_POINT ( 'NONE',  ( -0.2669480828848092013, 0.2341512108694271399, 1.953740157480315043 ) ) ;
#21414=CARTESIAN_POINT ( 'NONE',  ( -0.1480156394741835579, -0.5526079293737254927, 0.9399606299212598381 ) ) ;
#21422=CARTESIAN_POINT ( 'NONE',  ( 0.1651192144506304360, -0.3349073414798397486, -3.115157480314960647 ) ) ;
#21427=CARTESIAN_POINT ( 'NONE',  ( 0.3024344094364739832, -0.3935368318888683437, -1.569881889763779625 ) ) ;
#21434=CARTESIAN_POINT ( 'NONE',  ( 0.3512268162760113777, -0.4004221243553278131, 1.747047244094488194 ) ) ;
#21436=CARTESIAN_POINT ( 'NONE',  ( -0.3382184156732009339, -0.3855916753051547574, 1.766732283464566899 ) ) ;
#21437=CARTESIAN_POINT ( 'NONE',  ( -0.4441657790107820802, -0.2564944395515947884, 1.747047244094488194 ) ) ;
#21444=CARTESIAN_POINT ( 'NONE',  ( -0.3535721684717625934, 0.1200583359873131500, -3.115157480314960647 ) ) ;
#21451=CARTESIAN_POINT ( 'NONE',  ( -0.3239425792934402248, -0.08676778863011362641, 1.973425196850393970 ) ) ;
#21455=CARTESIAN_POINT ( 'NONE',  ( 0.06441834428466734763, 0.4889536969035060965, -1.550196850393700920 ) ) ;
#21470=CARTESIAN_POINT ( 'NONE',  ( 0.2309201403895324856, 0.4006498629591504490, -1.928289503579156516 ) ) ;
#21478=CARTESIAN_POINT ( 'NONE',  ( -2.685748425196850164E-17, 0.000000000000000000, -3.745078740157480546 ) ) ;
#21484=CARTESIAN_POINT ( 'NONE',  ( -0.5511811023622048555, 0.000000000000000000, 0.9399606299212598381 ) ) ;
#21495=ORIENTED_EDGE ( 'NONE', *, *, #2298, .F. ) ;
#21497=CARTESIAN_POINT ( 'NONE',  ( -0.09842519685039366473, 0.1968503937007873850, -3.272637795275590733 ) ) ;
#21503=CARTESIAN_POINT ( 'NONE',  ( -0.2860899518037490763, 0.4954156765914824456, 0.9399606299212598381 ) ) ;
#21508=CARTESIAN_POINT ( 'NONE',  ( -0.4527559054764770385, -0.02963280468031422032, -1.934055118110236338 ) ) ;
#21515=CARTESIAN_POINT ( 'NONE',  ( 0.4069448477569521661, 0.3121994997578569353, -1.550196850393700920 ) ) ;
#21518=CARTESIAN_POINT ( 'NONE',  ( 0.5314960629921261503, -0.03489125111630842629, 1.747047244094488416 ) ) ;
#21530=CARTESIAN_POINT ( 'NONE',  ( -0.1275996891957733581, -0.4763861460130334735, -1.569881889763779625 ) ) ;
#21531=CARTESIAN_POINT ( 'NONE',  ( 0.02963280468032102044, 0.4527559054764770385, -1.934055118110236338 ) ) ;
#21538=CARTESIAN_POINT ( 'NONE',  ( -0.09842519685039370636, 0.2165354330708661457, -3.272637795275590733 ) ) ;
#21540=CARTESIAN_POINT ( 'NONE',  ( -0.3362580771780888655, -0.1141156591734552583, 1.953740157480314599 ) ) ;
#21543=CARTESIAN_POINT ( 'NONE',  ( 0.2937477835497820378, 0.3350125228554541312, -1.934055118110236560 ) ) ;
#21546=CARTESIAN_POINT ( 'NONE',  ( -0.3929158813954827245, 0.2268989272876178465, -1.934055118110236338 ) ) ;
#21551=CARTESIAN_POINT ( 'NONE',  ( 0.2272836761397793726, 0.2962590301041582164, -3.115157480314960647 ) ) ;
#21569=ADVANCED_FACE ( 'NONE', ( #19775 ), #25727, .T. ) ;
#21571=CARTESIAN_POINT ( 'NONE',  ( 0.5118110236220471121, 0.06699590632655406941, 1.766732283464567121 ) ) ;
#21573=CARTESIAN_POINT ( 'NONE',  ( 0.06699507805370044644, -0.5085118447801416641, 1.766732283464566899 ) ) ;
#21574=CARTESIAN_POINT ( 'NONE',  ( -0.3121994997598253052, -0.4069448477556119048, 1.747047244094488194 ) ) ;
#21579=CARTESIAN_POINT ( 'NONE',  ( -0.2693339498142344746, -0.2362439534887506021, -3.115157480314960647 ) ) ;
#21584=CARTESIAN_POINT ( 'NONE',  ( -0.02190250779246035590, 0.3346456692913385988, 1.953740157480315043 ) ) ;
#21597=CARTESIAN_POINT ( 'NONE',  ( -2.685748425196850164E-17, 0.000000000000000000, -3.745078740157480546 ) ) ;
#21599=CARTESIAN_POINT ( 'NONE',  ( -0.5043865966253989752, 0.1711654736997713921, 1.747047244094488416 ) ) ;
#21608=CARTESIAN_POINT ( 'NONE',  ( -0.2817828961649163078, 0.3666644560843324019, -1.928289503579156294 ) ) ;
#21621=VERTEX_POINT ( 'NONE', #27852 ) ;
#21622=CARTESIAN_POINT ( 'NONE',  ( -0.5511811023622047445, -0.03607471876259067678, 0.9202755905511811330 ) ) ;
#21635=FACE_OUTER_BOUND ( 'NONE', #17350, .T. ) ;
#21643=CARTESIAN_POINT ( 'NONE',  ( 0.4539000224941021067, -0.3482225189666773302, 0.9399606299212598381 ) ) ;
#21644=DIRECTION ( 'NONE',  ( 0.000000000000000000, 0.000000000000000000, -1.000000000000000000 ) ) ;
#21646=CARTESIAN_POINT ( 'NONE',  ( -0.1584813376850940092, 0.3213059197594776428, -3.115157480314961980 ) ) ;
#21652=CARTESIAN_POINT ( 'NONE',  ( 0.06699507805605696420, 0.5085118447796661556, -1.550196850393700920 ) ) ;
#21658=CARTESIAN_POINT ( 'NONE',  ( -0.5118110236220472231, 3.201384367575308305E-17, 1.766732283464566899 ) ) ;
#21661=CONICAL_SURFACE ( 'NONE', #21201, 0.3135473077061334268, 0.2617993874999994808 ) ;
#21669=CARTESIAN_POINT ( 'NONE',  ( 0.4351030398461776527, -0.1477428134820240602, -1.928289503579159625 ) ) ;
#21670=CARTESIAN_POINT ( 'NONE',  ( 0.4351030398461604998, 0.1477428134820414352, -1.928289503579168951 ) ) ;
#21674=LINE ( 'NONE', #17424, #11241 ) ;
#21679=CARTESIAN_POINT ( 'NONE',  ( 0.3512268162760113777, -0.4004221243553278131, 1.747047244094488194 ) ) ;
#21680=PLANE ( 'NONE',  #4832 ) ;
#21690=VERTEX_POINT ( 'NONE', #16097 ) ;
#21694=CARTESIAN_POINT ( 'NONE',  ( 0.4954156765914815574, -0.2860899518037339773, 0.9399606299212598381 ) ) ;
#21697=CARTESIAN_POINT ( 'NONE',  ( 0.4417502570507448323, -0.05811937031602956022, -1.934055118110236116 ) ) ;
#21699=CARTESIAN_POINT ( 'NONE',  ( 0.02438677169350735724, -0.3726024258163779246, -3.115157480314960647 ) ) ;
#21711=CARTESIAN_POINT ( 'NONE',  ( -0.1339654526248285626, 0.4984899526255159308, 1.766732283464566899 ) ) ;
#21712=CARTESIAN_POINT ( 'NONE',  ( -0.03349795313264326141, 0.5118110236220472231, 1.766732283464566899 ) ) ;
#21713=CARTESIAN_POINT ( 'NONE',  ( -0.1327036767659760530, 0.4954415918530867269, 1.747047244094488194 ) ) ;
#21717=CARTESIAN_POINT ( 'NONE',  ( 0.1151913129404419367, -0.3392387706403586223, -3.115157480314960647 ) ) ;
#21718=EDGE_LOOP ( 'NONE', ( #21065, #2391 ) ) ;
#21722=CARTESIAN_POINT ( 'NONE',  ( 0.3007905576423755556, -0.1482986320106471911, 1.953740157480315043 ) ) ;
#21724=EDGE_CURVE ( 'NONE', #16188, #285, #4574, .T. ) ;
#21735=ADVANCED_FACE ( 'NONE', ( #13545 ), #6386, .T. ) ;
#21736=CARTESIAN_POINT ( 'NONE',  ( -2.685748425196850164E-17, 0.000000000000000000, -3.115157480314960647 ) ) ;
#21739=ORIENTED_EDGE ( 'NONE', *, *, #17953, .T. ) ;
#21749=FACE_OUTER_BOUND ( 'NONE', #9862, .T. ) ;
#21752=CARTESIAN_POINT ( 'NONE',  ( 0.3520570504767833175, -0.04632170870443329952, 1.953740157480315487 ) ) ;
#21755=EDGE_CURVE ( 'NONE', #3938, #21621, #5208, .T. ) ;
#21761=CARTESIAN_POINT ( 'NONE',  ( 0.03607471876262385857, -0.5511811023622048555, 0.9202755905511811330 ) ) ;
#21776=CARTESIAN_POINT ( 'NONE',  ( 0.5526079293737076181, -0.1480156394741905801, 0.9399606299212598381 ) ) ;
#21801=CARTESIAN_POINT ( 'NONE',  ( 0.08582157620924656116, 0.3030878557544539054, -3.598143271073415139 ) ) ;
#21802=CARTESIAN_POINT ( 'NONE',  ( -0.2180862235769562008, -0.4423390553432419714, -1.569881889763779625 ) ) ;
#21804=CARTESIAN_POINT ( 'NONE',  ( 0.4585215200179055817, -0.03001016326913584151, -1.928289503579156516 ) ) ;
#21826=CARTESIAN_POINT ( 'NONE',  ( -0.4417361510194242613, -0.05819755867303597063, -1.934055118110236338 ) ) ;
#21833=CARTESIAN_POINT ( 'NONE',  ( 0.2937497900415150243, -0.3350145293469216079, -1.934055118110236560 ) ) ;
#21834=CARTESIAN_POINT ( 'NONE',  ( -0.2462256503455939050, 0.2807137536170327685, -3.115157480314960647 ) ) ;
#21837=CONICAL_SURFACE ( 'NONE', #6517, 0.3726024258163779246, 0.2617993874999969828 ) ;
#21851=CARTESIAN_POINT ( 'NONE',  ( 0.3606853515406215904, 0.09660931395005435685, -3.115157480314960647 ) ) ;
#21857=CARTESIAN_POINT ( 'NONE',  ( -0.1078280746903930304, -0.3175540113612211890, 1.953740157480315043 ) ) ;
#21864=ORIENTED_EDGE ( 'NONE', *, *, #14504, .T. ) ;
#21875=LINE ( 'NONE', #25839, #3773 ) ;
#21890=CARTESIAN_POINT ( 'NONE',  ( 0.3543307086614173040, -0.02325840746512450319, 1.953740157480314821 ) ) ;
#21892=ORIENTED_EDGE ( 'NONE', *, *, #3729, .T. ) ;
#21893=CARTESIAN_POINT ( 'NONE',  ( -0.3765118517642104257, 2.305470170520414967E-17, -3.100567304031763172 ) ) ;
#21894=CARTESIAN_POINT ( 'NONE',  ( -0.4889536969035324643, 0.06441834428466573781, -1.569881889763779625 ) ) ;
#21898=CARTESIAN_POINT ( 'NONE',  ( -0.5230301363771709955, 0.1775991818008312573, 0.9399606299212598381 ) ) ;
#21915=CARTESIAN_POINT ( 'NONE',  ( -0.5118110236220472231, 3.201384367575308305E-17, 1.766732283464566899 ) ) ;
#21917=CARTESIAN_POINT ( 'NONE',  ( 0.4300830224589536899, -0.3772436174784755680, 0.9399606299212598381 ) ) ;
#21933=VERTEX_POINT ( 'NONE', #13778 ) ;
#21938=B_SPLINE_CURVE_WITH_KNOTS ( 'NONE', 3,
 ( #22650, #11768, #20672, #12053, #13892, #1326, #5272, #20390, #24759, #16163, #11914, #763, #24613, #22228, #9495, #5562, #5422, #13609, #14041, #18091, #26456, #9354, #2991, #24472, #7119, #16016, #11624, #7247, #1192, #15866, #20247, #14187, #15742, #4987 ),
 .UNSPECIFIED., .F., .F.,
 ( 4, 2, 2, 2, 2, 2, 2, 2, 2, 2, 2, 2, 2, 2, 2, 2, 4 ),
 ( 0.5000000000000000000, 0.5312500000000000000, 0.5624999999999998890, 0.5937499999999998890, 0.6249999999999998890, 0.6562499999999998890, 0.6874999999999997780, 0.7187499999999997780, 0.7499999999999997780, 0.7812499999999997780, 0.8124999999999998890, 0.8437499999999998890, 0.8749999999999998890, 0.9062500000000000000, 0.9375000000000000000, 0.9687500000000000000, 1.000000000000000000 ),
 .UNSPECIFIED. ) ;
#21945=CARTESIAN_POINT ( 'NONE',  ( -0.4423390553432507977, -0.2180862235769348567, -1.569881889763779625 ) ) ;
#21947=CARTESIAN_POINT ( 'NONE',  ( 0.4351030398461604998, 0.1477428134820414352, -1.928289503579168951 ) ) ;
#21952=CARTESIAN_POINT ( 'NONE',  ( -0.03001016326913591784, 0.4585215200179055817, -1.928289503579156516 ) ) ;
#21962=CARTESIAN_POINT ( 'NONE',  ( 0.5511811023622047445, 3.414809992080329023E-17, 0.9202755905511811330 ) ) ;
#21965=CARTESIAN_POINT ( 'NONE',  ( -0.4303822302053990634, -0.1152775731717099322, -1.934055118110236338 ) ) ;
#21970=CARTESIAN_POINT ( 'NONE',  ( 0.2836590635674519634, 0.2488091035917033567, -3.100567304031761395 ) ) ;
#21975=CARTESIAN_POINT ( 'NONE',  ( -0.4417361510194065533, 0.05819755867303653962, -1.934055118110236338 ) ) ;
#21980=CARTESIAN_POINT ( 'NONE',  ( 0.4472135058506040983, 0.2577577458591219783, 1.766732283464566899 ) ) ;
#21982=CARTESIAN_POINT ( 'NONE',  ( -0.4856708409200499732, 0.1649135259616961724, 1.747047244094488194 ) ) ;
#21989=CARTESIAN_POINT ( 'NONE',  ( -0.3535721684717733071, -0.1200583359873110406, -3.115157480314960647 ) ) ;
#21993=CARTESIAN_POINT ( 'NONE',  ( 0.1482986320106562672, -0.3007905576423960392, 1.953740157480315043 ) ) ;
#22000=CARTESIAN_POINT ( 'NONE',  ( -0.1648275707511323573, -0.4857079805364574177, -1.550196850393701142 ) ) ;
#22001=ORIENTED_EDGE ( 'NONE', *, *, #15691, .F. ) ;
#22002=ORIENTED_EDGE ( 'NONE', *, *, #22244, .F. ) ;
#22003=CARTESIAN_POINT ( 'NONE',  ( 0.07874015748031480688, 0.1968503937007873850, -3.558522530913132531 ) ) ;
#22005=CARTESIAN_POINT ( 'NONE',  ( 0.01027864967365997931, 0.1968503937007874127, -3.193894829389441359 ) ) ;
#22007=CARTESIAN_POINT ( 'NONE',  ( 0.09842519685039355370, 0.2165354330708661457, -3.548228346456693050 ) ) ;
#22012=CARTESIAN_POINT ( 'NONE',  ( -0.3429980251342298336, -0.09187177619659059324, 1.953740157480315043 ) ) ;
#22019=CARTESIAN_POINT ( 'NONE',  ( 0.06699507805369657454, 0.5085118447801424413, 1.766732283464566899 ) ) ;
#22034=DIRECTION ( 'NONE',  ( 0.000000000000000000, 0.000000000000000000, 1.000000000000000000 ) ) ;
#22038=CARTESIAN_POINT ( 'NONE',  ( 0.3543307086614173596, 0.000000000000000000, 1.953740157480315043 ) ) ;
#22044=CARTESIAN_POINT ( 'NONE',  ( 0.5671862884094760471, 0.07472527936312113594, 0.9399606299212598381 ) ) ;
#22055=VERTEX_POINT ( 'NONE', #3885 ) ;
#22067=CARTESIAN_POINT ( 'NONE',  ( 0.006552947699234559081, 0.3149606299212598381, -3.646653543307086576 ) ) ;
#22069=CARTESIAN_POINT ( 'NONE',  ( -0.1585706980422225409, -0.4669911931914833558, -1.550196850393700920 ) ) ;
#22070=CARTESIAN_POINT ( 'NONE',  ( 0.4555658499975999698, -0.06001958459475366381, -1.928289503579165398 ) ) ;
#22071=ORIENTED_EDGE ( 'NONE', *, *, #12766, .F. ) ;
#22072=CARTESIAN_POINT ( 'NONE',  ( 0.2796934465393767222, -0.3645739570812915331, -1.928289503579138753 ) ) ;
#22076=CARTESIAN_POINT ( 'NONE',  ( 0.06001958459474798779, 0.4555658499976080189, -1.928289503579158515 ) ) ;
#22092=ADVANCED_FACE ( 'NONE', ( #17430, #9078 ), #21680, .T. ) ;
#22093=CARTESIAN_POINT ( 'NONE',  ( -0.4446020952038907681, 0.000000000000000000, -1.934055118110236338 ) ) ;
#22104=CARTESIAN_POINT ( 'NONE',  ( -0.2296683860596825943, 0.2993674444872254092, -3.100567304031761395 ) ) ;
#22110=FACE_OUTER_BOUND ( 'NONE', #6208, .T. ) ;
#22112=CARTESIAN_POINT ( 'NONE',  ( 0.4585215200179057482, 0.06002032661671145852, -1.928289503579156960 ) ) ;
#22116=CARTESIAN_POINT ( 'NONE',  ( -0.3121994997598253052, -0.4069448477556119048, 1.747047244094488194 ) ) ;
#22120=CARTESIAN_POINT ( 'NONE',  ( 0.3726024258163779246, 0.02438677169350801990, -3.115157480314960647 ) ) ;
#22125=CARTESIAN_POINT ( 'NONE',  ( -0.1677079028045287967, 0.2904160862623510475, 1.953740157480315043 ) ) ;
#22130=VERTEX_POINT ( 'NONE', #15343 ) ;
#22140=CARTESIAN_POINT ( 'NONE',  ( 0.07870736637777360489, 0.2165354330708661457, -3.212150913388296836 ) ) ;
#22142=CARTESIAN_POINT ( 'NONE',  ( -0.3429980251342297226, 0.09187177619658862260, 1.953740157480315043 ) ) ;
#22149=CARTESIAN_POINT ( 'NONE',  ( 0.3382184156732163660, 0.3855916753051394363, 1.766732283464566899 ) ) ;
#22154=EDGE_LOOP ( 'NONE', ( #21216, #23566, #6079, #8724 ) ) ;
#22155=CARTESIAN_POINT ( 'NONE',  ( -0.2313841235333771451, 0.3010840436257776198, -3.100567304031763172 ) ) ;
#22161=DIRECTION ( 'NONE',  ( 1.000000000000000000, 0.000000000000000000, 0.000000000000000000 ) ) ;
#22164=CARTESIAN_POINT ( 'NONE',  ( -0.5230301363771188150, -0.1775991818008711975, 0.9399606299212598381 ) ) ;
#22176=CARTESIAN_POINT ( 'NONE',  ( 0.3429980251342366060, 0.09187177619658697114, 1.953740157480315043 ) ) ;
#22196=VECTOR ( 'NONE', #7676, 39.37007874015748143 ) ;
#22204=CARTESIAN_POINT ( 'NONE',  ( -0.2660793235464258277, -0.2041304421298378857, 1.973425196850393970 ) ) ;
#22206=CARTESIAN_POINT ( 'NONE',  ( -0.3912931228432058872, -0.3001918266902326993, -1.550196850393700920 ) ) ;
#22208=CARTESIAN_POINT ( 'NONE',  ( 0.3454440660767458815, 0.3030032861725153737, -1.928289503579147635 ) ) ;
#22209=CARTESIAN_POINT ( 'NONE',  ( 0.06001958459476169905, -0.4555658499976140696, -1.928289503579150077 ) ) ;
#22219=CARTESIAN_POINT ( 'NONE',  ( -0.3346456692913385988, 0.000000000000000000, 2.426181102355854158 ) ) ;
#22225=B_SPLINE_CURVE_WITH_KNOTS ( 'NONE', 2,
 ( #24159, #9166, #22038 ),
 .UNSPECIFIED., .F., .F.,
 ( 3, 3 ),
 ( 0.000000000000000000, 1.000000000000000000 ),
 .UNSPECIFIED. ) ;
#22228=CARTESIAN_POINT ( 'NONE',  ( -0.1141156591735126569, 0.3362580771780235844, 1.953740157480314821 ) ) ;
#22230=CARTESIAN_POINT ( 'NONE',  ( 0.4527559054764770385, -0.02963280468032104126, -1.934055118110236338 ) ) ;
#22239=CARTESIAN_POINT ( 'NONE',  ( 0.02464264302293732445, -0.3765118517642105367, -3.100567304031763172 ) ) ;
#22243=CARTESIAN_POINT ( 'NONE',  ( -0.4303822302054170490, 0.1152775731717081975, -1.934055118110236338 ) ) ;
#22244=EDGE_CURVE ( 'NONE', #12810, #22996, #3020, .T. ) ;
#22251=CARTESIAN_POINT ( 'NONE',  ( -0.5118110236220472231, -0.03349795313264326835, 1.747047244094488194 ) ) ;
#22255=CARTESIAN_POINT ( 'NONE',  ( -0.1200583359873150374, -0.3535721684717939017, -3.115157480314960647 ) ) ;
#22264=CARTESIAN_POINT ( 'NONE',  ( 0.2938049579018460755, 0.3349573549949649842, -1.934055118110236338 ) ) ;
#22268=CARTESIAN_POINT ( 'NONE',  ( 0.01027864967283271050, 0.1968503937007874127, -3.626965695530909972 ) ) ;
#22271=CARTESIAN_POINT ( 'NONE',  ( -0.3381532161292066796, -0.3856588814717588076, -1.550196850393701142 ) ) ;
#22273=CARTESIAN_POINT ( 'NONE',  ( 0.09842519685039370636, 0.2165354330708661457, -3.364501312335958172 ) ) ;
#22275=CARTESIAN_POINT ( 'NONE',  ( 0.000000000000000000, 0.000000000000000000, -1.550196850393700920 ) ) ;
#22276=CARTESIAN_POINT ( 'NONE',  ( 0.08600259727896232553, 0.2165354330708660902, -3.223068997994990248 ) ) ;
#22277=CARTESIAN_POINT ( 'NONE',  ( -0.3346456692913385988, -0.04380501567505450111, 1.973425196850393526 ) ) ;
#22283=CARTESIAN_POINT ( 'NONE',  ( 0.2355331214654129424, 0.4777261797697872625, 1.747047244094488194 ) ) ;
#22289=EDGE_LOOP ( 'NONE', ( #157, #4921 ) ) ;
#22291=CARTESIAN_POINT ( 'NONE',  ( 0.02325127328526765264, -0.3543292900373042342, 1.953740157480315043 ) ) ;
#22294=VERTEX_POINT ( 'NONE', #22219 ) ;
#22295=CARTESIAN_POINT ( 'NONE',  ( -0.06441834428466709783, -0.4889536969035322977, -1.569881889763779625 ) ) ;
#22301=CARTESIAN_POINT ( 'NONE',  ( -0.5708661417322835607, 0.03736310157554031952, 0.9399606299212598381 ) ) ;
#22311=CONICAL_SURFACE ( 'NONE', #11479, 0.3135473077061334268, 0.2617993874999994808 ) ;
#22312=CYLINDRICAL_SURFACE ( 'NONE', #26704, 0.09842519685039378963 ) ;
#22314=CARTESIAN_POINT ( 'NONE',  ( -0.3324885138898231451, -0.04380447413659061678, 1.953740157480315043 ) ) ;
#22325=CARTESIAN_POINT ( 'NONE',  ( 0.3574975638436101444, 4.268512490100411279E-17, -3.115157480314960647 ) ) ;
#22326=ADVANCED_FACE ( 'NONE', ( #5553 ), #3125, .T. ) ;
#22332=CARTESIAN_POINT ( 'NONE',  ( -0.04838950581351151442, 0.1968503937007873850, -3.611194239255213656 ) ) ;
#22345=CARTESIAN_POINT ( 'NONE',  ( -0.1677079028045458664, 0.2904160862623615391, 1.973425196850393970 ) ) ;
#22346=CARTESIAN_POINT ( 'NONE',  ( -0.5085118447796660446, 0.06699507805605008082, -1.550196850393700920 ) ) ;
#22349=CARTESIAN_POINT ( 'NONE',  ( 0.2031943647053979507, -0.4121342552748326060, -1.928289503579156960 ) ) ;
#22351=CARTESIAN_POINT ( 'NONE',  ( -0.4382482975805212511, 0.3362148458989001609, 0.9399606299212598381 ) ) ;
#22355=CARTESIAN_POINT ( 'NONE',  ( -0.2031943647053863211, 0.4121342552748505916, -1.928289503579144748 ) ) ;
#22362=( NAMED_UNIT ( * ) SI_UNIT ( $, .STERADIAN. ) SOLID_ANGLE_UNIT ( ) ) ;
#22367=ORIENTED_EDGE ( 'NONE', *, *, #26753, .T. ) ;
#22372=CARTESIAN_POINT ( 'NONE',  ( -0.2268989272875881757, -0.3929158813954942153, -1.934055118110236338 ) ) ;
#22381=CARTESIAN_POINT ( 'NONE',  ( -0.09762295995069900090, 0.3644697409450268766, -3.100567304031763172 ) ) ;
#22394=CARTESIAN_POINT ( 'NONE',  ( 0.5118110236220472231, 0.000000000000000000, 1.766732283464566899 ) ) ;
#22399=CARTESIAN_POINT ( 'NONE',  ( -0.3384212623783161011, 0.1668516812751324463, -3.100567304031758287 ) ) ;
#22412=CARTESIAN_POINT ( 'NONE',  ( 0.4218945342797220666, 0.1432577568504696530, -1.934055118110236338 ) ) ;
#22414=CARTESIAN_POINT ( 'NONE',  ( -0.4921259842519685179, 6.026805113914139867E-17, -1.894685039405410665 ) ) ;
#22418=CARTESIAN_POINT ( 'NONE',  ( -0.03962771305321603071, 0.1968503937007874127, -3.203827438958285256 ) ) ;
#22421=B_SPLINE_CURVE_WITH_KNOTS ( 'NONE', 2,
 ( #21915, #10896, #17655 ),
 .UNSPECIFIED., .F., .F.,
 ( 3, 3 ),
 ( 0.000000000000000000, 1.000000000000000000 ),
 .UNSPECIFIED. ) ;
#22424=CARTESIAN_POINT ( 'NONE',  ( 0.2161381151963047975, 0.2817310484609297228, 1.953740157480315043 ) ) ;
#22430=CARTESIAN_POINT ( 'NONE',  ( 0.3855916753051596424, -0.3382184156732262470, 1.747047244094488194 ) ) ;
#22431=CARTESIAN_POINT ( 'NONE',  ( 0.03349795313264332386, 0.5118110236220472231, 1.766732283464566899 ) ) ;
#22437=FACE_OUTER_BOUND ( 'NONE', #4436, .T. ) ;
#22440=CARTESIAN_POINT ( 'NONE',  ( -0.4270824798167633385, 0.2466292688015202517, -1.569881889763779625 ) ) ;
#22442=CARTESIAN_POINT ( 'NONE',  ( 0.4382482975805214731, -0.3362148458988676314, 0.9399606299212598381 ) ) ;
#22444=FACE_OUTER_BOUND ( 'NONE', #10216, .T. ) ;
#22449=EDGE_CURVE ( 'NONE', #22055, #19192, #24141, .T. ) ;
#22457=CARTESIAN_POINT ( 'NONE',  ( -0.3324885138898230341, 0.04380447413659110945, 1.953740157480315043 ) ) ;
#22459=CARTESIAN_POINT ( 'NONE',  ( -0.4921259842519685179, 3.013402556957069934E-17, -1.569881889763779625 ) ) ;
#22460=CARTESIAN_POINT ( 'NONE',  ( -0.1188866373884864824, -0.4438564651657386229, -1.928289503579162067 ) ) ;
#22464=PRODUCT_DEFINITION_SHAPE ( 'NONE', 'NONE',  #18243 ) ;
#22470=CARTESIAN_POINT ( 'NONE',  ( -0.03349795313264251895, -0.5118110236220472231, 1.747047244094488194 ) ) ;
#22474=CARTESIAN_POINT ( 'NONE',  ( -0.02576258753917910760, 0.1968503937008544147, -3.644091798679130800 ) ) ;
#22486=B_SPLINE_CURVE_WITH_KNOTS ( 'NONE', 3,
 ( #3599, #18717, #27353, #8005, #1633, #12369, #16607, #25222, #14516, #9919, #3127, #13880, #14027, #26872, #9780, #1445, #18520, #20235 ),
 .UNSPECIFIED., .F., .F.,
 ( 4, 2, 2, 2, 2, 2, 2, 2, 4 ),
 ( 0.000000000000000000, 0.06250000000000004163, 0.1250000000000000555, 0.1875000000000000278, 0.2500000000000000555, 0.3125000000000000555, 0.3750000000000000000, 0.4375000000000000000, 0.5000000000000000000 ),
 .UNSPECIFIED. ) ;
#22487=DIRECTION ( 'NONE',  ( 0.000000000000000000, 0.000000000000000000, -1.000000000000000000 ) ) ;
#22490=CARTESIAN_POINT ( 'NONE',  ( 0.2041304421298337501, 0.2660793235464286033, 1.973425196850393970 ) ) ;
#22491=CARTESIAN_POINT ( 'NONE',  ( -0.1327036767636164405, 0.4954415918535620134, -1.550196850393700920 ) ) ;
#22493=CARTESIAN_POINT ( 'NONE',  ( 0.1775991818008606782, -0.5230301363771325818, 0.9202755905511811330 ) ) ;
#22508=DIRECTION ( 'NONE',  ( -0.000000000000000000, -0.000000000000000000, 1.000000000000000000 ) ) ;
#22514=CARTESIAN_POINT ( 'NONE',  ( -0.4069519308876702324, -0.2006393256663696334, -1.934055118110236338 ) ) ;
#22517=CARTESIAN_POINT ( 'NONE',  ( -0.006547182368340512953, 0.3149607547026831433, -3.174212199124641920 ) ) ;
#22527=CARTESIAN_POINT ( 'NONE',  ( -0.1668516812751398570, -0.3384212623783108276, -3.100567304031765392 ) ) ;
#22531=CARTESIAN_POINT ( 'NONE',  ( -0.3929158813954827245, 0.2268989272876178465, -1.934055118110236338 ) ) ;
#22533=EDGE_CURVE ( 'NONE', #19192, #24677, #20866, .T. ) ;
#22534=ORIENTED_EDGE ( 'NONE', *, *, #12766, .T. ) ;
#22537=CARTESIAN_POINT ( 'NONE',  ( 0.4856708409200598542, 0.1649135259617023896, 1.747047244094488194 ) ) ;
#22541=CARTESIAN_POINT ( 'NONE',  ( -0.3572819248074403653, -0.1213180142433946673, -3.100567304031765392 ) ) ;
#22545=LINE ( 'NONE', #12224, #18102 ) ;
#22550=CARTESIAN_POINT ( 'NONE',  ( -0.02909913904662089768, -0.4446020952038907681, -1.934055118110236338 ) ) ;
#22552=DIRECTION ( 'NONE',  ( -0.000000000000000000, -0.000000000000000000, -1.000000000000000000 ) ) ;
#22557=CARTESIAN_POINT ( 'NONE',  ( -0.3259357382551450466, 0.08759279594700321303, 1.973425196850394192 ) ) ;
#22560=AXIS2_PLACEMENT_3D ( 'NONE', #21736, #4498, #13379 ) ;
#22564=CARTESIAN_POINT ( 'NONE',  ( -0.04638120790932972332, -0.3520466617656973218, 1.953740157480315043 ) ) ;
#22570=CARTESIAN_POINT ( 'NONE',  ( 0.1712563538833041243, 0.5043504886477225835, 1.747047244094488194 ) ) ;
#22571=CARTESIAN_POINT ( 'NONE',  ( 0.3855916753051394363, 0.3382184156732163660, 1.766732283464566899 ) ) ;
#22579=CARTESIAN_POINT ( 'NONE',  ( -0.2938049579018706114, 0.3349573549949406148, -1.934055118110236338 ) ) ;
#22585=CARTESIAN_POINT ( 'NONE',  ( -0.1275996891957733581, -0.4763861460130334735, -1.569881889763779625 ) ) ;
#22614=DIRECTION ( 'NONE',  ( 1.000000000000000000, 0.000000000000000000, 0.000000000000000000 ) ) ;
#22617=CARTESIAN_POINT ( 'NONE',  ( 0.09842519684999338769, 0.1968503937007873850, -3.561114497143033297 ) ) ;
#22621=CARTESIAN_POINT ( 'NONE',  ( -0.3149606299212598381, 3.857155272905049219E-17, -3.115157480314960647 ) ) ;
#22625=CARTESIAN_POINT ( 'NONE',  ( 0.3667122560601320802, 0.09855118063547671503, -3.100567304031762728 ) ) ;
#22629=CARTESIAN_POINT ( 'NONE',  ( -0.08676778863011327947, 0.3239425792934402248, 1.973425196850393970 ) ) ;
#22630=CARTESIAN_POINT ( 'NONE',  ( -0.03349795313024159921, 0.5118110236220473341, -1.550196850393700920 ) ) ;
#22632=CARTESIAN_POINT ( 'NONE',  ( -0.2442565704126240245, -0.4954197419817664150, 0.9202755905511811330 ) ) ;
#22650=CARTESIAN_POINT ( 'NONE',  ( -0.3543307086614173596, 4.268512490100411279E-17, 1.953740157480315043 ) ) ;
#22652=CARTESIAN_POINT ( 'NONE',  ( 0.1173917140416396443, 0.4382752542996237732, -1.934055118110236338 ) ) ;
#22665=CARTESIAN_POINT ( 'NONE',  ( -0.3267488823401750730, -0.1886891683788910756, -3.100567304031762284 ) ) ;
#22668=CARTESIAN_POINT ( 'NONE',  ( -0.4303822302053990634, -0.1152775731717099322, -1.934055118110236338 ) ) ;
#22669=CARTESIAN_POINT ( 'NONE',  ( 0.4121342552748534227, 0.2031943647053804092, -1.928289503579144304 ) ) ;
#22672=B_SPLINE_CURVE_WITH_KNOTS ( 'NONE', 2,
 ( #12128, #18899, #27398 ),
 .UNSPECIFIED., .F., .F.,
 ( 3, 3 ),
 ( 0.000000000000000000, 1.000000000000000000 ),
 .UNSPECIFIED. ) ;
#22675=CARTESIAN_POINT ( 'NONE',  ( 0.1327036767659768302, -0.4954415918531079877, 1.747047244094488194 ) ) ;
#22679=CARTESIAN_POINT ( 'NONE',  ( 0.04928467685643989765, -0.3740848232703748444, -3.100567304031760507 ) ) ;
#22686=DIRECTION ( 'NONE',  ( -1.000000000000000000, 0.000000000000000000, 0.000000000000000000 ) ) ;
#22694=CARTESIAN_POINT ( 'NONE',  ( -0.1584254766472275311, 0.3213305936751604253, -3.115157480314960647 ) ) ;
#22708=CARTESIAN_POINT ( 'NONE',  ( 0.4724409448465559103, 6.026805113697782438E-17, 1.953740157480315043 ) ) ;
#22711=CARTESIAN_POINT ( 'NONE',  ( 0.4856708409200665155, -0.1649135259616916482, 1.747047244094488194 ) ) ;
#22713=CARTESIAN_POINT ( 'NONE',  ( 0.06699507805369034341, 0.5085118447801111330, 1.747047244094488194 ) ) ;
#22722=CARTESIAN_POINT ( 'NONE',  ( -0.2466292688015201129, 0.4270824798167635050, -1.569881889763779625 ) ) ;
#22734=CARTESIAN_POINT ( 'NONE',  ( 0.1482986320106562672, -0.3007905576423960392, 1.953740157480315043 ) ) ;
#22741=CARTESIAN_POINT ( 'NONE',  ( -0.3543307086614173596, 4.268512490100411279E-17, 1.953740157480315043 ) ) ;
#22742=CARTESIAN_POINT ( 'NONE',  ( -0.4300129863948118358, 0.2478439864030018147, -1.569881889763779625 ) ) ;
#22745=ORIENTED_EDGE ( 'NONE', *, *, #8273, .F. ) ;
#22757=EDGE_CURVE ( 'NONE', #18491, #26373, #13951, .T. ) ;
#22760=FACE_OUTER_BOUND ( 'NONE', #24755, .T. ) ;
#22762=CARTESIAN_POINT ( 'NONE',  ( 0.5118096047255313863, -0.03359157810808697381, -1.550196850393700920 ) ) ;
#22764=CARTESIAN_POINT ( 'NONE',  ( -0.3007905576423877680, -0.1482986320106428613, 1.973425196850393970 ) ) ;
#22766=CARTESIAN_POINT ( 'NONE',  ( 0.5118110236220473341, 0.03349795313024165472, -1.550196850393700920 ) ) ;
#22767=ADVANCED_FACE ( 'NONE', ( #19031, #1943 ), #25541, .T. ) ;
#22768=CARTESIAN_POINT ( 'NONE',  ( 0.07214943758244279914, 0.5511811023622046335, 0.9202755905511812440 ) ) ;
#22769=CARTESIAN_POINT ( 'NONE',  ( -0.2762247810519161129, -0.4783323773986413729, 0.9202755905511811330 ) ) ;
#22792=CARTESIAN_POINT ( 'NONE',  ( 0.1458850421962665789, 0.4296318976990154970, -1.934055118110236338 ) ) ;
#22795=CARTESIAN_POINT ( 'NONE',  ( 0.04992990154984337792, 0.3112132001918756496, -3.186824010432603327 ) ) ;
#22812=CARTESIAN_POINT ( 'NONE',  ( 0.1970259548082060608, 0.3996230174612934172, -1.934055118110236338 ) ) ;
#22814=CARTESIAN_POINT ( 'NONE',  ( 0.3645739570812633890, 0.2796934465393874358, -1.928289503579156072 ) ) ;
#22822=CARTESIAN_POINT ( 'NONE',  ( 0.4600326175560532915, -0.2268096725222599475, 1.747047244094488194 ) ) ;
#22828=CARTESIAN_POINT ( 'NONE',  ( 0.1213180142433833847, 0.3572819248074460829, -3.100567304031761395 ) ) ;
#22834=CARTESIAN_POINT ( 'NONE',  ( -0.4225434286521154159, 0.3242892624566993121, 1.747047244094488194 ) ) ;
#22835=CARTESIAN_POINT ( 'NONE',  ( 0.3858397471888846408, -0.2228126397719881469, -1.934055118110236338 ) ) ;
#22842=CARTESIAN_POINT ( 'NONE',  ( -0.02339816079119156136, -0.3574975638436101444, -3.115157480314960647 ) ) ;
#22845=DIRECTION ( 'NONE',  ( -1.000000000000000000, 0.000000000000000000, 0.000000000000000000 ) ) ;
#22848=CARTESIAN_POINT ( 'NONE',  ( 0.1685339107540412551, -0.2924088307484720706, 1.973425196850393970 ) ) ;
#22849=CARTESIAN_POINT ( 'NONE',  ( 0.3543307086614173596, -0.02319089060379044345, 1.953740157480315043 ) ) ;
#22852=CARTESIAN_POINT ( 'NONE',  ( 0.03746919241557470498, 0.5708647227724243933, 0.9399606299212600602 ) ) ;
#22861=CARTESIAN_POINT ( 'NONE',  ( -0.4777261797697566759, 0.2355331214654138305, 1.747047244094488194 ) ) ;
#22862=CARTESIAN_POINT ( 'NONE',  ( 0.03349795313264332386, 0.5118110236220472231, 1.747047244094488194 ) ) ;
#22866=CARTESIAN_POINT ( 'NONE',  ( -0.3213305936751693626, 0.1584254766472210918, -3.115157480314960647 ) ) ;
#22871=CARTESIAN_POINT ( 'NONE',  ( -0.5511811023622047445, 3.375010863791918375E-17, 0.9202755905511811330 ) ) ;
#22875=CARTESIAN_POINT ( 'NONE',  ( 0.3912931228432222075, -0.3001918266902142696, -1.569881889763779625 ) ) ;
#22903=CARTESIAN_POINT ( 'NONE',  ( -0.2268096725200377806, -0.4600326175569655618, -1.550196850393700920 ) ) ;
#22904=CARTESIAN_POINT ( 'NONE',  ( 0.000000000000000000, 0.000000000000000000, 0.9399606299212598381 ) ) ;
#22905=DIRECTION ( 'NONE',  ( 0.2588190448135617161, 0.000000000000000000, 0.9659258263664945998 ) ) ;
#22906=CARTESIAN_POINT ( 'NONE',  ( 0.06296589279854435117, 0.1968503937007873850, -3.596617852270155513 ) ) ;
#22915=CARTESIAN_POINT ( 'NONE',  ( 0.3856588814717663571, -0.3381532161291455618, -1.550196850393700476 ) ) ;
#22919=CARTESIAN_POINT ( 'NONE',  ( 0.4954415918535723939, -0.1327036767636087800, -1.550196850393700920 ) ) ;
#22921=CARTESIAN_POINT ( 'NONE',  ( 0.4954197419817656933, 0.2442565704126251624, 0.9202755905511811330 ) ) ;
#22955=ORIENTED_EDGE ( 'NONE', *, *, #5693, .F. ) ;
#22956=CARTESIAN_POINT ( 'NONE',  ( 0.4446020952038907681, -0.02909913904662010317, -1.934055118110236338 ) ) ;
#22963=CARTESIAN_POINT ( 'NONE',  ( 0.07874015748031495954, 0.1968503937007873850, -3.456364829396327387 ) ) ;
#22965=CARTESIAN_POINT ( 'NONE',  ( 0.03478633594543729946, 0.5314960629921260393, 1.747047244094488194 ) ) ;
#22969=CARTESIAN_POINT ( 'NONE',  ( 0.2993674444872233553, -0.2296683860596848981, -3.100567304031763172 ) ) ;
#22974=CARTESIAN_POINT ( 'NONE',  ( -0.3543307086614173596, 0.02319089060378165187, 1.953740157480315043 ) ) ;
#22980=CARTESIAN_POINT ( 'NONE',  ( 0.03736310157557554135, 0.5708661417322835607, 0.9399606299212598381 ) ) ;
#22982=EDGE_CURVE ( 'NONE', #13505, #18491, #20340, .T. ) ;
#22988=CARTESIAN_POINT ( 'NONE',  ( -0.3392387706403586223, -0.1151913129404420061, -3.115157480314960647 ) ) ;
#22990=CIRCLE ( 'NONE', #5374, 0.3149606299212598381 ) ;
#22992=DIRECTION ( 'NONE',  ( 1.000000000000000000, 0.000000000000000000, 0.000000000000000000 ) ) ;
#22996=VERTEX_POINT ( 'NONE', #22414 ) ;
#22997=CARTESIAN_POINT ( 'NONE',  ( -0.5525844203311578440, 0.1481265526513353969, 0.9399606299212601712 ) ) ;
#23002=CARTESIAN_POINT ( 'NONE',  ( 0.5314960629921260393, 0.000000000000000000, 1.747047244094488194 ) ) ;
#23006=CARTESIAN_POINT ( 'NONE',  ( -0.4441657790107744752, -0.2564944395515745823, 1.766732283464566899 ) ) ;
#23017=CARTESIAN_POINT ( 'NONE',  ( -0.3912931228432124930, 0.3001918266902225407, -1.550196850393700920 ) ) ;
#23035=CARTESIAN_POINT ( 'NONE',  ( -0.5905511811023621549, 7.232166136696967594E-17, 1.707677165389662743 ) ) ;
#23045=CARTESIAN_POINT ( 'NONE',  ( -0.4069448477569433953, -0.3121994997578269593, -1.550196850393700920 ) ) ;
#23056=CARTESIAN_POINT ( 'NONE',  ( -0.4442166144910411063, -0.2564158049327064925, -1.550196850393700920 ) ) ;
#23063=CARTESIAN_POINT ( 'NONE',  ( 0.4068916527365293856, -0.3122765577857888331, -1.550196850393700920 ) ) ;
#23065=CARTESIAN_POINT ( 'NONE',  ( 0.3007905576423883232, 0.1482986320106616795, 1.953740157480315043 ) ) ;
#23066=CARTESIAN_POINT ( 'NONE',  ( 0.5085118447796559416, -0.06699507805604926203, -1.550196850393700920 ) ) ;
#23067=CARTESIAN_POINT ( 'NONE',  ( -0.4446020952038907681, 0.000000000000000000, -1.934055118110236338 ) ) ;
#23068=CARTESIAN_POINT ( 'NONE',  ( -0.5708661417322835607, 0.000000000000000000, 0.9399606299212598381 ) ) ;
#23073=EDGE_CURVE ( 'NONE', #20420, #20990, #13938, .T. ) ;
#23079=CARTESIAN_POINT ( 'NONE',  ( 0.3242876858384301508, -0.4225410690758546473, 1.747047244094488194 ) ) ;
#23095=CARTESIAN_POINT ( 'NONE',  ( 0.1585706980422492418, -0.4669911931914798586, -1.569881889763779625 ) ) ;
#23098=CARTESIAN_POINT ( 'NONE',  ( 0.4303822302054278182, -0.1152775731717046309, -1.934055118110236338 ) ) ;
#23106=CARTESIAN_POINT ( 'NONE',  ( -0.06957181182498481387, 0.5280699926563169333, 1.747047244094488194 ) ) ;
#23110=CARTESIAN_POINT ( 'NONE',  ( 0.1886891683788910479, -0.3267488823401750730, -3.100567304031762284 ) ) ;
#23111=CARTESIAN_POINT ( 'NONE',  ( -0.09193127540133588793, -0.3429876364231727037, 1.953740157480314821 ) ) ;
#23115=CARTESIAN_POINT ( 'NONE',  ( -0.3074993854542729665, -0.1775730735577446262, 1.953740157480315043 ) ) ;
#23120=CARTESIAN_POINT ( 'NONE',  ( 0.4954197419818043846, -0.2442565704126259674, 0.9399606299212598381 ) ) ;
#23128=CARTESIAN_POINT ( 'NONE',  ( 0.2693339498142252042, 0.2362439534887496861, -3.115157480314960647 ) ) ;
#23129=CARTESIAN_POINT ( 'NONE',  ( -0.1442704874421230077, -0.5368353335967094297, 0.9202755905511812440 ) ) ;
#23136=CARTESIAN_POINT ( 'NONE',  ( -0.5130713940405708939, 0.2530774914993670910, 0.9399606299212600602 ) ) ;
#23142=CARTESIAN_POINT ( 'NONE',  ( 0.07870736637777375755, 0.2165354330708660624, -3.608715228343986503 ) ) ;
#23145=CARTESIAN_POINT ( 'NONE',  ( -0.1649135259617057203, -0.4856708409200641841, 1.766732283464566899 ) ) ;
#23150=CARTESIAN_POINT ( 'NONE',  ( 0.2309201403895322358, -0.4006498629591506155, -1.928289503579156960 ) ) ;
#23153=B_SPLINE_CURVE_WITH_KNOTS ( 'NONE', 2,
 ( #6011, #10506, #8126 ),
 .UNSPECIFIED., .F., .F.,
 ( 3, 3 ),
 ( 0.000000000000000000, 1.000000000000000000 ),
 .UNSPECIFIED. ) ;
#23154=CARTESIAN_POINT ( 'NONE',  ( -0.3324885138898239778, 0.04380447413658877104, 1.973425196850393970 ) ) ;
#23157=CARTESIAN_POINT ( 'NONE',  ( -0.3001918266902322552, -0.3912931228432061648, -1.550196850393700920 ) ) ;
#23189=CARTESIAN_POINT ( 'NONE',  ( -0.3855916753034467903, -0.3382184156749090675, -1.550196850393700920 ) ) ;
#23193=CARTESIAN_POINT ( 'NONE',  ( -0.1775991818008739453, 0.5230301363771271417, 0.9202755905511811330 ) ) ;
#23204=CARTESIAN_POINT ( 'NONE',  ( 0.08676778863010879694, -0.3239425792934411685, 1.973425196850393970 ) ) ;
#23205=CARTESIAN_POINT ( 'NONE',  ( -0.1649135259639108730, -0.4856708409191554665, -1.550196850393700920 ) ) ;
#23209=CARTESIAN_POINT ( 'NONE',  ( 0.3362148458988353239, 0.4382482975805538361, 0.9399606299212598381 ) ) ;
#23213=ORIENTED_EDGE ( 'NONE', *, *, #14207, .T. ) ;
#23214=CARTESIAN_POINT ( 'NONE',  ( 0.09275304139143687732, 0.3460530745557324206, -3.115157480314960647 ) ) ;
#23217=CARTESIAN_POINT ( 'NONE',  ( 0.4776874499715109135, 0.2356229156554291715, 1.747047244094487528 ) ) ;
#23220=CARTESIAN_POINT ( 'NONE',  ( -0.4600326175569863785, 0.2268096725200117181, -1.550196850393700920 ) ) ;
#23224=CARTESIAN_POINT ( 'NONE',  ( -0.1711654736996711390, -0.5043865966254131861, 1.747047244094488194 ) ) ;
#23239=CARTESIAN_POINT ( 'NONE',  ( -0.3102827802123664935, -0.1791101711252766349, -3.115157480314960647 ) ) ;
#23244=CARTESIAN_POINT ( 'NONE',  ( 0.2761764805255846333, -0.3599896729929844552, -1.934055118110236338 ) ) ;
#23245=CARTESIAN_POINT ( 'NONE',  ( 0.4121342552748372690, -0.2031943647053953139, -1.928289503579153630 ) ) ;
#23251=CARTESIAN_POINT ( 'NONE',  ( -0.4004221243553304777, 0.3512268162760389667, 1.747047244094488194 ) ) ;
#23257=CARTESIAN_POINT ( 'NONE',  ( -0.2161891097064467526, -0.2816986811833155913, 1.953740157480314821 ) ) ;
#23259=CARTESIAN_POINT ( 'NONE',  ( 0.4417530401346461688, 0.05811992390560041799, -1.934055118110236116 ) ) ;
#23261=CARTESIAN_POINT ( 'NONE',  ( -0.3362336590883616139, -0.1141709026133614219, 1.953740157480315043 ) ) ;
#23265=VERTEX_POINT ( 'NONE', #4122 ) ;
#23267=CARTESIAN_POINT ( 'NONE',  ( -0.5671862884095228985, -0.07472527936312044206, 0.9399606299212598381 ) ) ;
#23273=CARTESIAN_POINT ( 'NONE',  ( -0.1584254766472190379, -0.3213305936751582048, -3.115157480314960647 ) ) ;
#23275=CARTESIAN_POINT ( 'NONE',  ( -0.3387265385688505437, -0.4407612517155324316, 0.9202755905511810219 ) ) ;
#23294=CARTESIAN_POINT ( 'NONE',  ( -0.4954415918530867824, -0.1327036767659759697, 1.747047244094488194 ) ) ;
#23297=CARTESIAN_POINT ( 'NONE',  ( -0.3702005978258633423, 0.04877294052296513721, -3.115157480314960647 ) ) ;
#23300=CARTESIAN_POINT ( 'NONE',  ( 0.1200170377978877767, -0.4465874321618642506, -1.928289503579156294 ) ) ;
#23304=CARTESIAN_POINT ( 'NONE',  ( -0.2041304421298429650, -0.2660793235464223860, 1.973425196850393970 ) ) ;
#23308=CARTESIAN_POINT ( 'NONE',  ( 0.4763861460130703329, 0.1275996891957705826, -1.550196850393700920 ) ) ;
#23319=CARTESIAN_POINT ( 'NONE',  ( 0.3995939286813819935, -0.1970998888482827227, -1.934055118110237004 ) ) ;
#23329=CARTESIAN_POINT ( 'NONE',  ( 0.2817828961649165298, 0.3666644560843322909, -1.928289503579156294 ) ) ;
#23344=CARTESIAN_POINT ( 'NONE',  ( -0.4382482975805018222, 0.3362148458988871713, 0.9202755905511811330 ) ) ;
#23358=CARTESIAN_POINT ( 'NONE',  ( 0.3007905576423843819, -0.1482986320106508549, 1.973425196850393970 ) ) ;
#23359=CARTESIAN_POINT ( 'NONE',  ( 0.06699507805604380806, -0.5085118447796470598, -1.550196850393700920 ) ) ;
#23363=CARTESIAN_POINT ( 'NONE',  ( -0.4954197419817796266, -0.2442565704126152260, 0.9399606299212598381 ) ) ;
#23367=B_SPLINE_SURFACE_WITH_KNOTS ( 'NONE', 2, 3, ( 
 ( #5036, #9259, #17875, #20292, #952, #3183, #11816, #27507, #16616, #6182, #27647, #18725, #22694, #10115, #5897, #1642, #8011, #12520, #11961, #10393, #20581, #3320, #18432, #1235, #27082, #23128, #3607, #16760, #3465, #16345, #8290, #9974, #1362, #14525, #20996, #10244, #14670, #24943, #25372, #19011, #12237, #5607, #6034, #18574, #20716, #3756, #14235, #18863, #27218, #22842, #12096, #7867, #16476, #23273, #25089, #3903, #21137, #1779, #16906, #5755, #14376, #22988, #20854, #1503, #27361, #12378 ),
 ( #10956, #2995, #2468, #6725, #13206, #382, #8829, #17453, #11093, #21834, #8561, #14942, #19715, #8964, #26068, #23554, #12927, #17587, #23419, #10533, #6311, #26200, #4187, #21551, #4461, #8423, #10817, #13075, #14810, #17178, #2197, #15361, #15076, #23689, #12796, #2059, #4050, #19433, #124, #4322, #6585, #25657, #12655, #21284, #21422, #15211, #27782, #23820, #21699, #1921, #23954, #17043, #19149, #10672, #19291, #25793, #6441, #2327, #19580, #259, #7129, #17971, #24086, #1065, #26336, #26608 ),
 ( #7405, #11639, #2866, #17714, #6860, #637, #7261, #17846, #13345, #9659, #22104, #13474, #779, #5135, #22381, #26751, #18260, #20261, #3154, #24356, #15487, #18106, #2733, #4859, #9367, #21970, #3003, #11365, #9095, #4722, #6999, #15622, #13762, #19981, #9506, #24625, #920, #16027, #24221, #2599, #9225, #26467, #15753, #5284, #15883, #4998, #11223, #13620, #22239, #11505, #20118, #24487, #13908, #22527, #14052, #5439, #16176, #20547, #24773, #22665, #1204, #26896, #3290, #11929, #9804, #7547 ) ),
 .UNSPECIFIED., .F., .T., .F.,
 ( 3, 3 ),
 ( 4, 2, 2, 2, 2, 2, 2, 2, 2, 2, 2, 2, 2, 2, 2, 2, 2, 2, 2, 2, 2, 2, 2, 2, 2, 2, 2, 2, 2, 2, 2, 2, 4 ),
 ( 0.000000000000000000, 1.000000000000000000 ),
 ( 0.000000000000000000, 0.1963495408493620697, 0.3926990816987241395, 0.5890486225480862092, 0.7853981633974482790, 0.9817477042468103487, 1.178097245096172418, 1.374446785945534488, 1.570796326794896558, 1.767145867644258628, 1.963495408493620697, 2.159844949342982545, 2.356194490192344837, 2.552544031041707129, 2.748893571891068976, 2.945243112740430824, 3.141592653589793116, 3.337942194439155408, 3.534291735288517255, 3.730641276137879103, 3.926990816987241395, 4.123340357836603687, 4.319689898685965090, 4.516039439535327382, 4.712388980384689674, 4.908738521234051966, 5.105088062083414258, 5.301437602932775661, 5.497787143782137953, 5.694136684631500245, 5.890486225480861648, 6.086835766330223940, 6.283185307179586232 ),
 .UNSPECIFIED. ) ;
#23368=CARTESIAN_POINT ( 'NONE',  ( -0.2842163005027485978, 0.2181214148711163314, -3.115157480314960203 ) ) ;
#23371=CARTESIAN_POINT ( 'NONE',  ( -0.4301570366550043767, -0.3771675965699594624, 0.9399606299212597271 ) ) ;
#23389=CARTESIAN_POINT ( 'NONE',  ( 0.1173917140416396443, 0.4382752542996237732, -1.934055118110236338 ) ) ;
#23406=CARTESIAN_POINT ( 'NONE',  ( 0.3543307086614173596, 0.000000000000000000, 1.953740157480315043 ) ) ;
#23419=CARTESIAN_POINT ( 'NONE',  ( 0.04877294052295595012, 0.3702005978258479102, -3.115157480314960647 ) ) ;
#23422=DIRECTION ( 'NONE',  ( 0.000000000000000000, 0.000000000000000000, -1.000000000000000000 ) ) ;
#23426=CARTESIAN_POINT ( 'NONE',  ( -0.5511811023622047445, 0.03607471876259063515, 0.9202755905511811330 ) ) ;
#23427=ORIENTED_EDGE ( 'NONE', *, *, #18095, .F. ) ;
#23432=CARTESIAN_POINT ( 'NONE',  ( -0.5085118447801421082, 0.06699507805369804558, 1.766732283464566899 ) ) ;
#23436=CIRCLE ( 'NONE', #23871, 0.3937007874015748254 ) ;
#23437=CARTESIAN_POINT ( 'NONE',  ( -0.09269288654273742656, -0.3460635936745020680, -3.115157480314960647 ) ) ;
#23445=CARTESIAN_POINT ( 'NONE',  ( -0.3346456692913385988, -0.02190250779246036283, 1.973425196850393970 ) ) ;
#23448=CARTESIAN_POINT ( 'NONE',  ( 0.3912931228432187658, 0.3001918266902420251, -1.550196850393700920 ) ) ;
#23458=CARTESIAN_POINT ( 'NONE',  ( -0.09842519685039387289, 0.2991866959364304357, -3.554781501636282037 ) ) ;
#23471=CARTESIAN_POINT ( 'NONE',  ( 0.07874015747999522918, 0.1968503937007873850, -3.262328874726532213 ) ) ;
#23476=DIRECTION ( 'NONE',  ( 1.000000000000000000, 0.000000000000000000, 0.000000000000000000 ) ) ;
#23482=CARTESIAN_POINT ( 'NONE',  ( 0.5476281405333177643, 0.07214854559198216610, 0.9202755905511811330 ) ) ;
#23491=CARTESIAN_POINT ( 'NONE',  ( 0.000000000000000000, 0.000000000000000000, 1.707677165389662743 ) ) ;
#23497=AXIS2_PLACEMENT_3D ( 'NONE', #3798, #1677, #16944 ) ;
#23498=CARTESIAN_POINT ( 'NONE',  ( 0.5335524835332415838, 0.1429116519061139345, 0.9399606299212598381 ) ) ;
#23501=CARTESIAN_POINT ( 'NONE',  ( 0.3460502918090235247, 0.09275248786873148410, -3.115157480314960203 ) ) ;
#23507=CARTESIAN_POINT ( 'NONE',  ( 0.2268096725200263730, 0.4600326175569572351, -1.550196850393700920 ) ) ;
#23509=CARTESIAN_POINT ( 'NONE',  ( 0.5417516942598733509, -0.1838445375782305768, 0.9399606299212601712 ) ) ;
#23524=PRODUCT_DEFINITION_CONTEXT ( 'detailed design', #21371, 'design' ) ;
#23525=CARTESIAN_POINT ( 'NONE',  ( 0.2006393256663384084, 0.4069519308876483610, -1.934055118110236338 ) ) ;
#23529=AXIS2_PLACEMENT_3D ( 'NONE', #8558, #17177, #25791 ) ;
#23543=CARTESIAN_POINT ( 'NONE',  ( -0.1570220809524473238, 0.3184841198566425446, 1.953740157480315043 ) ) ;
#23548=CARTESIAN_POINT ( 'NONE',  ( -0.2860899518037610667, -0.4954156765914530247, 0.9399606299212598381 ) ) ;
#23550=CARTESIAN_POINT ( 'NONE',  ( 0.000000000000000000, 0.000000000000000000, -1.550196850393700920 ) ) ;
#23554=CARTESIAN_POINT ( 'NONE',  ( -0.04877294052296160531, 0.3702005978258477437, -3.115157480314960647 ) ) ;
#23566=ORIENTED_EDGE ( 'NONE', *, *, #11576, .T. ) ;
#23569=CARTESIAN_POINT ( 'NONE',  ( -0.1327036767659680594, 0.4954415918530845619, 1.766732283464566899 ) ) ;
#23571=CARTESIAN_POINT ( 'NONE',  ( -0.3855916753051397139, 0.3382184156732160329, 1.747047244094488194 ) ) ;
#23575=CARTESIAN_POINT ( 'NONE',  ( 0.09269288654274054906, 0.3460635936744927976, -3.115157480314960647 ) ) ;
#23580=CARTESIAN_POINT ( 'NONE',  ( 0.2660793235464301021, -0.2041304421298313909, 1.973425196850393970 ) ) ;
#23582=ORIENTED_EDGE ( 'NONE', *, *, #6894, .T. ) ;
#23585=CARTESIAN_POINT ( 'NONE',  ( 0.4270824798167666692, -0.2466292688015215839, -1.550196850393700920 ) ) ;
#23591=CYLINDRICAL_SURFACE ( 'NONE', #22560, 0.3937007874015748254 ) ;
#23605=CARTESIAN_POINT ( 'NONE',  ( 0.4921259842519686289, 0.06441914069860960046, -1.569881889763779625 ) ) ;
#23607=CARTESIAN_POINT ( 'NONE',  ( 0.04956879678463937261, 0.1968503937007873850, -3.186635197791150453 ) ) ;
#23625=ORIENTED_EDGE ( 'NONE', *, *, #12749, .T. ) ;
#23631=DIRECTION ( 'NONE',  ( 1.000000000000000000, 0.000000000000000000, 0.000000000000000000 ) ) ;
#23632=CIRCLE ( 'NONE', #10068, 0.3149606299212598381 ) ;
#23633=CARTESIAN_POINT ( 'NONE',  ( 0.4954197419818043846, -0.2442565704126259674, 0.9399606299212598381 ) ) ;
#23634=LINE ( 'NONE', #334, #10113 ) ;
#23643=CARTESIAN_POINT ( 'NONE',  ( 0.3483115186085852799, -0.4538422614029385405, 0.9399606299212601712 ) ) ;
#23646=CARTESIAN_POINT ( 'NONE',  ( -0.5314946440730490274, -0.03488411621207028468, 1.747047244094488416 ) ) ;
#23664=CARTESIAN_POINT ( 'NONE',  ( 0.2466292688015071233, 0.4270824798167958125, -1.550196850393700920 ) ) ;
#23666=CARTESIAN_POINT ( 'NONE',  ( 0.3929158813954875540, -0.2268989272875726881, -1.934055118110236338 ) ) ;
#23683=CARTESIAN_POINT ( 'NONE',  ( 0.1839420097223035677, -0.5417097841048799101, 0.9399606299212598381 ) ) ;
#23689=CARTESIAN_POINT ( 'NONE',  ( 0.3726024258163779246, -0.02438677169350792623, -3.115157480314960647 ) ) ;
#23691=CARTESIAN_POINT ( 'NONE',  ( -0.02576258704323625137, 0.2165354330708661734, -3.644091798884676159 ) ) ;
#23703=CARTESIAN_POINT ( 'NONE',  ( -0.06699507805369578350, -0.5085118447801426633, 1.766732283464566899 ) ) ;
#23709=CARTESIAN_POINT ( 'NONE',  ( -0.3392387706403586223, -0.1151913129404420061, -3.115157480314960647 ) ) ;
#23714=CARTESIAN_POINT ( 'NONE',  ( -0.3007905576423873240, 0.1482986320106437494, 1.973425196850393970 ) ) ;
#23715=CARTESIAN_POINT ( 'NONE',  ( -0.02576258753924276154, 0.2165354330708661457, -3.644091798679223615 ) ) ;
#23728=CYLINDRICAL_SURFACE ( 'NONE', #6528, 0.3149606299212598381 ) ;
#23738=CARTESIAN_POINT ( 'NONE',  ( -0.09842519685039377575, 0.2165354330708661457, -3.259751644589249597 ) ) ;
#23742=SHAPE_REPRESENTATION_RELATIONSHIP ( 'NONE' , 'NONE' ,  #713, #15726 ) ;
#23744=EDGE_CURVE ( 'NONE', #1806, #24677, #21875, .T. ) ;
#23750=CARTESIAN_POINT ( 'NONE',  ( 0.3642352168757554964, -0.4152525734086275899, 0.9202755905511811330 ) ) ;
#23758=VECTOR ( 'NONE', #17272, 39.37007874015748854 ) ;
#23763=CARTESIAN_POINT ( 'NONE',  ( -2.685748425196850164E-17, 0.000000000000000000, -3.115157480314960647 ) ) ;
#23767=CARTESIAN_POINT ( 'NONE',  ( -0.03736310157557653361, -0.5708661417322835607, 0.9399606299212598381 ) ) ;
#23769=CARTESIAN_POINT ( 'NONE',  ( -2.685748425196850164E-17, 0.000000000000000000, -3.115157480314960647 ) ) ;
#23778=CARTESIAN_POINT ( 'NONE',  ( -0.4921259842519685179, 0.000000000000000000, -1.550196850393700920 ) ) ;
#23795=CARTESIAN_POINT ( 'NONE',  ( -0.4669911931914605407, 0.1585706980422390278, -1.550196850393700920 ) ) ;
#23797=CARTESIAN_POINT ( 'NONE',  ( 0.4382752542996382616, -0.1173917140416361471, -1.934055118110236338 ) ) ;
#23798=EDGE_CURVE ( 'NONE', #7673, #5072, #4505, .T. ) ;
#23806=CARTESIAN_POINT ( 'NONE',  ( -0.3543292900373042897, -0.02325127328527671483, 1.953740157480314599 ) ) ;
#23812=CARTESIAN_POINT ( 'NONE',  ( -0.2268989272875546748, 0.3929158813954828355, -1.934055118110236338 ) ) ;
#23820=CARTESIAN_POINT ( 'NONE',  ( 0.04877294052296175797, -0.3702005978258584573, -3.115157480314960647 ) ) ;
#23838=CARTESIAN_POINT ( 'NONE',  ( -0.4441657790107740866, 0.2564944395515753039, 1.766732283464566899 ) ) ;
#23844=CARTESIAN_POINT ( 'NONE',  ( -0.2807137536170428715, 0.2462256503456040635, -3.115157480314960647 ) ) ;
#23852=CARTESIAN_POINT ( 'NONE',  ( -0.2521176338356424518, 0.2211428102655600414, 1.953740157480315043 ) ) ;
#23855=ORIENTED_EDGE ( 'NONE', *, *, #11576, .F. ) ;
#23863=B_SPLINE_CURVE_WITH_KNOTS ( 'NONE', 3,
 ( #13356, #21571, #6738, #21980, #2207, #8708, #6870, #8972, #13087, #15500, #21711, #15632, #11235, #26348, #4874, #2614, #19860, #24235 ),
 .UNSPECIFIED., .F., .F.,
 ( 4, 2, 2, 2, 2, 2, 2, 2, 4 ),
 ( 0.000000000000000000, 0.06250000000000000000, 0.1250000000000000000, 0.1875000000000000000, 0.2500000000000000000, 0.3125000000000000000, 0.3750000000000000000, 0.4375000000000000000, 0.5000000000000000000 ),
 .UNSPECIFIED. ) ;
#23865=CARTESIAN_POINT ( 'NONE',  ( -1.452994488188976472E-16, 0.3149606299212598381, -3.646653543307086576 ) ) ;
#23871=AXIS2_PLACEMENT_3D ( 'NONE', #26543, #20484, #20347 ) ;
#23877=CARTESIAN_POINT ( 'NONE',  ( 0.04956879678462317029, 0.2165354330708661457, -3.186635197791187757 ) ) ;
#23887=ORIENTED_EDGE ( 'NONE', *, *, #23744, .T. ) ;
#23888=CARTESIAN_POINT ( 'NONE',  ( -0.03607471876262473287, 0.5511811023622048555, 0.9399606299212598381 ) ) ;
#23907=CARTESIAN_POINT ( 'NONE',  ( -0.3482225189666507403, -0.4539000224941303063, 0.9399606299212598381 ) ) ;
#23916=ADVANCED_FACE ( 'NONE', ( #9135 ), #17754, .T. ) ;
#23921=EDGE_CURVE ( 'NONE', #10030, #19599, #14617, .T. ) ;
#23929=CARTESIAN_POINT ( 'NONE',  ( 0.04991721480923575621, 0.3112151455537437439, -3.634049048173129126 ) ) ;
#23930=CARTESIAN_POINT ( 'NONE',  ( 0.3912931228432187658, 0.3001918266902420251, -1.550196850393700920 ) ) ;
#23931=CARTESIAN_POINT ( 'NONE',  ( 0.2297883689023240139, -0.3979194638820313656, -1.928289503579174280 ) ) ;
#23932=AXIS2_PLACEMENT_3D ( 'NONE', #10456, #7790, #16401 ) ;
#23934=ADVANCED_FACE ( 'NONE', ( #25095 ), #14241, .T. ) ;
#23946=CARTESIAN_POINT ( 'NONE',  ( -0.1173917140416340377, 0.4382752542996236622, -1.934055118110236338 ) ) ;
#23953=CARTESIAN_POINT ( 'NONE',  ( -0.2937477835495413414, -0.3350125228557411239, -1.934055118110236560 ) ) ;
#23954=CARTESIAN_POINT ( 'NONE',  ( -0.04877294052295848975, -0.3702005978258383068, -3.115157480314960647 ) ) ;
#23959=CARTESIAN_POINT ( 'NONE',  ( -0.1152775731717075036, 0.4303822302054133853, -1.934055118110236338 ) ) ;
#23962=ORIENTED_EDGE ( 'NONE', *, *, #14363, .T. ) ;
#23964=CARTESIAN_POINT ( 'NONE',  ( 0.4856708409200646281, 0.1649135259617043880, 1.766732283464566899 ) ) ;
#23969=CARTESIAN_POINT ( 'NONE',  ( -0.3572819248074391996, 0.1213180142433954029, -3.100567304031768057 ) ) ;
#23973=CARTESIAN_POINT ( 'NONE',  ( -0.1677079028045393438, -0.2904160862623708095, 1.953740157480315043 ) ) ;
#23976=CIRCLE ( 'NONE', #25792, 0.5511811023622047445 ) ;
#24004=CARTESIAN_POINT ( 'NONE',  ( 0.5905511811023621549, 0.000000000000000000, 0.9399606299212598381 ) ) ;
#24006=DIRECTION ( 'NONE',  ( 0.000000000000000000, 0.000000000000000000, -1.000000000000000000 ) ) ;
#24009=CARTESIAN_POINT ( 'NONE',  ( 0.5476281405333119912, 0.07214854559198101425, 0.9399606299212598381 ) ) ;
#24027=CARTESIAN_POINT ( 'NONE',  ( -0.3772436174784659646, -0.4300830224589956563, 0.9399606299212598381 ) ) ;
#24036=CARTESIAN_POINT ( 'NONE',  ( -0.06699507805605005306, -0.5085118447796763697, -1.550196850393700920 ) ) ;
#24055=CARTESIAN_POINT ( 'NONE',  ( -0.3001918266902340870, -0.3912931228432089403, -1.569881889763779625 ) ) ;
#24057=CARTESIAN_POINT ( 'NONE',  ( -0.4555658499976152354, -0.06001958459474936169, -1.928289503579151187 ) ) ;
#24060=CARTESIAN_POINT ( 'NONE',  ( -0.5476281405333199848, 0.07214854559197045325, 0.9202755905511811330 ) ) ;
#24063=CARTESIAN_POINT ( 'NONE',  ( -0.3030032861725269200, 0.3454440660767091886, -1.928289503579165620 ) ) ;
#24086=CARTESIAN_POINT ( 'NONE',  ( -0.3606853515406215904, -0.09660931395005714628, -3.115157480314960647 ) ) ;
#24094=VERTEX_POINT ( 'NONE', #22459 ) ;
#24099=SHAPE_DEFINITION_REPRESENTATION ( #22464, #713 ) ;
#24100=CARTESIAN_POINT ( 'NONE',  ( 0.1649135259616801574, 0.4856708409200201637, 1.747047244094488194 ) ) ;
#24106=CARTESIAN_POINT ( 'NONE',  ( 0.09660931395005890876, 0.3606853515406323596, -3.115157480314960647 ) ) ;
#24112=CARTESIAN_POINT ( 'NONE',  ( -0.08676778863011463949, -0.3239425792934414461, 1.953740157480315043 ) ) ;
#24119=CARTESIAN_POINT ( 'NONE',  ( 0.06881554280502791276, 0.1968503937007874127, -3.587858213119324180 ) ) ;
#24122=FACE_OUTER_BOUND ( 'NONE', #3207, .T. ) ;
#24125=CARTESIAN_POINT ( 'NONE',  ( 0.09842519685039370636, 0.2165354330708661457, -3.272637795275590733 ) ) ;
#24134=CARTESIAN_POINT ( 'NONE',  ( -0.3382184156732166436, 0.3855916753051391033, 1.766732283464566899 ) ) ;
#24141=LINE ( 'NONE', #17372, #2237 ) ;
#24151=CARTESIAN_POINT ( 'NONE',  ( -0.5230301363771269196, -0.1775991818008745282, 0.9202755905511811330 ) ) ;
#24159=CARTESIAN_POINT ( 'NONE',  ( 0.3346456692913385988, 2.049113738730807321E-17, 1.973425196850393970 ) ) ;
#24167=CARTESIAN_POINT ( 'NONE',  ( -0.5708661417322835607, 0.000000000000000000, 0.9399606299212598381 ) ) ;
#24195=CARTESIAN_POINT ( 'NONE',  ( -0.3001918266902322552, -0.3912931228432061648, -1.550196850393700920 ) ) ;
#24196=CARTESIAN_POINT ( 'NONE',  ( -0.3454440660767502114, -0.3030032861725112103, -1.928289503579147635 ) ) ;
#24220=DIRECTION ( 'NONE',  ( -1.000000000000000000, 0.000000000000000000, 0.000000000000000000 ) ) ;
#24221=CARTESIAN_POINT ( 'NONE',  ( 0.3267488823401797360, -0.1886891683788832486, -3.100567304031763172 ) ) ;
#24226=CARTESIAN_POINT ( 'NONE',  ( -0.3024344094364737612, -0.3935368318888682881, -1.569881889763779403 ) ) ;
#24228=CARTESIAN_POINT ( 'NONE',  ( -0.3030032861724965554, -0.3454440660767394422, -1.928289503579165620 ) ) ;
#24235=CARTESIAN_POINT ( 'NONE',  ( -0.5118110236220472231, 3.201384367575308305E-17, 1.766732283464566899 ) ) ;
#24236=CARTESIAN_POINT ( 'NONE',  ( -0.4069448477556031341, -0.3121994997598085408, 1.747047244094488194 ) ) ;
#24239=ORIENTED_EDGE ( 'NONE', *, *, #16442, .T. ) ;
#24240=CARTESIAN_POINT ( 'NONE',  ( 0.2272836761397793726, 0.2962590301041582164, -3.115157480314960647 ) ) ;
#24243=CARTESIAN_POINT ( 'NONE',  ( -0.3324885138898230341, 0.04380447413659110945, 1.953740157480315043 ) ) ;
#24254=CIRCLE ( 'NONE', #21098, 0.5118110236220472231 ) ;
#24258=CARTESIAN_POINT ( 'NONE',  ( -0.3074993854542726890, 0.1775730735577450703, 1.953740157480315043 ) ) ;
#24266=EDGE_CURVE ( 'NONE', #18491, #22996, #8920, .T. ) ;
#24274=CARTESIAN_POINT ( 'NONE',  ( -0.3765118517642103702, 0.04928528614549729236, -3.100567304031763616 ) ) ;
#24280=CARTESIAN_POINT ( 'NONE',  ( 0.5511811023622048555, -0.03607471876262468430, 0.9399606299212598381 ) ) ;
#24284=CARTESIAN_POINT ( 'NONE',  ( 0.000000000000000000, 0.000000000000000000, 1.747047244094488194 ) ) ;
#24293=CARTESIAN_POINT ( 'NONE',  ( 0.3543307086614173596, 0.02319089060379041917, 1.953740157480315043 ) ) ;
#24296=CARTESIAN_POINT ( 'NONE',  ( 0.3772436174784756235, 0.4300830224589536899, 0.9399606299212598381 ) ) ;
#24297=CARTESIAN_POINT ( 'NONE',  ( 0.4472135058506041538, -0.2577577458591220338, 1.766732283464566455 ) ) ;
#24321=CARTESIAN_POINT ( 'NONE',  ( -0.1078280746904044657, 0.3175540113612282389, 1.973425196850393970 ) ) ;
#24322=CARTESIAN_POINT ( 'NONE',  ( 0.4763861460130704994, -0.1275996891957771051, -1.550196850393700920 ) ) ;
#24324=CARTESIAN_POINT ( 'NONE',  ( -0.4121342552748326060, -0.2031943647053980340, -1.928289503579156960 ) ) ;
#24326=CARTESIAN_POINT ( 'NONE',  ( 0.07214854559196579031, 0.5476281405333208729, 0.9202755905511811330 ) ) ;
#24330=AXIS2_PLACEMENT_3D ( 'NONE', #21478, #49, #23476 ) ;
#24332=CARTESIAN_POINT ( 'NONE',  ( 0.2796934465393868807, 0.3645739570812638330, -1.928289503579156072 ) ) ;
#24337=CARTESIAN_POINT ( 'NONE',  ( -2.685748425196850164E-17, 0.000000000000000000, -1.894685039405410665 ) ) ;
#24356=CARTESIAN_POINT ( 'NONE',  ( 0.09762295995069844579, 0.3644697409450269321, -3.100567304031763172 ) ) ;
#24369=CARTESIAN_POINT ( 'NONE',  ( 0.4441657790108421988, 0.2564944395515498798, 1.747047244094488194 ) ) ;
#24373=CARTESIAN_POINT ( 'NONE',  ( -0.3726024258163779246, 0.000000000000000000, -3.115157480314960647 ) ) ;
#24377=CARTESIAN_POINT ( 'NONE',  ( 0.2904160862623607620, -0.1677079028045494191, 1.953740157480315043 ) ) ;
#24380=CARTESIAN_POINT ( 'NONE',  ( 0.5511811023622047445, 3.414809992080329023E-17, 0.9202755905511811330 ) ) ;
#24383=ORIENTED_EDGE ( 'NONE', *, *, #7028, .T. ) ;
#24384=CARTESIAN_POINT ( 'NONE',  ( -0.4527559054764770385, 0.000000000000000000, -1.934055118110236338 ) ) ;
#24385=CARTESIAN_POINT ( 'NONE',  ( -0.07874015748031511219, 0.1968503937007874127, -3.548228346456693050 ) ) ;
#24388=CARTESIAN_POINT ( 'NONE',  ( -0.4921259842519685179, 3.013402556957069934E-17, -1.569881889763779625 ) ) ;
#24391=ADVANCED_FACE ( 'NONE', ( #770 ), #17964, .F. ) ;
#24399=CARTESIAN_POINT ( 'NONE',  ( 0.4612490782035170156, 0.2663596103035609786, 1.747047244094488194 ) ) ;
#24411=CARTESIAN_POINT ( 'NONE',  ( 0.1275996891957681401, 0.4763861460130344172, -1.569881889763779625 ) ) ;
#24415=CARTESIAN_POINT ( 'NONE',  ( 0.3362148458988509225, -0.4382482975804891101, 0.9399606299212598381 ) ) ;
#24423=EDGE_CURVE ( 'NONE', #18589, #5007, #5486, .T. ) ;
#24448=CARTESIAN_POINT ( 'NONE',  ( 0.2564944395535760924, 0.4441657790094617475, -1.550196850393700920 ) ) ;
#24450=CARTESIAN_POINT ( 'NONE',  ( 0.06001958459474798779, 0.4555658499976080189, -1.928289503579158515 ) ) ;
#24453=CARTESIAN_POINT ( 'NONE',  ( -0.4954197419817713000, -0.2442565704126117565, 0.9202755905511811330 ) ) ;
#24458=CARTESIAN_POINT ( 'NONE',  ( -0.2466292688015201129, 0.4270824798167635050, -1.569881889763779625 ) ) ;
#24470=ORIENTED_EDGE ( 'NONE', *, *, #19376, .F. ) ;
#24472=CARTESIAN_POINT ( 'NONE',  ( 0.2161891097063337874, 0.2816986811834100157, 1.953740157480314599 ) ) ;
#24474=CARTESIAN_POINT ( 'NONE',  ( -0.1458850421962728516, -0.4296318976990441407, -1.934055118110236338 ) ) ;
#24487=CARTESIAN_POINT ( 'NONE',  ( -0.09762295995069376897, -0.3644697409450285974, -3.100567304031760951 ) ) ;
#24490=CARTESIAN_POINT ( 'NONE',  ( -0.2228126397719833174, 0.3858397471888795893, -1.934055118110236338 ) ) ;
#24492=CARTESIAN_POINT ( 'NONE',  ( -0.2031943647053778002, -0.4121342552748231136, -1.928289503579173614 ) ) ;
#24498=CARTESIAN_POINT ( 'NONE',  ( -0.4954415918530866159, 0.1327036767659691974, 1.747047244094488194 ) ) ;
#24502=CARTESIAN_POINT ( 'NONE',  ( -0.2836590635674538508, 0.2488091035917008864, -3.100567304031763172 ) ) ;
#24516=CARTESIAN_POINT ( 'NONE',  ( 0.02909913904662007542, 0.4446020952038907681, -1.934055118110236338 ) ) ;
#24528=CARTESIAN_POINT ( 'NONE',  ( 0.3346456692913385433, -0.04380501567505458438, 1.973425196850393526 ) ) ;
#24530=CARTESIAN_POINT ( 'NONE',  ( -0.2161381151962937508, 0.2817310484609270027, 1.953740157480315043 ) ) ;
#24531=DIRECTION ( 'NONE',  ( 0.000000000000000000, 0.000000000000000000, -1.000000000000000000 ) ) ;
#24535=CARTESIAN_POINT ( 'NONE',  ( 0.4069448477556011912, 0.3121994997598430133, 1.766732283464566899 ) ) ;
#24542=ORIENTED_EDGE ( 'NONE', *, *, #10729, .F. ) ;
#24545=CARTESIAN_POINT ( 'NONE',  ( 0.3001918266902144361, -0.3912931228432220410, -1.569881889763779625 ) ) ;
#24550=CARTESIAN_POINT ( 'NONE',  ( 0.4152525734086595088, -0.3642352168757885811, 0.9399606299212598381 ) ) ;
#24560=EDGE_CURVE ( 'NONE', #21933, #724, #16428, .T. ) ;
#24564=CARTESIAN_POINT ( 'NONE',  ( 0.2660793235464290474, -0.2041304421298306693, 1.953740157480315043 ) ) ;
#24565=UNCERTAINTY_MEASURE_WITH_UNIT (LENGTH_MEASURE( 1.000000000000000082E-05 ), #17236, 'distance_accuracy_value', 'NONE') ;
#24583=CARTESIAN_POINT ( 'NONE',  ( 0.07870736599822261703, 0.1968503937007382021, -3.608715228723502921 ) ) ;
#24584=CARTESIAN_POINT ( 'NONE',  ( -0.5118110236220473341, 0.03361326524566096707, -1.550196850393701142 ) ) ;
#24593=EDGE_LOOP ( 'NONE', ( #27205, #20246, #25675, #9229 ) ) ;
#24594=CARTESIAN_POINT ( 'NONE',  ( -0.2041304421298429650, -0.2660793235464223860, 1.973425196850393970 ) ) ;
#24595=CARTESIAN_POINT ( 'NONE',  ( -0.2180862235769588653, -0.4423390553432484107, -1.550196850393700920 ) ) ;
#24611=CYLINDRICAL_SURFACE ( 'NONE', #11399, 0.3346456692913385988 ) ;
#24612=ORIENTED_EDGE ( 'NONE', *, *, #18615, .T. ) ;
#24613=CARTESIAN_POINT ( 'NONE',  ( -0.1570773243922992946, 0.3184597017669829055, 1.953740157480315043 ) ) ;
#24616=CARTESIAN_POINT ( 'NONE',  ( -0.3411003281197191872, -0.2991932138496762317, -1.934055118110236338 ) ) ;
#24619=CARTESIAN_POINT ( 'NONE',  ( 0.006559182411507800264, 0.3149605050255358529, -3.174212998091514137 ) ) ;
#24624=CARTESIAN_POINT ( 'NONE',  ( -0.3995913070739969819, -0.1970988029421826826, -1.934055118110236338 ) ) ;
#24625=CARTESIAN_POINT ( 'NONE',  ( 0.3644697409450285974, -0.09762295995069371346, -3.100567304031760951 ) ) ;
#24630=CARTESIAN_POINT ( 'NONE',  ( 0.3996230174612959707, 0.1970259548082022305, -1.934055118110236338 ) ) ;
#24632=CARTESIAN_POINT ( 'NONE',  ( -0.3645739570812778219, -0.2796934465393718927, -1.928289503579152742 ) ) ;
#24638=CARTESIAN_POINT ( 'NONE',  ( -0.4441657790107820802, -0.2564944395515947884, 1.747047244094488194 ) ) ;
#24656=CARTESIAN_POINT ( 'NONE',  ( 0.07874015748031489015, 0.1968503937007874127, -3.272637795275590733 ) ) ;
#24662=LINE ( 'NONE', #3765, #16217 ) ;
#24665=CARTESIAN_POINT ( 'NONE',  ( -0.3362336590883616139, -0.1141709026133614219, 1.953740157480315043 ) ) ;
#24674=CARTESIAN_POINT ( 'NONE',  ( 0.5314960629921260393, 0.03478633594540018331, 1.747047244094488194 ) ) ;
#24676=CARTESIAN_POINT ( 'NONE',  ( 0.4856708409200646281, 0.1649135259617043880, 1.766732283464566899 ) ) ;
#24677=VERTEX_POINT ( 'NONE', #1269 ) ;
#24682=CARTESIAN_POINT ( 'NONE',  ( -0.4417361510194065533, 0.05819755867303653962, -1.934055118110236338 ) ) ;
#24686=CARTESIAN_POINT ( 'NONE',  ( -0.03220957031754000111, 0.4921259842519685179, -1.569881889763779625 ) ) ;
#24689=CARTESIAN_POINT ( 'NONE',  ( 0.2442565704126313797, -0.4954197419817796266, 0.9399606299212598381 ) ) ;
#24722=CARTESIAN_POINT ( 'NONE',  ( -0.01288382760289888060, 0.1968503937007873850, -3.646653543307086576 ) ) ;
#24725=CARTESIAN_POINT ( 'NONE',  ( -0.07874015748031495954, 0.1968503937007874127, -3.364501312335958172 ) ) ;
#24727=CONICAL_SURFACE ( 'NONE', #14848, 0.4724409448465559103, 0.7853981642948979491 ) ;
#24737=CARTESIAN_POINT ( 'NONE',  ( 0.2521176338356569957, 0.2211428102655756955, 1.973425196850393970 ) ) ;
#24738=CARTESIAN_POINT ( 'NONE',  ( 0.4921259842519685179, 0.03220957031754003580, -1.550196850393700920 ) ) ;
#24741=CARTESIAN_POINT ( 'NONE',  ( 0.3642352168757561071, 0.4152525734086270348, 0.9202755905511811330 ) ) ;
#24747=CARTESIAN_POINT ( 'NONE',  ( 0.4423390553432540173, 0.2180862235769270852, -1.569881889763779625 ) ) ;
#24755=EDGE_LOOP ( 'NONE', ( #17678, #20280 ) ) ;
#24756=DIRECTION ( 'NONE',  ( 1.000000000000000000, 0.000000000000000000, 0.000000000000000000 ) ) ;
#24759=CARTESIAN_POINT ( 'NONE',  ( -0.2669897767696617907, 0.2341075107471362882, 1.953740157480315487 ) ) ;
#24761=CARTESIAN_POINT ( 'NONE',  ( -0.1173917140416368271, -0.4382752542996092293, -1.934055118110236338 ) ) ;
#24772=ORIENTED_EDGE ( 'NONE', *, *, #3062, .F. ) ;
#24773=CARTESIAN_POINT ( 'NONE',  ( -0.2993674444872274076, -0.2296683860596782090, -3.100567304031764060 ) ) ;
#24775=CARTESIAN_POINT ( 'NONE',  ( 0.2362017869179295071, -0.2693781226336162127, -3.115157480314961091 ) ) ;
#24779=CARTESIAN_POINT ( 'NONE',  ( -0.3599896729929454864, 0.2761764805255169652, -1.934055118110236338 ) ) ;
#24785=CARTESIAN_POINT ( 'NONE',  ( 0.03349795313264414959, -0.5118110236220472231, 1.747047244094488194 ) ) ;
#24791=CARTESIAN_POINT ( 'NONE',  ( 0.04928467685643810742, 0.3740848232703744003, -3.100567304031763172 ) ) ;
#24799=CARTESIAN_POINT ( 'NONE',  ( 0.2712027394948692827, 0.3535065162672724748, -1.934055118110236338 ) ) ;
#24821=EDGE_LOOP ( 'NONE', ( #5480, #2879, #23213, #11229, #21892 ) ) ;
#24823=CARTESIAN_POINT ( 'NONE',  ( -0.4777261797697572310, -0.2355331214654124150, 1.747047244094488194 ) ) ;
#24826=CARTESIAN_POINT ( 'NONE',  ( -0.4954415918530846175, -0.1327036767659680039, 1.766732283464566899 ) ) ;
#24830=ADVANCED_FACE ( 'NONE', ( #25414, #15119 ), #23728, .T. ) ;
#24833=EDGE_LOOP ( 'NONE', ( #8176, #12726, #10988, #18461, #2084 ) ) ;
#24835=CARTESIAN_POINT ( 'NONE',  ( 0.3707612262533033776, -0.3252100150720387273, -1.569881889763779625 ) ) ;
#24850=CARTESIAN_POINT ( 'NONE',  ( -0.2521176338356424518, 0.2211428102655600414, 1.953740157480315043 ) ) ;
#24855=CARTESIAN_POINT ( 'NONE',  ( -0.09842519685039370636, 0.5905905511811023745, -3.548228346456693050 ) ) ;
#24858=VECTOR ( 'NONE', #11707, 39.37007874015748143 ) ;
#24861=ORIENTED_EDGE ( 'NONE', *, *, #23798, .F. ) ;
#24863=ORIENTED_EDGE ( 'NONE', *, *, #2871, .T. ) ;
#24866=CARTESIAN_POINT ( 'NONE',  ( -0.06048688226689268727, 0.1968503937007873850, -3.626935712454880001 ) ) ;
#24875=VECTOR ( 'NONE', #2712, 39.37007874015748854 ) ;
#24880=CARTESIAN_POINT ( 'NONE',  ( -0.3324885138898239778, 0.04380447413658877104, 1.973425196850393970 ) ) ;
#24882=CARTESIAN_POINT ( 'NONE',  ( -0.4954415918535808872, -0.1327036767636090853, -1.550196850393700920 ) ) ;
#24884=CARTESIAN_POINT ( 'NONE',  ( 0.1442704874421230632, 0.5368353335967094297, 0.9202755905511812440 ) ) ;
#24885=CARTESIAN_POINT ( 'NONE',  ( 0.2442565704126255510, -0.4954197419817655823, 0.9202755905511811330 ) ) ;
#24903=ORIENTED_EDGE ( 'NONE', *, *, #26454, .T. ) ;
#24920=CARTESIAN_POINT ( 'NONE',  ( 0.02909913904661943010, -0.4446020952038907681, -1.934055118110236338 ) ) ;
#24932=EDGE_CURVE ( 'NONE', #21621, #10030, #8137, .T. ) ;
#24934=AXIS2_PLACEMENT_3D ( 'NONE', #14165, #18364, #23631 ) ;
#24938=CARTESIAN_POINT ( 'NONE',  ( 0.3349573549949902418, -0.2938049579018460755, -1.934055118110236338 ) ) ;
#24943=CARTESIAN_POINT ( 'NONE',  ( 0.3213305936751379432, -0.1584254766472190656, -3.115157480314960647 ) ) ;
#24949=ADVANCED_FACE ( 'NONE', ( #11537 ), #5614, .T. ) ;
#24963=CARTESIAN_POINT ( 'NONE',  ( 0.5144970376936013334, 0.1378076643338890239, 1.747047244094488194 ) ) ;
#24964=CARTESIAN_POINT ( 'NONE',  ( -0.2564944395515788567, -0.4441657790107717552, 1.766732283464566899 ) ) ;
#24976=CARTESIAN_POINT ( 'NONE',  ( 0.4921259842519685179, 0.03220957031754003580, -1.569881889763779625 ) ) ;
#24978=EDGE_LOOP ( 'NONE', ( #22745, #19939, #10302, #20647 ) ) ;
#24993=CARTESIAN_POINT ( 'NONE',  ( -0.06001958459474839719, -0.4555658499976154574, -1.928289503579151187 ) ) ;
#24995=CARTESIAN_POINT ( 'NONE',  ( -0.1288129352161812291, 0.4793172621399193756, -1.569881889763779848 ) ) ;
#25003=CARTESIAN_POINT ( 'NONE',  ( -0.1649135259639108730, -0.4856708409191554665, -1.550196850393700920 ) ) ;
#25022=CARTESIAN_POINT ( 'NONE',  ( 0.5085118447796558305, 0.06699507805605002531, -1.550196850393700920 ) ) ;
#25023=CARTESIAN_POINT ( 'NONE',  ( -0.4407612517155324872, 0.3387265385688508212, 0.9202755905511812440 ) ) ;
#25027=CARTESIAN_POINT ( 'NONE',  ( -0.5511811023622047445, 0.000000000000000000, 0.9202755905511811330 ) ) ;
#25036=ORIENTED_EDGE ( 'NONE', *, *, #15606, .T. ) ;
#25045=DIRECTION ( 'NONE',  ( 0.000000000000000000, 0.000000000000000000, 1.000000000000000000 ) ) ;
#25061=CARTESIAN_POINT ( 'NONE',  ( 0.2228126397719881469, 0.3858397471888846408, -1.934055118110236338 ) ) ;
#25067=EDGE_LOOP ( 'NONE', ( #399, #6227, #10348, #25338 ) ) ;
#25069=CARTESIAN_POINT ( 'NONE',  ( 0.09842519685039366473, 0.1968503937007873850, -3.272637795275590733 ) ) ;
#25071=CARTESIAN_POINT ( 'NONE',  ( 0.5118110236220472231, 0.000000000000000000, 1.747047244094488194 ) ) ;
#25075=CARTESIAN_POINT ( 'NONE',  ( 0.1886891683788904650, 0.3267488823401754061, -3.100567304031762284 ) ) ;
#25080=ORIENTED_EDGE ( 'NONE', *, *, #18832, .T. ) ;
#25089=CARTESIAN_POINT ( 'NONE',  ( -0.1791601451668923262, -0.3102476824511486986, -3.115157480314960647 ) ) ;
#25095=FACE_OUTER_BOUND ( 'NONE', #22289, .T. ) ;
#25098=EDGE_CURVE ( 'NONE', #8508, #16690, #27348, .T. ) ;
#25100=CARTESIAN_POINT ( 'NONE',  ( 0.07462150385400743990, 0.5672083774005964862, 0.9399606299212601712 ) ) ;
#25120=CARTESIAN_POINT ( 'NONE',  ( 0.1275996891957845991, -0.4763861460130774939, -1.550196850393700920 ) ) ;
#25129=B_SPLINE_SURFACE_WITH_KNOTS ( 'NONE', 2, 3, ( 
 ( #20877, #3486, #27383, #20599, #1251, #22866, #8036, #18314, #16643, #25254, #9715, #7751, #14550, #16364, #14256, #17063, #25539, #4070, #16782, #23575, #14961, #6330, #10697, #27665, #277, #10975, #8313, #4209, #1803, #14, #2083, #19601, #8716, #10413, #12543, #144, #21162, #8580, #19312, #12813, #16930, #25680, #6200, #17198, #6060, #21717, #14829, #25817, #6465, #25394, #2214, #23437, #15098, #14692, #12676, #10837, #19030, #21579, #21303, #1941, #17338, #23709, #10549, #4344, #19171, #12949 ),
 ( #19452, #27806, #23297, #2346, #21444, #25954, #6605, #15231, #23844, #13092, #3925, #13635, #5153, #26352, #20279, #2886, #9113, #17732, #17606, #24106, #8849, #15638, #7017, #24240, #2748, #19732, #17472, #3021, #400, #4881, #21851, #20000, #22120, #11657, #794, #2490, #4604, #20136, #13225, #651, #11382, #13495, #8982, #521, #26220, #9241, #26086, #13780, #6880, #17859, #26482, #6748, #22255, #15507, #7148, #15381, #4741, #11519, #11111, #9382, #13363, #21989, #17989, #15770, #2621, #24373 ),
 ( #5014, #26625, #7280, #11243, #23969, #22399, #19867, #15899, #24502, #27206, #16462, #20835, #12361, #5740, #25211, #18420, #937, #12222, #24791, #26919, #22828, #16047, #25075, #7563, #3166, #9525, #11799, #13924, #7855, #16190, #3591, #18708, #14357, #10098, #18278, #14508, #5454, #14067, #20419, #22969, #12082, #3304, #5880, #23110, #18125, #27066, #1081, #22679, #11947, #26769, #7716, #20566, #1217, #1487, #9821, #16328, #3741, #7417, #9677, #5302, #14219, #22541, #5591, #27344, #3446, #20702 ) ),
 .UNSPECIFIED., .F., .T., .F.,
 ( 3, 3 ),
 ( 4, 2, 2, 2, 2, 2, 2, 2, 2, 2, 2, 2, 2, 2, 2, 2, 2, 2, 2, 2, 2, 2, 2, 2, 2, 2, 2, 2, 2, 2, 2, 2, 4 ),
 ( 0.000000000000000000, 1.000000000000000000 ),
 ( 0.000000000000000000, 0.1963495408493620697, 0.3926990816987241395, 0.5890486225480862092, 0.7853981633974482790, 0.9817477042468103487, 1.178097245096172418, 1.374446785945534488, 1.570796326794896558, 1.767145867644258628, 1.963495408493620697, 2.159844949342982545, 2.356194490192344837, 2.552544031041707129, 2.748893571891068976, 2.945243112740430824, 3.141592653589793116, 3.337942194439155408, 3.534291735288517255, 3.730641276137879103, 3.926990816987241395, 4.123340357836603687, 4.319689898685965090, 4.516039439535327382, 4.712388980384689674, 4.908738521234051966, 5.105088062083414258, 5.301437602932775661, 5.497787143782137953, 5.694136684631500245, 5.890486225480861648, 6.086835766330223940, 6.283185307179586232 ),
 .UNSPECIFIED. ) ;
#25154=EDGE_CURVE ( 'NONE', #3990, #20420, #2476, .T. ) ;
#25156=CARTESIAN_POINT ( 'NONE',  ( -0.4599980997183342191, -0.2268967137092737507, -1.550196850393701364 ) ) ;
#25165=CARTESIAN_POINT ( 'NONE',  ( -0.5511811023622048555, -0.03607471876259069760, 0.9399606299212598381 ) ) ;
#25179=CARTESIAN_POINT ( 'NONE',  ( 0.03488411621168054089, -0.5314946440730492494, 1.747047244094488416 ) ) ;
#25186=CARTESIAN_POINT ( 'NONE',  ( -0.06045787421035515169, 0.3092457124703104632, -3.193900699392901554 ) ) ;
#25198=CARTESIAN_POINT ( 'NONE',  ( -0.3574975638436101444, 0.000000000000000000, -3.115157480314960647 ) ) ;
#25201=CARTESIAN_POINT ( 'NONE',  ( -0.3535065162672666461, -0.2712027394948650083, -1.934055118110236338 ) ) ;
#25204=CARTESIAN_POINT ( 'NONE',  ( -0.4585215200179055817, 0.000000000000000000, -1.928289503579156516 ) ) ;
#25209=CARTESIAN_POINT ( 'NONE',  ( -0.03478633594543723007, 0.5314960629921260393, 1.747047244094488194 ) ) ;
#25211=CARTESIAN_POINT ( 'NONE',  ( -0.09762295995069900090, 0.3644697409450268766, -3.100567304031763172 ) ) ;
#25214=CARTESIAN_POINT ( 'NONE',  ( -0.2341512108694376038, 0.2669480828848188603, 1.953740157480315043 ) ) ;
#25215=CARTESIAN_POINT ( 'NONE',  ( 0.02576258753921166489, 0.2165354330708661457, -3.644091798679236494 ) ) ;
#25219=AXIS2_PLACEMENT_3D ( 'NONE', #27365, #14239, #22845 ) ;
#25222=CARTESIAN_POINT ( 'NONE',  ( -0.09855118063547688156, -0.3667122560601323022, -3.100567304031763616 ) ) ;
#25223=CARTESIAN_POINT ( 'NONE',  ( -0.4152525734085961151, -0.3642352168756899933, 0.9399606299212598381 ) ) ;
#25225=ORIENTED_EDGE ( 'NONE', *, *, #522, .T. ) ;
#25243=CARTESIAN_POINT ( 'NONE',  ( 0.3483099419446107348, 0.4538399017592875118, 0.9399606299212600602 ) ) ;
#25246=AXIS2_PLACEMENT_3D ( 'NONE', #6037, #21141, #10396 ) ;
#25249=CARTESIAN_POINT ( 'NONE',  ( 0.09842519685039362309, 0.2165354330708660902, -3.561112174596413826 ) ) ;
#25251=CARTESIAN_POINT ( 'NONE',  ( 0.3382184156732089830, -0.3855916753051465973, 1.766732283464566899 ) ) ;
#25254=CARTESIAN_POINT ( 'NONE',  ( -0.2362439534887433856, 0.2693339498142315325, -3.115157480314960647 ) ) ;
#25258=CARTESIAN_POINT ( 'NONE',  ( -0.3007905576423877680, -0.1482986320106428613, 1.973425196850393970 ) ) ;
#25275=VERTEX_POINT ( 'NONE', #19014 ) ;
#25288=ORIENTED_EDGE ( 'NONE', *, *, #5693, .T. ) ;
#25289=( NAMED_UNIT ( * ) SI_UNIT ( $, .STERADIAN. ) SOLID_ANGLE_UNIT ( ) ) ;
#25294=CARTESIAN_POINT ( 'NONE',  ( -0.4152525734086684461, 0.3642352168757148068, 0.9202755905511811330 ) ) ;
#25307=CARTESIAN_POINT ( 'NONE',  ( 0.4442189740298561618, -0.2564173815256141631, -1.550196850393701364 ) ) ;
#25311=CARTESIAN_POINT ( 'NONE',  ( 0.1482986320106464417, 0.3007905576423925420, 1.953740157480315043 ) ) ;
#25312=CARTESIAN_POINT ( 'NONE',  ( -0.3855916753034467903, -0.3382184156749090675, -1.550196850393700920 ) ) ;
#25314=CARTESIAN_POINT ( 'NONE',  ( -0.4539000224941007744, 0.3482225189667277343, 0.9399606299212598381 ) ) ;
#25318=CARTESIAN_POINT ( 'NONE',  ( 0.1711654736996354453, 0.5043865966253979760, 1.747047244094488416 ) ) ;
#25322=CARTESIAN_POINT ( 'NONE',  ( -0.4921259842519975503, -0.03220957031763956036, -1.550196850393700920 ) ) ;
#25327=CARTESIAN_POINT ( 'NONE',  ( 0.4776900717922462625, -0.2356240016486843558, 1.747047244094488194 ) ) ;
#25331=ORIENTED_EDGE ( 'NONE', *, *, #22533, .T. ) ;
#25338=ORIENTED_EDGE ( 'NONE', *, *, #19037, .F. ) ;
#25340=CARTESIAN_POINT ( 'NONE',  ( 0.2991932138496291582, 0.3411003281196904324, -1.934055118110236338 ) ) ;
#25346=ORIENTED_EDGE ( 'NONE', *, *, #19844, .T. ) ;
#25349=CARTESIAN_POINT ( 'NONE',  ( -0.5043504886477528926, -0.1712563538833036247, 1.747047244094488194 ) ) ;
#25357=CARTESIAN_POINT ( 'NONE',  ( 0.05811937031584422236, 0.4417502570508218263, -1.934055118110236560 ) ) ;
#25359=CARTESIAN_POINT ( 'NONE',  ( 0.3362336590883814313, -0.1141709026133623794, 1.953740157480315043 ) ) ;
#25366=CARTESIAN_POINT ( 'NONE',  ( 0.2529800193559378352, 0.5131133041953702678, 0.9399606299212598381 ) ) ;
#25372=CARTESIAN_POINT ( 'NONE',  ( 0.3102476824511487541, -0.1791601451668820011, -3.115157480314960647 ) ) ;
#25375=CYLINDRICAL_SURFACE ( 'NONE', #25246, 0.4921259842519685179 ) ;
#25376=VECTOR ( 'NONE', #22552, 39.37007874015748143 ) ;
#25382=CARTESIAN_POINT ( 'NONE',  ( -0.07462095020359073294, 0.5672055940106845995, 0.9399606299212600602 ) ) ;
#25384=AXIS2_PLACEMENT_3D ( 'NONE', #15486, #17452, #24220 ) ;
#25388=CARTESIAN_POINT ( 'NONE',  ( 0.1378076643338767004, -0.5144970376935934508, 1.747047244094488194 ) ) ;
#25391=CARTESIAN_POINT ( 'NONE',  ( 0.3855916753051394363, 0.3382184156732163660, 1.747047244094488194 ) ) ;
#25394=CARTESIAN_POINT ( 'NONE',  ( -0.02339816079119156136, -0.3574975638436101444, -3.115157480314960647 ) ) ;
#25401=CARTESIAN_POINT ( 'NONE',  ( -0.2211428102655755012, 0.2521176338356572177, 1.973425196850393970 ) ) ;
#25404=CARTESIAN_POINT ( 'NONE',  ( -0.3252100150720236837, -0.3707612262533185321, -1.550196850393700920 ) ) ;
#25414=FACE_BOUND ( 'NONE', #24821, .T. ) ;
#25435=CARTESIAN_POINT ( 'NONE',  ( -0.4441657790094409863, -0.2564944395535778687, -1.550196850393700920 ) ) ;
#25439=CARTESIAN_POINT ( 'NONE',  ( -0.5230301363771427958, 0.1775991818008358647, 0.9202755905511811330 ) ) ;
#25441=DIRECTION ( 'NONE',  ( 0.000000000000000000, 0.000000000000000000, 1.000000000000000000 ) ) ;
#25451=CARTESIAN_POINT ( 'NONE',  ( 0.1677079028045370679, 0.2904160862623488826, 1.953740157480315043 ) ) ;
#25452=CARTESIAN_POINT ( 'NONE',  ( 0.4856708409191126674, 0.1649135259639225026, -1.550196850393700920 ) ) ;
#25457=CARTESIAN_POINT ( 'NONE',  ( -0.07214854559198104200, 0.5476281405333119912, 0.9399606299212598381 ) ) ;
#25460=CARTESIAN_POINT ( 'NONE',  ( 0.5511811023268710086, 6.991093931924045359E-17, 1.747047244094488194 ) ) ;
#25466=ORIENTED_EDGE ( 'NONE', *, *, #19844, .F. ) ;
#25469=CARTESIAN_POINT ( 'NONE',  ( 0.3382184156749452608, -0.3855916753034395184, -1.550196850393700920 ) ) ;
#25473=CARTESIAN_POINT ( 'NONE',  ( -0.1379038425970198212, -0.5144793533649091311, 1.747047244094487972 ) ) ;
#25474=CARTESIAN_POINT ( 'NONE',  ( 0.3856568748495315946, 0.3381512095064278522, -1.550196850393701364 ) ) ;
#25490=CARTESIAN_POINT ( 'NONE',  ( 0.4763861460130341396, -0.1275996891957698887, -1.569881889763779625 ) ) ;
#25492=CARTESIAN_POINT ( 'NONE',  ( -0.3645739570812708275, 0.2796934465393700053, -1.928289503579159625 ) ) ;
#25501=CARTESIAN_POINT ( 'NONE',  ( -0.06957181182499248828, -0.5280699926562971713, 1.747047244094488194 ) ) ;
#25506=CARTESIAN_POINT ( 'NONE',  ( -0.4303681241740391905, 0.1153557615289447225, -1.934055118110236338 ) ) ;
#25508=CARTESIAN_POINT ( 'NONE',  ( -0.09187177619658792871, 0.3429980251342187314, 1.953740157480315043 ) ) ;
#25518=AXIS2_PLACEMENT_3D ( 'NONE', #22275, #11678, #20300 ) ;
#25532=ORIENTED_EDGE ( 'NONE', *, *, #6335, .T. ) ;
#25535=CARTESIAN_POINT ( 'NONE',  ( 0.02576258704323635199, 0.2165354330708661457, -3.644091798884676159 ) ) ;
#25539=CARTESIAN_POINT ( 'NONE',  ( -0.02339816079119098197, 0.3574975638436101444, -3.115157480314960647 ) ) ;
#25541=PLANE ( 'NONE',  #16392 ) ;
#25545=CARTESIAN_POINT ( 'NONE',  ( -0.1482986320106437217, -0.3007905576423873795, 1.973425196850393970 ) ) ;
#25549=CARTESIAN_POINT ( 'NONE',  ( 0.2466292688015316592, -0.4270824798167792147, -1.550196850393700920 ) ) ;
#25559=B_SPLINE_CURVE_WITH_KNOTS ( 'NONE', 3,
 ( #7779, #5516, #10298, #22742, #3365, #12012, #16386, #24995, #20766, #6356, #12840, #10441, #27689, #25704, #17227, #21191, #23605, #25844 ),
 .UNSPECIFIED., .F., .F.,
 ( 4, 2, 2, 2, 2, 2, 2, 2, 4 ),
 ( 0.000000000000000000, 0.06249999999999995837, 0.1249999999999999167, 0.1874999999999999167, 0.2499999999999999445, 0.3124999999999999445, 0.3749999999999999445, 0.4375000000000000000, 0.5000000000000000000 ),
 .UNSPECIFIED. ) ;
#25569=CARTESIAN_POINT ( 'NONE',  ( -0.4006498629591500604, 0.2309201403895328464, -1.928289503579156960 ) ) ;
#25570=DIRECTION ( 'NONE',  ( -0.000000000000000000, -0.000000000000000000, -1.000000000000000000 ) ) ;
#25572=CARTESIAN_POINT ( 'NONE',  ( 0.01030706208231648401, 0.1968503937007873850, -3.193897637795275912 ) ) ;
#25582=CARTESIAN_POINT ( 'NONE',  ( 0.4954197419817656933, 0.2442565704126251624, 0.9202755905511811330 ) ) ;
#25593=DIRECTION ( 'NONE',  ( 0.000000000000000000, 0.000000000000000000, -1.000000000000000000 ) ) ;
#25598=CARTESIAN_POINT ( 'NONE',  ( 0.3642352168757886366, 0.4152525734086595088, 0.9399606299212598381 ) ) ;
#25602=B_SPLINE_SURFACE_WITH_KNOTS ( 'NONE', 2, 3, ( 
 ( #1702, #18785, #16687, #1563, #25439, #27567, #18933, #23344, #25294, #5956, #4250, #14589, #6104, #23193, #12583, #14738, #3823, #21345, #12445, #21057, #1981, #6368, #3971, #10590, #21205, #10453, #19072, #16967, #25582, #6237, #14874, #23482, #4112, #19215, #8481, #17102, #25721, #2530, #2126, #2255, #15550, #23750, #26263, #15139, #17241, #4783, #8759, #8894, #21761, #4648, #10742, #26395, #12992, #13276, #19772, #4925, #10877, #17379, #11152, #19357, #19492, #24151, #4385, #6925, #21622, #25857 ),
 ( #21484, #8622, #56, #6508, #21898, #2392, #13402, #188, #25996, #7058, #6652, #15278, #15422, #438, #9026, #2663, #23888, #11292, #17777, #11021, #4527, #19910, #13131, #17645, #19644, #561, #9158, #317, #17514, #26132, #6787, #24009, #15677, #24280, #16608, #3750, #12229, #23120, #26818, #22442, #24550, #11561, #24415, #10106, #24689, #15945, #10239, #18854, #2790, #11702, #5060, #26671, #20179, #11423, #20324, #7326, #2932, #25223, #840, #5202, #27499, #22164, #16752, #3067, #13681, #9429 ),
 ( #1634, #22301, #981, #3600, #7190, #9567, #20845, #8146, #13828, #18176, #8006, #7466, #16094, #18030, #5749, #13539, #14366, #22980, #1495, #18718, #27354, #25366, #20045, #5892, #14517, #26525, #12370, #20988, #696, #9286, #15808, #17899, #17308, #10951, #1914, #25927, #10525, #17445, #21694, #14663, #10385, #27776, #2321, #17039, #12790, #23683, #27639, #2053, #4317, #255, #25650, #21414, #118, #6304, #23548, #10665, #19287, #6027, #7994, #17175, #25789, #12922, #16902, #23267, #12515, #10813 ) ),
 .UNSPECIFIED., .F., .T., .F.,
 ( 3, 3 ),
 ( 4, 2, 2, 2, 2, 2, 2, 2, 2, 2, 2, 2, 2, 2, 2, 2, 2, 2, 2, 2, 2, 2, 2, 2, 2, 2, 2, 2, 2, 2, 2, 2, 4 ),
 ( 0.000000000000000000, 1.000000000000000000 ),
 ( 0.000000000000000000, 0.1963495408493620697, 0.3926990816987241395, 0.5890486225480862092, 0.7853981633974482790, 0.9817477042468103487, 1.178097245096172418, 1.374446785945534488, 1.570796326794896558, 1.767145867644258628, 1.963495408493620697, 2.159844949342982545, 2.356194490192344837, 2.552544031041707129, 2.748893571891068976, 2.945243112740430824, 3.141592653589793116, 3.337942194439155408, 3.534291735288517255, 3.730641276137879103, 3.926990816987241395, 4.123340357836603687, 4.319689898685965090, 4.516039439535327382, 4.712388980384689674, 4.908738521234051966, 5.105088062083414258, 5.301437602932775661, 5.497787143782137953, 5.694136684631500245, 5.890486225480861648, 6.086835766330223940, 6.283185307179586232 ),
 .UNSPECIFIED. ) ;
#25607=CARTESIAN_POINT ( 'NONE',  ( 0.06699507805604380806, -0.5085118447796470598, -1.550196850393700920 ) ) ;
#25608=CARTESIAN_POINT ( 'NONE',  ( -0.5525886237719659366, -0.1481199686355886558, 0.9399606299212600602 ) ) ;
#25611=CARTESIAN_POINT ( 'NONE',  ( -0.4776874499715845213, -0.2356229156551546411, 1.747047244094488194 ) ) ;
#25628=CARTESIAN_POINT ( 'NONE',  ( 0.05926487674659523808, -0.4498374011143459472, -1.934055118110236338 ) ) ;
#25638=DIRECTION ( 'NONE',  ( 0.000000000000000000, 0.000000000000000000, -1.000000000000000000 ) ) ;
#25641=CARTESIAN_POINT ( 'NONE',  ( -0.3184597017669179020, -0.1570773243923554441, 1.953740157480315043 ) ) ;
#25646=CARTESIAN_POINT ( 'NONE',  ( -0.1141709026133623378, -0.3362336590883613363, 1.953740157480315043 ) ) ;
#25650=CARTESIAN_POINT ( 'NONE',  ( -0.07472527936312729768, -0.5671862884094908130, 0.9399606299212598381 ) ) ;
#25657=CARTESIAN_POINT ( 'NONE',  ( 0.2462256503455907131, -0.2807137536170764003, -3.115157480314960647 ) ) ;
#25662=CARTESIAN_POINT ( 'NONE',  ( 0.4300129863948120024, -0.2478439864030017314, -1.569881889763779625 ) ) ;
#25668=CARTESIAN_POINT ( 'NONE',  ( -0.3483115186085786741, 0.4538422614031236146, 0.9399606299212601712 ) ) ;
#25672=CARTESIAN_POINT ( 'NONE',  ( 0.5118110236220472231, 0.000000000000000000, 1.766732283464566899 ) ) ;
#25673=CARTESIAN_POINT ( 'NONE',  ( -0.3121994997597934973, 0.4069448477556333321, 1.747047244094488194 ) ) ;
#25675=ORIENTED_EDGE ( 'NONE', *, *, #775, .T. ) ;
#25680=CARTESIAN_POINT ( 'NONE',  ( 0.2362439534887394721, -0.2693339498142455213, -3.115157480314960647 ) ) ;
#25685=CARTESIAN_POINT ( 'NONE',  ( 0.3175540113612325133, 0.1078280746903942239, 1.973425196850393970 ) ) ;
#25688=CARTESIAN_POINT ( 'NONE',  ( 0.4423390553432928751, 0.2180862235769577551, -1.550196850393700920 ) ) ;
#25703=CARTESIAN_POINT ( 'NONE',  ( 0.3666644560843329015, 0.2817828961649157526, -1.928289503579156294 ) ) ;
#25704=CARTESIAN_POINT ( 'NONE',  ( 0.3935368318888682326, 0.3024344094364738167, -1.569881889763779625 ) ) ;
#25707=ADVANCED_FACE ( 'NONE', ( #21635 ), #1442, .T. ) ;
#25708=CARTESIAN_POINT ( 'NONE',  ( 0.09842519685039363697, 0.2165354330708661457, -3.272637795275590733 ) ) ;
#25715=EDGE_LOOP ( 'NONE', ( #24903, #23962 ) ) ;
#25721=CARTESIAN_POINT ( 'NONE',  ( 0.5230301363771282519, -0.1775991818008710588, 0.9202755905511811330 ) ) ;
#25727=CYLINDRICAL_SURFACE ( 'NONE', #1879, 0.5118110236220472231 ) ;
#25739=CARTESIAN_POINT ( 'NONE',  ( 0.5511811023622048555, 0.03607471876262481614, 0.9399606299212598381 ) ) ;
#25743=CARTESIAN_POINT ( 'NONE',  ( -0.3102804211135531398, 0.1791085948259530103, -3.115157480314961091 ) ) ;
#25750=CARTESIAN_POINT ( 'NONE',  ( 0.4954415918535722829, 0.1327036767636095571, -1.550196850393700920 ) ) ;
#25755=CARTESIAN_POINT ( 'NONE',  ( -0.5144765700550301135, -0.1379032889622909541, 1.747047244094488194 ) ) ;
#25767=CARTESIAN_POINT ( 'NONE',  ( -0.4921259842519685179, 0.000000000000000000, -1.550196850393700920 ) ) ;
#25769=CARTESIAN_POINT ( 'NONE',  ( 0.2268989272875507057, -0.3929158813954434226, -1.934055118110236338 ) ) ;
#25776=CARTESIAN_POINT ( 'NONE',  ( 0.1712563538833069832, -0.5043504886477723215, 1.747047244094488194 ) ) ;
#25783=CARTESIAN_POINT ( 'NONE',  ( -0.05811992390534824471, 0.4417530401346466129, -1.934055118110236338 ) ) ;
#25786=CARTESIAN_POINT ( 'NONE',  ( -0.4446020952038907681, -0.02909913904661340714, -1.934055118110236338 ) ) ;
#25789=CARTESIAN_POINT ( 'NONE',  ( -0.5131133041954075713, -0.2529800193559338384, 0.9399606299212598381 ) ) ;
#25791=DIRECTION ( 'NONE',  ( -1.000000000000000000, 0.000000000000000000, 0.000000000000000000 ) ) ;
#25792=AXIS2_PLACEMENT_3D ( 'NONE', #23550, #8959, #11633 ) ;
#25793=CARTESIAN_POINT ( 'NONE',  ( -0.2272836761397795113, -0.2962590301041581053, -3.115157480314960647 ) ) ;
#25805=ORIENTED_EDGE ( 'NONE', *, *, #18832, .F. ) ;
#25809=CARTESIAN_POINT ( 'NONE',  ( -0.2268096725222457366, -0.4600326175560556230, 1.766732283464566899 ) ) ;
#25811=CARTESIAN_POINT ( 'NONE',  ( -0.4600326175560703335, -0.2268096725222389642, 1.747047244094488194 ) ) ;
#25817=CARTESIAN_POINT ( 'NONE',  ( 0.04679574315772527804, -0.3551931031211721379, -3.115157480314960647 ) ) ;
#25823=CARTESIAN_POINT ( 'NONE',  ( 0.3346456692913385988, 0.000000000000000000, 1.973425196850393970 ) ) ;
#25826=VECTOR ( 'NONE', #8201, 39.37007874015748143 ) ;
#25839=CARTESIAN_POINT ( 'NONE',  ( -0.3937007874015748254, 4.821444091131312140E-17, -3.115157480314960647 ) ) ;
#25844=CARTESIAN_POINT ( 'NONE',  ( 0.4921259842519685179, 2.987958743070287587E-17, -1.569881889763779625 ) ) ;
#25847=CARTESIAN_POINT ( 'NONE',  ( -0.01288382760289588647, 0.1968503937007873850, -3.174212598425197207 ) ) ;
#25850=( LENGTH_UNIT ( ) NAMED_UNIT ( * ) SI_UNIT ( $, .METRE. ) ) ;
#25857=CARTESIAN_POINT ( 'NONE',  ( -0.5511811023622047445, 0.000000000000000000, 0.9202755905511811330 ) ) ;
#25859=DIMENSIONAL_EXPONENTS ( 1.000000000000000000, 0.000000000000000000, 0.000000000000000000, 0.000000000000000000, 0.000000000000000000, 0.000000000000000000, 0.000000000000000000 ) ;
#25867=CARTESIAN_POINT ( 'NONE',  ( -0.3856568748491470133, -0.3381512095065993262, -1.550196850393700920 ) ) ;
#25871=CARTESIAN_POINT ( 'NONE',  ( -0.09842519685039370636, 0.2165354330708661457, -3.456364829396327831 ) ) ;
#25879=CARTESIAN_POINT ( 'NONE',  ( -0.1839420097223181394, -0.5417097841048805762, 0.9399606299212598381 ) ) ;
#25880=EDGE_CURVE ( 'NONE', #10004, #15380, #15584, .T. ) ;
#25881=DIRECTION ( 'NONE',  ( -0.000000000000000000, -1.000000000000000000, -0.000000000000000000 ) ) ;
#25882=ORIENTED_EDGE ( 'NONE', *, *, #11383, .T. ) ;
#25889=CARTESIAN_POINT ( 'NONE',  ( 0.1649135259639241124, 0.4856708409191630715, -1.550196850393700920 ) ) ;
#25890=CARTESIAN_POINT ( 'NONE',  ( 0.1838434515533423907, -0.5417490723641140704, 0.9399606299212598381 ) ) ;
#25895=EDGE_LOOP ( 'NONE', ( #1419, #19450, #1587, #12753 ) ) ;
#25908=CARTESIAN_POINT ( 'NONE',  ( -0.4921259842519395411, 0.03220957031763951872, -1.550196850393700920 ) ) ;
#25910=CARTESIAN_POINT ( 'NONE',  ( -0.1458850421962728516, -0.4296318976990441407, -1.934055118110236338 ) ) ;
#25924=CARTESIAN_POINT ( 'NONE',  ( -0.2991932138496531390, 0.3411003281196664516, -1.934055118110236338 ) ) ;
#25927=CARTESIAN_POINT ( 'NONE',  ( 0.5526079293737076181, -0.1480156394741905801, 0.9399606299212598381 ) ) ;
#25932=CARTESIAN_POINT ( 'NONE',  ( 0.3350125228553208490, -0.2937477835499151535, -1.934055118110235894 ) ) ;
#25943=ORIENTED_EDGE ( 'NONE', *, *, #7056, .F. ) ;
#25954=CARTESIAN_POINT ( 'NONE',  ( -0.3349073414798507953, 0.1651192144506273274, -3.115157480314960647 ) ) ;
#25960=CARTESIAN_POINT ( 'NONE',  ( 0.04380447413658805633, -0.3324885138898231451, 1.953740157480315043 ) ) ;
#25967=ORIENTED_EDGE ( 'NONE', *, *, #14363, .F. ) ;
#25975=ORIENTED_EDGE ( 'NONE', *, *, #26454, .F. ) ;
#25986=CARTESIAN_POINT ( 'NONE',  ( -0.07870736599817813872, 0.2165354330708661457, -3.212150913008700481 ) ) ;
#25987=VERTEX_POINT ( 'NONE', #5860 ) ;
#25990=LINE ( 'NONE', #6920, #17107 ) ;
#25995=EDGE_LOOP ( 'NONE', ( #25882, #25080 ) ) ;
#25996=CARTESIAN_POINT ( 'NONE',  ( -0.4152525734086685016, 0.3642352168757148623, 0.9399606299212598381 ) ) ;
#26004=CARTESIAN_POINT ( 'NONE',  ( 0.09842519685039351207, 0.1968503937007873850, -3.548228346456693050 ) ) ;
#26014=CARTESIAN_POINT ( 'NONE',  ( 0.5708661417322835607, 0.03736310157557569400, 0.9399606299212598381 ) ) ;
#26024=B_SPLINE_CURVE_WITH_KNOTS ( 'NONE', 2,
 ( #9993, #20871, #5485 ),
 .UNSPECIFIED., .F., .F.,
 ( 3, 3 ),
 ( 0.000000000000000000, 1.000000000000000000 ),
 .UNSPECIFIED. ) ;
#26041=CARTESIAN_POINT ( 'NONE',  ( -0.4423390553432706152, 0.2180862235769438773, -1.550196850393700920 ) ) ;
#26042=CARTESIAN_POINT ( 'NONE',  ( 0.1188866373884749916, -0.4438564651657395665, -1.928289503579163178 ) ) ;
#26043=DIRECTION ( 'NONE',  ( -0.000000000000000000, -0.000000000000000000, 1.000000000000000000 ) ) ;
#26045=CARTESIAN_POINT ( 'NONE',  ( 0.4777261797697372470, -0.2355331214654103889, 1.747047244094488194 ) ) ;
#26058=CARTESIAN_POINT ( 'NONE',  ( 0.3543307086614173596, -0.02319089060379044345, 1.953740157480315043 ) ) ;
#26067=CARTESIAN_POINT ( 'NONE',  ( -0.05811937031499277845, -0.4417502570510357662, -1.934055118110236338 ) ) ;
#26068=CARTESIAN_POINT ( 'NONE',  ( -0.09660931395005439848, 0.3606853515406323596, -3.115157480314960647 ) ) ;
#26074=CARTESIAN_POINT ( 'NONE',  ( -0.4446020952038907681, 0.000000000000000000, -1.934055118110236338 ) ) ;
#26080=CARTESIAN_POINT ( 'NONE',  ( -0.5118110236220472231, -0.03349795313264326835, 1.766732283464566899 ) ) ;
#26081=CARTESIAN_POINT ( 'NONE',  ( -0.4600326175560697783, 0.2268096725222554233, 1.747047244094488194 ) ) ;
#26086=CARTESIAN_POINT ( 'NONE',  ( 0.09660931395005455113, -0.3606853515406215904, -3.115157480314960647 ) ) ;
#26088=ORIENTED_EDGE ( 'NONE', *, *, #2298, .T. ) ;
#26094=CARTESIAN_POINT ( 'NONE',  ( -0.3239425792934414461, 0.08676778863010937981, 1.953740157480315043 ) ) ;
#26097=CARTESIAN_POINT ( 'NONE',  ( 0.4585215200179055817, -2.840735999735804609E-17, -1.928289503579156516 ) ) ;
#26101=ORIENTED_EDGE ( 'NONE', *, *, #19019, .T. ) ;
#26120=CARTESIAN_POINT ( 'NONE',  ( -0.04956879678463866484, 0.1968503937007873850, -3.186635197791150453 ) ) ;
#26126=DIRECTION ( 'NONE',  ( 1.000000000000000000, 0.000000000000000000, 0.000000000000000000 ) ) ;
#26132=CARTESIAN_POINT ( 'NONE',  ( 0.5230301363771271417, 0.1775991818008589573, 0.9399606299212598381 ) ) ;
#26134=EDGE_CURVE ( 'NONE', #8508, #17093, #22225, .T. ) ;
#26149=CARTESIAN_POINT ( 'NONE',  ( 0.5671862884095085766, -0.07472527936312026164, 0.9399606299212598381 ) ) ;
#26177=CARTESIAN_POINT ( 'NONE',  ( -0.3252100150720236282, -0.3707612262533184766, -1.569881889763779625 ) ) ;
#26178=CARTESIAN_POINT ( 'NONE',  ( 0.3645739570812633890, 0.2796934465393874358, -1.928289503579156072 ) ) ;
#26180=CARTESIAN_POINT ( 'NONE',  ( 0.2297883689023240139, -0.3979194638820313656, -1.928289503579174280 ) ) ;
#26194=CARTESIAN_POINT ( 'NONE',  ( -0.4527559054764770385, 0.000000000000000000, -1.934055118110236338 ) ) ;
#26200=CARTESIAN_POINT ( 'NONE',  ( 0.1651192144506298254, 0.3349073414798210413, -3.115157480314960647 ) ) ;
#26207=CARTESIAN_POINT ( 'NONE',  ( -0.1288129352161812846, -0.4793172621399191535, -1.569881889763779848 ) ) ;
#26211=EDGE_CURVE ( 'NONE', #7455, #21621, #15494, .T. ) ;
#26220=CARTESIAN_POINT ( 'NONE',  ( 0.1651192144506304360, -0.3349073414798397486, -3.115157480314960647 ) ) ;
#26226=CARTESIAN_POINT ( 'NONE',  ( 0.1078280746903870629, -0.3175540113612215221, 1.953740157480315043 ) ) ;
#26251=CARTESIAN_POINT ( 'NONE',  ( 0.000000000000000000, 0.000000000000000000, 1.953740157480315043 ) ) ;
#26252=CARTESIAN_POINT ( 'NONE',  ( 0.4954415918530860607, 0.1327036767659604266, 1.766732283464566899 ) ) ;
#26263=CARTESIAN_POINT ( 'NONE',  ( 0.3362148458988418187, -0.4382482975805321312, 0.9202755905511811330 ) ) ;
#26279=CARTESIAN_POINT ( 'NONE',  ( -0.07472527936312729768, -0.5671862884094908130, 0.9399606299212598381 ) ) ;
#26280=CARTESIAN_POINT ( 'NONE',  ( -0.4092783051644229841, -0.3145317858139328182, 1.766732283464566899 ) ) ;
#26306=CARTESIAN_POINT ( 'NONE',  ( 0.1327036767636011194, 0.4954415918535620689, -1.550196850393700920 ) ) ;
#26311=CARTESIAN_POINT ( 'NONE',  ( -0.2442565704126104242, 0.4954197419817720216, 0.9202755905511811330 ) ) ;
#26327=ORIENTED_EDGE ( 'NONE', *, *, #11440, .T. ) ;
#26335=CARTESIAN_POINT ( 'NONE',  ( 0.1970988029421506804, -0.3995913070740104711, -1.934055118110236560 ) ) ;
#26336=CARTESIAN_POINT ( 'NONE',  ( -0.3726024258163779246, -0.02438677169354843896, -3.115157480314960647 ) ) ;
#26348=CARTESIAN_POINT ( 'NONE',  ( -0.4092783051644230397, 0.3145317858139328182, 1.766732283464566899 ) ) ;
#26350=CARTESIAN_POINT ( 'NONE',  ( -0.5118110236220472231, 0.03349795313264340019, 1.747047244094488194 ) ) ;
#26352=CARTESIAN_POINT ( 'NONE',  ( -0.1200583359873055728, 0.3535721684717720859, -3.115157480314960647 ) ) ;
#26357=CARTESIAN_POINT ( 'NONE',  ( 0.3239425792934479409, 0.08676778863010962961, 1.953740157480315043 ) ) ;
#26364=CARTESIAN_POINT ( 'NONE',  ( -0.06690352886863247528, -0.5085315017396038195, -1.550196850393700476 ) ) ;
#26372=DIRECTION ( 'NONE',  ( -1.000000000000000000, 0.000000000000000000, 0.000000000000000000 ) ) ;
#26373=VERTEX_POINT ( 'NONE', #16311 ) ;
#26375=CARTESIAN_POINT ( 'NONE',  ( 0.1775730735577439323, 0.3074993854542599769, 1.953740157480315043 ) ) ;
#26395=CARTESIAN_POINT ( 'NONE',  ( -0.1429116519061075785, -0.5335524835332366989, 0.9202755905511811330 ) ) ;
#26408=CARTESIAN_POINT ( 'NONE',  ( 0.2041304421298504035, -0.2660793235464293249, 1.953740157480315043 ) ) ;
#26411=CARTESIAN_POINT ( 'NONE',  ( 0.5417097841048850171, 0.1839420097223152528, 0.9399606299212598381 ) ) ;
#26413=DIRECTION ( 'NONE',  ( 1.000000000000000000, 0.000000000000000000, -0.000000000000000000 ) ) ;
#26414=CARTESIAN_POINT ( 'NONE',  ( 0.3552064049866301976, 0.04673614183173152581, -3.115157480314960647 ) ) ;
#26434=FACE_OUTER_BOUND ( 'NONE', #3271, .T. ) ;
#26435=CARTESIAN_POINT ( 'NONE',  ( -0.06441834428466408635, -0.4889536969035170877, -1.550196850393700920 ) ) ;
#26436=CARTESIAN_POINT ( 'NONE',  ( 0.2031943647053979507, -0.4121342552748326060, -1.928289503579156960 ) ) ;
#26438=CARTESIAN_POINT ( 'NONE',  ( -0.07214854559198219386, 0.5476281405333177643, 0.9202755905511811330 ) ) ;
#26439=CARTESIAN_POINT ( 'NONE',  ( 0.000000000000000000, 0.000000000000000000, 0.9399606299212598381 ) ) ;
#26447=FILL_AREA_STYLE_COLOUR ( '', #2333 ) ;
#26454=EDGE_CURVE ( 'NONE', #19648, #5266, #13770, .T. ) ;
#26456=CARTESIAN_POINT ( 'NONE',  ( 0.1141145734057279204, 0.3362554559025014989, 1.953740157480315487 ) ) ;
#26458=CARTESIAN_POINT ( 'NONE',  ( 0.4296318976989615401, 0.1458850421962473720, -1.934055118110236338 ) ) ;
#26467=CARTESIAN_POINT ( 'NONE',  ( 0.2488091035916884242, -0.2836590635674675620, -3.100567304031759175 ) ) ;
#26480=CARTESIAN_POINT ( 'NONE',  ( 0.5118110236220472231, 0.000000000000000000, 1.747047244094488194 ) ) ;
#26482=CARTESIAN_POINT ( 'NONE',  ( -0.04877294052295848975, -0.3702005978258383068, -3.115157480314960647 ) ) ;
#26487=CARTESIAN_POINT ( 'NONE',  ( 0.2904160862623688666, 0.1677079028045472542, 1.953740157480315043 ) ) ;
#26493=EDGE_LOOP ( 'NONE', ( #16127, #24863, #25225, #17438 ) ) ;
#26495=CARTESIAN_POINT ( 'NONE',  ( 0.02063739440522441987, 0.1968503937007874127, -3.624910829905205745 ) ) ;
#26497=CARTESIAN_POINT ( 'NONE',  ( -0.4921259842519685179, 0.000000000000000000, -1.550196850393700920 ) ) ;
#26504=CARTESIAN_POINT ( 'NONE',  ( 0.04638120790932896698, -0.3520466617656974884, 1.953740157480315043 ) ) ;
#26516=CARTESIAN_POINT ( 'NONE',  ( -2.685748425196850164E-17, 0.000000000000000000, -1.934055118110236338 ) ) ;
#26521=CARTESIAN_POINT ( 'NONE',  ( -0.3346456692913385988, 4.268512490100411279E-17, 1.953740157480315043 ) ) ;
#26525=CARTESIAN_POINT ( 'NONE',  ( 0.4300830224589218820, 0.3772436174784425389, 0.9399606299212598381 ) ) ;
#26538=CARTESIAN_POINT ( 'NONE',  ( -0.3239425792934414461, 0.08676778863010937981, 1.953740157480315043 ) ) ;
#26543=CARTESIAN_POINT ( 'NONE',  ( -2.685748425196850164E-17, 0.000000000000000000, -3.036417322828325105 ) ) ;
#26559=CARTESIAN_POINT ( 'NONE',  ( -0.5085329218535696860, 0.06689639104893733978, -1.550196850393700920 ) ) ;
#26568=CARTESIAN_POINT ( 'NONE',  ( 0.3175540113612325133, 0.1078280746903942239, 1.973425196850393970 ) ) ;
#26569=CARTESIAN_POINT ( 'NONE',  ( -0.1649135259639237794, 0.4856708409191340947, -1.550196850393700920 ) ) ;
#26571=CARTESIAN_POINT ( 'NONE',  ( 0.2796934465393868807, 0.3645739570812638330, -1.928289503579156072 ) ) ;
#26574=CARTESIAN_POINT ( 'NONE',  ( 0.4783323773986568606, 0.2762247810518930202, 0.9202755905511811330 ) ) ;
#26599=CARTESIAN_POINT ( 'NONE',  ( 0.02963280468032034737, -0.4527559054764770385, -1.934055118110236338 ) ) ;
#26608=CARTESIAN_POINT ( 'NONE',  ( -0.3726024258163779246, 0.000000000000000000, -3.115157480314960647 ) ) ;
#26612=CARTESIAN_POINT ( 'NONE',  ( -0.2938049579018706114, 0.3349573549949406148, -1.934055118110236338 ) ) ;
#26619=CARTESIAN_POINT ( 'NONE',  ( -0.06699507805368211388, 0.5085118447801414421, 1.747047244094488194 ) ) ;
#26625=CARTESIAN_POINT ( 'NONE',  ( -0.3765118517642104257, 0.02464264302297881210, -3.100567304031763172 ) ) ;
#26626=EDGE_LOOP ( 'NONE', ( #11122, #3208, #21739, #21016 ) ) ;
#26629=CARTESIAN_POINT ( 'NONE',  ( 0.3346456692913385988, -0.02190250779246876237, 1.953740157480315043 ) ) ;
#26642=CARTESIAN_POINT ( 'NONE',  ( -0.07667729696029146336, 0.1968503937007874405, -3.252002554478575558 ) ) ;
#26646=CARTESIAN_POINT ( 'NONE',  ( 0.02576258704323619239, 0.2165354330708661734, -3.176774342847608068 ) ) ;
#26648=CARTESIAN_POINT ( 'NONE',  ( 0.1570220809524471017, 0.3184841198566427112, 1.953740157480315043 ) ) ;
#26654=CARTESIAN_POINT ( 'NONE',  ( 0.5043504886477625515, 0.1712563538832952981, 1.747047244094488194 ) ) ;
#26655=CARTESIAN_POINT ( 'NONE',  ( 0.5085118447801419972, 0.06699507805369840641, 1.766732283464566899 ) ) ;
#26663=CARTESIAN_POINT ( 'NONE',  ( -0.1141145734061086853, -0.3362554559022283285, 1.953740157480315043 ) ) ;
#26665=CARTESIAN_POINT ( 'NONE',  ( -2.685748425196850164E-17, 0.000000000000000000, -1.934055118110236338 ) ) ;
#26668=CARTESIAN_POINT ( 'NONE',  ( 0.06441834428466665374, -0.4889536969035324088, -1.569881889763779625 ) ) ;
#26671=CARTESIAN_POINT ( 'NONE',  ( -0.1429116519060979196, -0.5335524835332288163, 0.9399606299212598381 ) ) ;
#26679=CIRCLE ( 'NONE', #6858, 0.3346456692913385988 ) ;
#26692=ORIENTED_EDGE ( 'NONE', *, *, #3729, .F. ) ;
#26699=CARTESIAN_POINT ( 'NONE',  ( 0.06048688226684505176, 0.1968503937008365401, -3.626935712454951943 ) ) ;
#26704=AXIS2_PLACEMENT_3D ( 'NONE', #11433, #10250, #20190 ) ;
#26707=CARTESIAN_POINT ( 'NONE',  ( 0.2313841235333772006, 0.3010840436257775088, -3.100567304031763172 ) ) ;
#26712=CARTESIAN_POINT ( 'NONE',  ( -0.3239425792934402248, -0.08676778863011362641, 1.973425196850393970 ) ) ;
#26715=CARTESIAN_POINT ( 'NONE',  ( -0.3707612262533164782, -0.3252100150720257377, -1.550196850393700920 ) ) ;
#26718=CARTESIAN_POINT ( 'NONE',  ( 0.4954197419817712444, -0.2442565704126122561, 0.9202755905511811330 ) ) ;
#26738=CARTESIAN_POINT ( 'NONE',  ( -0.02963280468032184270, -0.4527559054764770385, -1.934055118110236338 ) ) ;
#26743=DIRECTION ( 'NONE',  ( -0.000000000000000000, -1.000000000000000000, -0.000000000000000000 ) ) ;
#26751=CARTESIAN_POINT ( 'NONE',  ( -0.04928467685643870416, 0.3740848232703742893, -3.100567304031763172 ) ) ;
#26753=EDGE_CURVE ( 'NONE', #18631, #21933, #2086, .T. ) ;
#26759=CARTESIAN_POINT ( 'NONE',  ( -0.4417361510194242613, -0.05819755867303597063, -1.934055118110236338 ) ) ;
#26765=CARTESIAN_POINT ( 'NONE',  ( -0.2268096725222397969, 0.4600326175560398023, 1.747047244094488194 ) ) ;
#26769=CARTESIAN_POINT ( 'NONE',  ( -0.02464264302293858039, -0.3765118517642103702, -3.100567304031763172 ) ) ;
#26771=ORIENTED_EDGE ( 'NONE', *, *, #8518, .T. ) ;
#26774=CARTESIAN_POINT ( 'NONE',  ( 0.3175540113612412840, -0.1078280746903980958, 1.953740157480315043 ) ) ;
#26784=CARTESIAN_POINT ( 'NONE',  ( -0.07668265949366928624, 0.1968503937007874127, -3.568865316179323788 ) ) ;
#26787=CARTESIAN_POINT ( 'NONE',  ( 0.07874015748031491790, 0.1968503937007874127, -3.262315100355583031 ) ) ;
#26789=CARTESIAN_POINT ( 'NONE',  ( -0.04380501567505456356, 0.3346456692913385988, 1.973425196850394192 ) ) ;
#26795=CARTESIAN_POINT ( 'NONE',  ( -0.02319089060378155473, 0.3543307086614173596, 1.953740157480315043 ) ) ;
#26802=CARTESIAN_POINT ( 'NONE',  ( -0.3242071728275051634, -0.4225965726693019509, 1.747047244094488194 ) ) ;
#26803=CARTESIAN_POINT ( 'NONE',  ( -0.2564944395515745823, 0.4441657790107744752, 1.766732283464566899 ) ) ;
#26813=EDGE_LOOP ( 'NONE', ( #20006, #20781, #2497, #6162 ) ) ;
#26815=CARTESIAN_POINT ( 'NONE',  ( -0.03220957031754079214, -0.4921259842519684624, -1.569881889763779625 ) ) ;
#26818=CARTESIAN_POINT ( 'NONE',  ( 0.4783323773986630778, -0.2762247810518744240, 0.9399606299212598381 ) ) ;
#26837=DIRECTION ( 'NONE',  ( -0.000000000000000000, -1.000000000000000000, -0.000000000000000000 ) ) ;
#26839=DIRECTION ( 'NONE',  ( 1.000000000000000000, 0.000000000000000000, 0.000000000000000000 ) ) ;
#26846=CARTESIAN_POINT ( 'NONE',  ( 0.09842519685039351207, 0.1968503937007873850, -3.548228346456693050 ) ) ;
#26855=CARTESIAN_POINT ( 'NONE',  ( -0.04928528614549706338, 0.3765118517642103146, -3.100567304031762728 ) ) ;
#26861=CARTESIAN_POINT ( 'NONE',  ( 0.2211428102655756955, 0.2521176338356569957, 1.973425196850393970 ) ) ;
#26862=CARTESIAN_POINT ( 'NONE',  ( -0.4889536969034878333, -0.06441834428466509943, -1.550196850393700920 ) ) ;
#26864=CARTESIAN_POINT ( 'NONE',  ( -0.07214943758244271588, 0.5511811023622048555, 0.9202755905511812440 ) ) ;
#26865=CARTESIAN_POINT ( 'NONE',  ( -0.2762247810519398716, 0.4783323773986303262, 0.9399606299212598381 ) ) ;
#26871=CARTESIAN_POINT ( 'NONE',  ( 0.1275996891957681401, 0.4763861460130344172, -1.569881889763779625 ) ) ;
#26872=CARTESIAN_POINT ( 'NONE',  ( 0.3010840436257777308, -0.2313841235333769231, -3.100567304031763616 ) ) ;
#26886=CARTESIAN_POINT ( 'NONE',  ( 0.3599896729929412120, -0.2761764805255614297, -1.934055118110236338 ) ) ;
#26891=CARTESIAN_POINT ( 'NONE',  ( 0.5118110236220473341, 6.402768735150616610E-17, -1.550196850393700920 ) ) ;
#26896=CARTESIAN_POINT ( 'NONE',  ( -0.3572819248074403653, -0.1213180142433946673, -3.100567304031765392 ) ) ;
#26902=CARTESIAN_POINT ( 'NONE',  ( -0.3349573549949665940, -0.2938049579018697788, -1.934055118110236338 ) ) ;
#26905=CARTESIAN_POINT ( 'NONE',  ( -0.4121342552748409327, 0.2031943647053852109, -1.928289503579154074 ) ) ;
#26911=CARTESIAN_POINT ( 'NONE',  ( 0.09842519685039370636, 0.2165354330708661457, -3.456364829396327387 ) ) ;
#26913=CARTESIAN_POINT ( 'NONE',  ( 0.3382184156732163660, 0.3855916753051394363, 1.747047244094488194 ) ) ;
#26919=CARTESIAN_POINT ( 'NONE',  ( 0.09762295995069844579, 0.3644697409450269321, -3.100567304031763172 ) ) ;
#26926=ORIENTED_EDGE ( 'NONE', *, *, #5794, .T. ) ;
#26927=CARTESIAN_POINT ( 'NONE',  ( 0.1648275707509661014, 0.4857079805365772107, -1.550196850393701142 ) ) ;
#26929=PLANE ( 'NONE',  #6733 ) ;
#26932=CARTESIAN_POINT ( 'NONE',  ( -0.1152775731717075036, 0.4303822302054133853, -1.934055118110236338 ) ) ;
#26935=CARTESIAN_POINT ( 'NONE',  ( -0.4446020952038907681, 0.000000000000000000, -1.934055118110236338 ) ) ;
#26940=CARTESIAN_POINT ( 'NONE',  ( -0.08759279594700326854, 0.3259357382551448246, 1.973425196850393526 ) ) ;
#26944=CARTESIAN_POINT ( 'NONE',  ( 0.2056553984168021654, -0.2676050456844303316, 1.973425196850393970 ) ) ;
#26945=CARTESIAN_POINT ( 'NONE',  ( 0.09187177619659094019, 0.3429980251342388264, 1.953740157480315043 ) ) ;
#26954=CARTESIAN_POINT ( 'NONE',  ( -0.3512268162760395773, 0.4004221243553298115, 1.747047244094488194 ) ) ;
#26956=CARTESIAN_POINT ( 'NONE',  ( 0.5118110236220472231, 0.000000000000000000, 1.766732283464566899 ) ) ;
#26968=CARTESIAN_POINT ( 'NONE',  ( -0.3252100150720236282, -0.3707612262533184766, -1.569881889763779625 ) ) ;
#26978=CARTESIAN_POINT ( 'NONE',  ( -0.2041304421298407168, -0.2660793235464189999, 1.953740157480315043 ) ) ;
#26999=CARTESIAN_POINT ( 'NONE',  ( -0.09586345222255253373, 0.1968503937007873850, -3.573990933995847996 ) ) ;
#27001=CARTESIAN_POINT ( 'NONE',  ( -0.3856588814717645808, 0.3381532161291478378, -1.550196850393700476 ) ) ;
#27014=CARTESIAN_POINT ( 'NONE',  ( -0.3346456692913385988, 0.02190250779246044610, 1.973425196850393970 ) ) ;
#27015=CARTESIAN_POINT ( 'NONE',  ( -0.3382184156749069581, -0.3855916753034488997, -1.550196850393700920 ) ) ;
#27016=CARTESIAN_POINT ( 'NONE',  ( 0.4816145447621894560, 0.2775852647713619170, 0.9202755905511812440 ) ) ;
#27017=CARTESIAN_POINT ( 'NONE',  ( 0.03001016326913514068, -0.4585215200179055817, -1.928289503579156516 ) ) ;
#27019=CARTESIAN_POINT ( 'NONE',  ( 0.03607471876262385857, -0.5511811023622048555, 0.9202755905511811330 ) ) ;
#27024=ADVANCED_FACE ( 'NONE', ( #13537 ), #314, .F. ) ;
#27029=CARTESIAN_POINT ( 'NONE',  ( 0.03488411621188176881, 0.5314974819112028293, 1.747047244094488194 ) ) ;
#27030=SURFACE_STYLE_FILL_AREA ( #3268 ) ;
#27035=DIRECTION ( 'NONE',  ( -0.2588190448135643806, 3.169619147893069890E-17, 0.9659258263664939337 ) ) ;
#27039=ORIENTED_EDGE ( 'NONE', *, *, #16585, .T. ) ;
#27051=CARTESIAN_POINT ( 'NONE',  ( 0.2181198385717777743, -0.2842139414039452361, -3.115157480314960647 ) ) ;
#27053=CARTESIAN_POINT ( 'NONE',  ( 0.4218945342797225662, -0.1432577568504558585, -1.934055118110236338 ) ) ;
#27054=CARTESIAN_POINT ( 'NONE',  ( 0.3979194638820595098, 0.2297883689023132170, -1.928289503579157183 ) ) ;
#27058=CARTESIAN_POINT ( 'NONE',  ( 0.09842519685039370636, 0.2165354330708661457, -3.364501312335955063 ) ) ;
#27060=CARTESIAN_POINT ( 'NONE',  ( 0.4225965726692672009, 0.3242071728275124354, 1.747047244094488194 ) ) ;
#27066=CARTESIAN_POINT ( 'NONE',  ( 0.1213180142433946118, -0.3572819248074403653, -3.100567304031765392 ) ) ;
#27070=CARTESIAN_POINT ( 'NONE',  ( 0.3324885138898230341, -0.04380447413659129680, 1.953740157480315043 ) ) ;
#27074=ORIENTED_EDGE ( 'NONE', *, *, #12850, .T. ) ;
#27076=CARTESIAN_POINT ( 'NONE',  ( 0.3996230174612964148, -0.1970259548082136380, -1.934055118110236338 ) ) ;
#27082=CARTESIAN_POINT ( 'NONE',  ( 0.2362439534887500470, 0.2693339498142248156, -3.115157480314960647 ) ) ;
#27085=FACE_OUTER_BOUND ( 'NONE', #19603, .T. ) ;
#27090=CARTESIAN_POINT ( 'NONE',  ( 0.3184841198566246701, -0.1570220809524502659, 1.953740157480315043 ) ) ;
#27098=CARTESIAN_POINT ( 'NONE',  ( 0.4954415918530775120, -0.1327036767659478256, 1.747047244094488194 ) ) ;
#27099=DIMENSIONAL_EXPONENTS ( 1.000000000000000000, 0.000000000000000000, 0.000000000000000000, 0.000000000000000000, 0.000000000000000000, 0.000000000000000000, 0.000000000000000000 ) ;
#27101=CARTESIAN_POINT ( 'NONE',  ( 0.1649135259617042493, -0.4856708409200646281, 1.766732283464566899 ) ) ;
#27103=FACE_OUTER_BOUND ( 'NONE', #1117, .T. ) ;
#27111=EDGE_CURVE ( 'NONE', #16690, #5287, #2603, .T. ) ;
#27113=CARTESIAN_POINT ( 'NONE',  ( -0.2180862235769353841, 0.4423390553432505756, -1.569881889763779625 ) ) ;
#27143=CARTESIAN_POINT ( 'NONE',  ( 0.04838950581350980051, 0.1968503937007873850, -3.611194239255285598 ) ) ;
#27153=STYLED_ITEM ( 'NONE', ( #20525 ), #12711 ) ;
#27158=CARTESIAN_POINT ( 'NONE',  ( 0.3324885138898233672, 0.04380447413659172701, 1.973425196850393970 ) ) ;
#27159=CARTESIAN_POINT ( 'NONE',  ( 0.4954415918535722829, 0.1327036767636095571, -1.550196850393700920 ) ) ;
#27162=CARTESIAN_POINT ( 'NONE',  ( -0.1775991818008590406, -0.5230301363771331369, 0.9202755905511811330 ) ) ;
#27164=EDGE_LOOP ( 'NONE', ( #2478, #8123 ) ) ;
#27171=CARTESIAN_POINT ( 'NONE',  ( 0.3242892624569754800, 0.4225434286518392479, 1.747047244094487972 ) ) ;
#27194=CARTESIAN_POINT ( 'NONE',  ( -0.1151343661285636755, -0.3392608232660268563, -3.115157480314960647 ) ) ;
#27196=CARTESIAN_POINT ( 'NONE',  ( -0.02909913904662089768, -0.4446020952038907681, -1.934055118110236338 ) ) ;
#27200=CARTESIAN_POINT ( 'NONE',  ( -0.3512268162760395773, 0.4004221243553298115, 1.747047244094488194 ) ) ;
#27205=ORIENTED_EDGE ( 'NONE', *, *, #22244, .T. ) ;
#27206=CARTESIAN_POINT ( 'NONE',  ( -0.2488091035917009419, 0.2836590635674538508, -3.100567304031763172 ) ) ;
#27218=CARTESIAN_POINT ( 'NONE',  ( 0.02339816079119036787, -0.3574975638436101444, -3.115157480314960647 ) ) ;
#27220=CARTESIAN_POINT ( 'NONE',  ( -0.3346456692913387099, 0.04380501567505452193, 1.973425196850393970 ) ) ;
#27229=CARTESIAN_POINT ( 'NONE',  ( 0.5672055940108537975, 0.07462095020313340432, 0.9399606299212600602 ) ) ;
#27235=CARTESIAN_POINT ( 'NONE',  ( 0.03478633594543814600, -0.5314960629921260393, 1.747047244094488194 ) ) ;
#27236=CARTESIAN_POINT ( 'NONE',  ( -0.06699507805368211388, 0.5085118447801414421, 1.747047244094488194 ) ) ;
#27244=CARTESIAN_POINT ( 'NONE',  ( -0.3349573549949658169, 0.2938049579018958690, -1.934055118110236338 ) ) ;
#27251=CARTESIAN_POINT ( 'NONE',  ( -0.06441834428466812479, 0.4889536969035060410, -1.550196850393700920 ) ) ;
#27272=CARTESIAN_POINT ( 'NONE',  ( -0.2564944395535628252, -0.4441657790094413749, -1.550196850393700920 ) ) ;
#27292=CARTESIAN_POINT ( 'NONE',  ( 0.3239425792934479409, 0.08676778863010962961, 1.953740157480315043 ) ) ;
#27295=CARTESIAN_POINT ( 'NONE',  ( 0.4152525734086595088, -0.3642352168757885811, 0.9399606299212598381 ) ) ;
#27312=DIRECTION ( 'NONE',  ( -0.000000000000000000, -0.000000000000000000, -1.000000000000000000 ) ) ;
#27318=CARTESIAN_POINT ( 'NONE',  ( -0.09842519685039373412, 0.2991866959364303802, -3.272637795275590733 ) ) ;
#27330=CARTESIAN_POINT ( 'NONE',  ( 0.1432577568504648236, 0.4218945342797248421, -1.934055118110236338 ) ) ;
#27336=VERTEX_POINT ( 'NONE', #4854 ) ;
#27339=CARTESIAN_POINT ( 'NONE',  ( 0.2663596103035608120, 0.4612490782035171266, 1.747047244094488194 ) ) ;
#27344=CARTESIAN_POINT ( 'NONE',  ( -0.3740848232703753440, -0.04928467685643751067, -3.100567304031760507 ) ) ;
#27345=FACE_OUTER_BOUND ( 'NONE', #24978, .T. ) ;
#27348=B_SPLINE_CURVE_WITH_KNOTS ( 'NONE', 3,
 ( #3040, #9542, #5468, #18145, #9837, #16347, #20718, #1364, #9976, #26789, #26940, #16066, #11818, #16479, #18576, #22557, #27220, #1099 ),
 .UNSPECIFIED., .F., .F.,
 ( 4, 2, 2, 2, 2, 2, 2, 2, 4 ),
 ( 0.000000000000000000, 0.06249999999999997224, 0.1249999999999999722, 0.1874999999999999722, 0.2499999999999999445, 0.3124999999999999445, 0.3750000000000000000, 0.4375000000000000000, 0.5000000000000000000 ),
 .UNSPECIFIED. ) ;
#27349=CARTESIAN_POINT ( 'NONE',  ( 0.3543307086614173596, 0.02319089060379041917, 1.953740157480315043 ) ) ;
#27353=CARTESIAN_POINT ( 'NONE',  ( -0.3667122560601320802, -0.09855118063547678442, -3.100567304031763172 ) ) ;
#27354=CARTESIAN_POINT ( 'NONE',  ( 0.1839420097223146422, 0.5417097841049177687, 0.9399606299212598381 ) ) ;
#27356=DIRECTION ( 'NONE',  ( 0.000000000000000000, 0.000000000000000000, -1.000000000000000000 ) ) ;
#27361=CARTESIAN_POINT ( 'NONE',  ( -0.3574975638436101444, -0.02339816079122979120, -3.115157480314960647 ) ) ;
#27365=CARTESIAN_POINT ( 'NONE',  ( 0.000000000000000000, 0.000000000000000000, 2.504921259842519898 ) ) ;
#27377=CARTESIAN_POINT ( 'NONE',  ( 6.136516277395897527E-17, 0.2165354330708661457, -3.646653543307086576 ) ) ;
#27379=CARTESIAN_POINT ( 'NONE',  ( -0.5085118447801421082, 0.06699507805369804558, 1.766732283464566899 ) ) ;
#27383=CARTESIAN_POINT ( 'NONE',  ( -0.3551931031211768008, 0.04679574315772456333, -3.115157480314960647 ) ) ;
#27388=CARTESIAN_POINT ( 'NONE',  ( 0.3346456692913385988, 0.000000000000000000, 1.953740157480315043 ) ) ;
#27391=CARTESIAN_POINT ( 'NONE',  ( 0.4889536969034951053, 0.06441834428467130280, -1.550196850393700920 ) ) ;
#27398=CARTESIAN_POINT ( 'NONE',  ( -0.3765118517642104257, 2.305470170520414967E-17, -3.100567304031763172 ) ) ;
#27428=CARTESIAN_POINT ( 'NONE',  ( -0.09586345222256538456, 0.2165354330708661457, -3.573990933995853769 ) ) ;
#27432=CARTESIAN_POINT ( 'NONE',  ( 0.3324885138898166503, 0.04380447413659039474, 1.953740157480315043 ) ) ;
#27433=CARTESIAN_POINT ( 'NONE',  ( 0.1649135259639267770, -0.4856708409191258236, -1.550196850393700920 ) ) ;
#27436=CARTESIAN_POINT ( 'NONE',  ( -0.2762247810519084523, -0.4783323773986298266, 0.9399606299212598381 ) ) ;
#27443=CARTESIAN_POINT ( 'NONE',  ( 0.4921259842519685179, -0.03220957031753991784, -1.569881889763779625 ) ) ;
#27468=CARTESIAN_POINT ( 'NONE',  ( -0.1584824234590963832, -0.3213085410494903593, -3.115157480314960647 ) ) ;
#27473=CARTESIAN_POINT ( 'NONE',  ( -0.02963280468032184270, -0.4527559054764770385, -1.934055118110236338 ) ) ;
#27477=CARTESIAN_POINT ( 'NONE',  ( -0.4527559054764770385, 0.000000000000000000, -1.934055118110236338 ) ) ;
#27481=CARTESIAN_POINT ( 'NONE',  ( -0.4777261797697566759, 0.2355331214654138305, 1.747047244094488194 ) ) ;
#27486=CARTESIAN_POINT ( 'NONE',  ( -0.1570784101597038906, -0.3184623230427779395, 1.953740157480314821 ) ) ;
#27490=CARTESIAN_POINT ( 'NONE',  ( -0.3543307086614173596, -0.02319089060378156514, 1.953740157480315043 ) ) ;
#27499=CARTESIAN_POINT ( 'NONE',  ( -0.4954197419817796266, -0.2442565704126152260, 0.9399606299212598381 ) ) ;
#27507=CARTESIAN_POINT ( 'NONE',  ( -0.2842490391651705806, 0.2180698645301660521, -3.115157480314960647 ) ) ;
#27517=CARTESIAN_POINT ( 'NONE',  ( 0.5708675606921426171, 0.03746919241596965988, 0.9399606299212597271 ) ) ;
#27523=CARTESIAN_POINT ( 'NONE',  ( -0.1378076643338853602, -0.5144970376935932288, 1.747047244094488194 ) ) ;
#27525=CARTESIAN_POINT ( 'NONE',  ( -0.03349795313264251895, -0.5118110236220473341, 1.766732283464566899 ) ) ;
#27528=EDGE_LOOP ( 'NONE', ( #25466, #17660, #22534, #12046 ) ) ;
#27529=CARTESIAN_POINT ( 'NONE',  ( -0.2309201403895324856, -0.4006498629591504490, -1.928289503579156516 ) ) ;
#27531=CARTESIAN_POINT ( 'NONE',  ( 0.3007905576423847704, 0.1482986320106501610, 1.973425196850393970 ) ) ;
#27558=FACE_OUTER_BOUND ( 'NONE', #13975, .T. ) ;
#27567=CARTESIAN_POINT ( 'NONE',  ( -0.4954197419817560344, 0.2442565704126489212, 0.9202755905511811330 ) ) ;
#27582=CARTESIAN_POINT ( 'NONE',  ( 0.04380447413659065842, -0.3324885138898235892, 1.973425196850393970 ) ) ;
#27586=CARTESIAN_POINT ( 'NONE',  ( 0.1775991818008549328, -0.5230301363771188150, 0.9399606299212598381 ) ) ;
#27590=CARTESIAN_POINT ( 'NONE',  ( 0.2662775206740974898, 0.4613022222209450796, 1.747047244094488194 ) ) ;
#27594=CARTESIAN_POINT ( 'NONE',  ( -0.4889536969034878333, -0.06441834428466509943, -1.550196850393700920 ) ) ;
#27599=CARTESIAN_POINT ( 'NONE',  ( 0.5314960629921260393, 0.000000000000000000, 1.747047244094488194 ) ) ;
#27603=AXIS2_PLACEMENT_3D ( 'NONE', #9433, #9290, #18033 ) ;
#27604=DIRECTION ( 'NONE',  ( -1.000000000000000000, 0.000000000000000000, 0.000000000000000000 ) ) ;
#27614=CARTESIAN_POINT ( 'NONE',  ( -0.4438564651657478377, 0.1188866373884873845, -1.928289503579152742 ) ) ;
#27633=CARTESIAN_POINT ( 'NONE',  ( -0.3184841198566451537, -0.1570220809524492667, 1.953740157480315043 ) ) ;
#27639=CARTESIAN_POINT ( 'NONE',  ( 0.1480156394741928561, -0.5526079293736928522, 0.9399606299212598381 ) ) ;
#27647=CARTESIAN_POINT ( 'NONE',  ( -0.2180698645301862859, 0.2842490391651604775, -3.115157480314960647 ) ) ;
#27655=CARTESIAN_POINT ( 'NONE',  ( -0.5417516942597173646, 0.1838445375788849978, 0.9399606299212601712 ) ) ;
#27665=CARTESIAN_POINT ( 'NONE',  ( 0.2180698645301765992, 0.2842490391651533721, -3.115157480314960647 ) ) ;
#27666=CARTESIAN_POINT ( 'NONE',  ( 0.000000000000000000, 0.000000000000000000, 1.953740157480315043 ) ) ;
#27669=CARTESIAN_POINT ( 'NONE',  ( 0.2521176338356617697, -0.2211428102655709493, 1.973425196850393970 ) ) ;
#27676=AXIS2_PLACEMENT_3D ( 'NONE', #27718, #8219, #16839 ) ;
#27689=CARTESIAN_POINT ( 'NONE',  ( 0.3024344094364739277, 0.3935368318888683437, -1.569881889763779625 ) ) ;
#27692=CARTESIAN_POINT ( 'NONE',  ( 0.08600259748439817442, 0.1968503937007873850, -3.223068998490986825 ) ) ;
#27693=CARTESIAN_POINT ( 'NONE',  ( -0.09842519685039370636, 0.5905905511811023745, -3.272637795275590733 ) ) ;
#27700=ORIENTED_EDGE ( 'NONE', *, *, #6203, .T. ) ;
#27703=CARTESIAN_POINT ( 'NONE',  ( -0.3382184156749069581, -0.3855916753034488997, -1.550196850393700920 ) ) ;
#27718=CARTESIAN_POINT ( 'NONE',  ( -2.685748425196850164E-17, 0.000000000000000000, -1.934055118110236338 ) ) ;
#27724=CARTESIAN_POINT ( 'NONE',  ( -0.1078280746903979848, 0.3175540113612246862, 1.953740157480315043 ) ) ;
#27727=CARTESIAN_POINT ( 'NONE',  ( -0.5671862884095143498, 0.07472527936311554320, 0.9399606299212598381 ) ) ;
#27732=CARTESIAN_POINT ( 'NONE',  ( 0.1791085948259714400, 0.3102804211135531398, -3.115157480314960647 ) ) ;
#27738=CARTESIAN_POINT ( 'NONE',  ( -0.4669911931914537129, -0.1585706980422384171, -1.550196850393700920 ) ) ;
#27739=CARTESIAN_POINT ( 'NONE',  ( 0.2860009521618275818, -0.4954734376826439579, 0.9399606299212600602 ) ) ;
#27742=CARTESIAN_POINT ( 'NONE',  ( 0.2356229156554159598, -0.4776874499715153544, 1.747047244094488194 ) ) ;
#27745=CARTESIAN_POINT ( 'NONE',  ( -0.2938049579018679469, -0.3349573549949684259, -1.934055118110236338 ) ) ;
#27747=CARTESIAN_POINT ( 'NONE',  ( -0.09522017135408125665, 0.3002250880419695678, -3.246903465181130599 ) ) ;
#27755=CARTESIAN_POINT ( 'NONE',  ( -0.1275996891957738577, 0.4763861460130593972, -1.550196850393700920 ) ) ;
#27759=CARTESIAN_POINT ( 'NONE',  ( -0.4296318976989931815, -0.1458850421962362698, -1.934055118110236338 ) ) ;
#27764=CARTESIAN_POINT ( 'NONE',  ( 0.03478633594543814600, -0.5314960629921260393, 1.747047244094488194 ) ) ;
#27773=CARTESIAN_POINT ( 'NONE',  ( 0.2817310484609195642, 0.2161381151962948888, 1.953740157480315043 ) ) ;
#27776=CARTESIAN_POINT ( 'NONE',  ( 0.3772436174784425389, -0.4300830224589218265, 0.9399606299212598381 ) ) ;
#27777=CARTESIAN_POINT ( 'NONE',  ( 0.000000000000000000, 0.000000000000000000, 2.504921259842519898 ) ) ;
#27782=CARTESIAN_POINT ( 'NONE',  ( 0.09660931395005455113, -0.3606853515406215904, -3.115157480314960647 ) ) ;
#27789=AXIS2_PLACEMENT_3D ( 'NONE', #10100, #6296, #18709 ) ;
#27792=CARTESIAN_POINT ( 'NONE',  ( -0.4783323773986817851, 0.2762247810518556612, 0.9202755905511811330 ) ) ;
#27796=CARTESIAN_POINT ( 'NONE',  ( -0.2530785775239965951, 0.5130740159366039554, 0.9399606299212602822 ) ) ;
#27803=CARTESIAN_POINT ( 'NONE',  ( -0.4600326175560542907, 0.2268096725222489285, 1.766732283464566899 ) ) ;
#27806=CARTESIAN_POINT ( 'NONE',  ( -0.3726024258163779246, 0.02438677169354841121, -3.115157480314960647 ) ) ;
#27810=CARTESIAN_POINT ( 'NONE',  ( 0.2041304421298337501, 0.2660793235464286033, 1.973425196850393970 ) ) ;
#27814=CARTESIAN_POINT ( 'NONE',  ( 0.3707612262533033776, -0.3252100150720387273, -1.550196850393700920 ) ) ;
#27834=DIRECTION ( 'NONE',  ( -1.000000000000000000, 0.000000000000000000, -0.000000000000000000 ) ) ;
#27835=CARTESIAN_POINT ( 'NONE',  ( -0.09842519684999360974, 0.1968503937007873850, -3.259751644589251818 ) ) ;
#27847=ORIENTED_EDGE ( 'NONE', *, *, #14207, .F. ) ;
#27852=CARTESIAN_POINT ( 'NONE',  ( 0.09842519685039355370, 0.2165354330708661457, -3.548228346456693050 ) ) ;
#27865=CARTESIAN_POINT ( 'NONE',  ( -0.03607471876262473287, 0.5511811023622048555, 0.9399606299212598381 ) ) ;
#27870=CARTESIAN_POINT ( 'NONE',  ( -0.2181198385716950350, 0.2842139414039993039, -3.115157480314961091 ) ) ;
#27872=ADVANCED_FACE ( 'NONE', ( #8575 ), #17032, .T. ) ;
#27876=CARTESIAN_POINT ( 'NONE',  ( 0.5085118447796559416, -0.06699507805604926203, -1.550196850393700920 ) ) ;
#27877=CARTESIAN_POINT ( 'NONE',  ( 0.03746919241598507117, -0.5708675606921427281, 0.9399606299212600602 ) ) ;
#27879=DIRECTION ( 'NONE',  ( -0.7071067818211432821, 8.659560570126489743E-17, 0.7071067805519516414 ) ) ;
ENDSEC;
END-ISO-10303-21;
